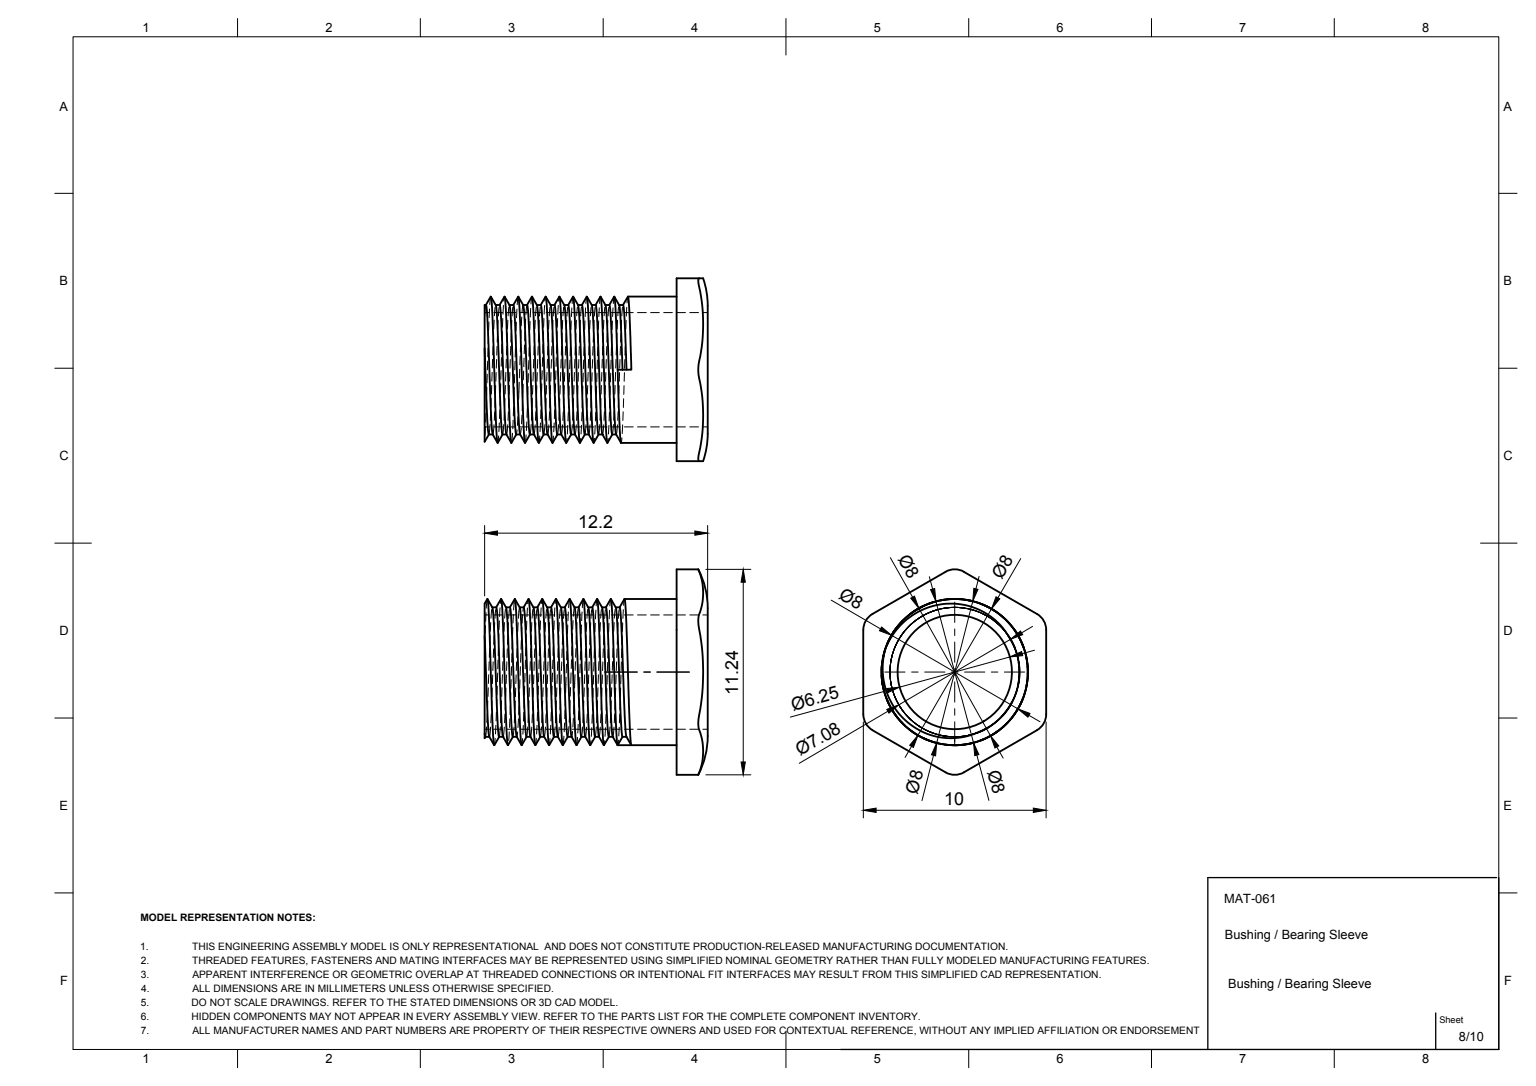
ISO-10303-21;
HEADER;
/* Generated by software containing ST-Developer
 * from STEP Tools, Inc. (www.steptools.com) 
 */

FILE_DESCRIPTION(
/* description */ ('', 'CAx-IF Rec.Pracs.---Representation and Presentation of Product Manufa
cturing Information (PMI)---4.0---2014-10-13'),
/* implementation_level */ '2;1');

FILE_NAME(
/* name */ 'Bushing _ Bearing Sleeve.step',
/* time_stamp */ '2026-10-28T14:45:12+01:00',
/* author */ (''),
/* organization */ (''),
/* preprocessor_version */ 'ST-DEVELOPER v20.2',
/* originating_system */ 'Autodesk Translation Framework v15.17.0.0',
/* authorisation */ '');

FILE_SCHEMA (('AP242_MANAGED_MODEL_BASED_3D_ENGINEERING_MIM_LF { 1 0 10303 442 2 1 4 }'));
ENDSEC;

DATA;
#10=MECHANICAL_DESIGN_GEOMETRIC_PRESENTATION_REPRESENTATION('',(#267),#52164);
#64=(
BOUNDED_CURVE()
B_SPLINE_CURVE(2,(#46348,#46349,#46350),.UNSPECIFIED.,.F.,.F.)
B_SPLINE_CURVE_WITH_KNOTS((3,3),(1.23956041519017,1.57079632679222),
 .UNSPECIFIED.)
CURVE()
GEOMETRIC_REPRESENTATION_ITEM()
RATIONAL_B_SPLINE_CURVE((0.987875274923375,0.980288238878012,1.))
REPRESENTATION_ITEM('')
);
#198=(
BOUNDED_SURFACE()
B_SPLINE_SURFACE(2,2,((#46210,#46211,#46212,#46213,#46214,#46215,#46216,
#46217,#46218),(#46219,#46220,#46221,#46222,#46223,#46224,#46225,#46226,
#46227),(#46228,#46229,#46230,#46231,#46232,#46233,#46234,#46235,#46236)),
 .UNSPECIFIED.,.F.,.T.,.F.)
B_SPLINE_SURFACE_WITH_KNOTS((3,3),(3,2,2,2,3),(-1.57079632679222,-1.09244241804695),
(-3.14159265358979,-1.5707963267949,0.,1.5707963267949,3.14159265358979),
 .UNSPECIFIED.)
GEOMETRIC_REPRESENTATION_ITEM()
RATIONAL_B_SPLINE_SURFACE(((1.,0.707106781186548,1.,0.707106781186548,1.,
0.707106781186548,1.,0.707106781186548,1.),(0.971533285943088,0.686977774638807,
0.971533285943088,0.686977774638807,0.971533285943088,0.686977774638807,
0.971533285943088,0.686977774638807,0.971533285943088),(1.,0.707106781186548,
1.,0.707106781186548,1.,0.707106781186548,1.,0.707106781186548,1.)))
REPRESENTATION_ITEM('')
SURFACE()
);
#241=SHAPE_REPRESENTATION_RELATIONSHIP('SRR','None',#52220,#254);
#254=ADVANCED_BREP_SHAPE_REPRESENTATION('',(#280),#52160);
#267=STYLED_ITEM('',(#52318),#280);
#280=MANIFOLD_SOLID_BREP('Body1',#9127);
#317=FACE_BOUND('',#1584,.T.);
#318=FACE_BOUND('',#1587,.T.);
#319=FACE_BOUND('',#1591,.T.);
#400=B_SPLINE_SURFACE_WITH_KNOTS('',3,3,((#46509,#46510,#46511,#46512,#46513,
#46514,#46515,#46516,#46517,#46518,#46519,#46520,#46521,#46522,#46523,#46524,
#46525,#46526,#46527,#46528,#46529,#46530,#46531,#46532,#46533,#46534,#46535,
#46536,#46537,#46538,#46539,#46540,#46541,#46542,#46543,#46544,#46545,#46546,
#46547,#46548,#46549,#46550,#46551,#46552,#46553,#46554,#46555,#46556,#46557,
#46558,#46559,#46560,#46561,#46562,#46563,#46564,#46565,#46566,#46567,#46568,
#46569,#46570,#46571,#46572,#46573,#46574,#46575),(#46576,#46577,#46578,
#46579,#46580,#46581,#46582,#46583,#46584,#46585,#46586,#46587,#46588,#46589,
#46590,#46591,#46592,#46593,#46594,#46595,#46596,#46597,#46598,#46599,#46600,
#46601,#46602,#46603,#46604,#46605,#46606,#46607,#46608,#46609,#46610,#46611,
#46612,#46613,#46614,#46615,#46616,#46617,#46618,#46619,#46620,#46621,#46622,
#46623,#46624,#46625,#46626,#46627,#46628,#46629,#46630,#46631,#46632,#46633,
#46634,#46635,#46636,#46637,#46638,#46639,#46640,#46641,#46642),(#46643,
#46644,#46645,#46646,#46647,#46648,#46649,#46650,#46651,#46652,#46653,#46654,
#46655,#46656,#46657,#46658,#46659,#46660,#46661,#46662,#46663,#46664,#46665,
#46666,#46667,#46668,#46669,#46670,#46671,#46672,#46673,#46674,#46675,#46676,
#46677,#46678,#46679,#46680,#46681,#46682,#46683,#46684,#46685,#46686,#46687,
#46688,#46689,#46690,#46691,#46692,#46693,#46694,#46695,#46696,#46697,#46698,
#46699,#46700,#46701,#46702,#46703,#46704,#46705,#46706,#46707,#46708,#46709),
(#46710,#46711,#46712,#46713,#46714,#46715,#46716,#46717,#46718,#46719,
#46720,#46721,#46722,#46723,#46724,#46725,#46726,#46727,#46728,#46729,#46730,
#46731,#46732,#46733,#46734,#46735,#46736,#46737,#46738,#46739,#46740,#46741,
#46742,#46743,#46744,#46745,#46746,#46747,#46748,#46749,#46750,#46751,#46752,
#46753,#46754,#46755,#46756,#46757,#46758,#46759,#46760,#46761,#46762,#46763,
#46764,#46765,#46766,#46767,#46768,#46769,#46770,#46771,#46772,#46773,#46774,
#46775,#46776)),.UNSPECIFIED.,.F.,.F.,.F.,(4,4),(4,1,1,1,1,1,1,1,1,1,1,
1,1,1,1,1,1,1,1,1,1,1,1,1,1,1,1,1,1,1,1,1,1,1,1,1,1,1,1,1,1,1,1,1,1,1,1,
1,1,1,1,1,1,1,1,1,1,1,1,1,1,1,1,1,4),(-0.04605142190376,1.046051421904),
(-0.02,-0.00375,0.0125,0.02875,0.045,0.06125,0.0775,0.09375,0.11,0.12625,
0.1425,0.15875,0.175,0.19125,0.2075,0.22375,0.24,0.25625,0.2725,0.28875,
0.305,0.32125,0.3375,0.35375,0.37,0.38625,0.4025,0.41875,0.435,0.45125,
0.4675,0.48375,0.5,0.51625,0.5325,0.54875,0.565,0.58125,0.5975,0.61375,
0.63,0.64625,0.6625,0.67875,0.695,0.71125,0.7275,0.74375,0.76,0.77625,0.7925,
0.80875,0.825,0.84125,0.8575,0.87375,0.89,0.90625,0.9225,0.93875,0.955,
0.97125,0.9875,1.00375,1.02),.UNSPECIFIED.);
#401=B_SPLINE_SURFACE_WITH_KNOTS('',3,3,((#47626,#47627,#47628,#47629,#47630,
#47631,#47632,#47633,#47634,#47635,#47636,#47637,#47638,#47639,#47640,#47641,
#47642,#47643,#47644,#47645,#47646,#47647,#47648,#47649,#47650,#47651,#47652,
#47653,#47654,#47655,#47656,#47657,#47658,#47659,#47660,#47661,#47662,#47663,
#47664,#47665,#47666,#47667,#47668,#47669,#47670,#47671,#47672,#47673,#47674,
#47675,#47676,#47677,#47678,#47679,#47680,#47681,#47682,#47683,#47684,#47685,
#47686,#47687,#47688,#47689,#47690,#47691,#47692),(#47693,#47694,#47695,
#47696,#47697,#47698,#47699,#47700,#47701,#47702,#47703,#47704,#47705,#47706,
#47707,#47708,#47709,#47710,#47711,#47712,#47713,#47714,#47715,#47716,#47717,
#47718,#47719,#47720,#47721,#47722,#47723,#47724,#47725,#47726,#47727,#47728,
#47729,#47730,#47731,#47732,#47733,#47734,#47735,#47736,#47737,#47738,#47739,
#47740,#47741,#47742,#47743,#47744,#47745,#47746,#47747,#47748,#47749,#47750,
#47751,#47752,#47753,#47754,#47755,#47756,#47757,#47758,#47759),(#47760,
#47761,#47762,#47763,#47764,#47765,#47766,#47767,#47768,#47769,#47770,#47771,
#47772,#47773,#47774,#47775,#47776,#47777,#47778,#47779,#47780,#47781,#47782,
#47783,#47784,#47785,#47786,#47787,#47788,#47789,#47790,#47791,#47792,#47793,
#47794,#47795,#47796,#47797,#47798,#47799,#47800,#47801,#47802,#47803,#47804,
#47805,#47806,#47807,#47808,#47809,#47810,#47811,#47812,#47813,#47814,#47815,
#47816,#47817,#47818,#47819,#47820,#47821,#47822,#47823,#47824,#47825,#47826),
(#47827,#47828,#47829,#47830,#47831,#47832,#47833,#47834,#47835,#47836,
#47837,#47838,#47839,#47840,#47841,#47842,#47843,#47844,#47845,#47846,#47847,
#47848,#47849,#47850,#47851,#47852,#47853,#47854,#47855,#47856,#47857,#47858,
#47859,#47860,#47861,#47862,#47863,#47864,#47865,#47866,#47867,#47868,#47869,
#47870,#47871,#47872,#47873,#47874,#47875,#47876,#47877,#47878,#47879,#47880,
#47881,#47882,#47883,#47884,#47885,#47886,#47887,#47888,#47889,#47890,#47891,
#47892,#47893)),.UNSPECIFIED.,.F.,.F.,.F.,(4,4),(4,1,1,1,1,1,1,1,1,1,1,
1,1,1,1,1,1,1,1,1,1,1,1,1,1,1,1,1,1,1,1,1,1,1,1,1,1,1,1,1,1,1,1,1,1,1,1,
1,1,1,1,1,1,1,1,1,1,1,1,1,1,1,1,1,4),(-0.04605142190375,1.046051421904),
(-0.02,-0.00375,0.0125,0.02875,0.045,0.06125,0.0775,0.09375,0.11,0.12625,
0.1425,0.15875,0.175,0.19125,0.2075,0.22375,0.24,0.25625,0.2725,0.28875,
0.305,0.32125,0.3375,0.35375,0.37,0.38625,0.4025,0.41875,0.435,0.45125,
0.4675,0.48375,0.5,0.51625,0.5325,0.54875,0.565,0.58125,0.5975,0.61375,
0.63,0.64625,0.6625,0.67875,0.695,0.71125,0.7275,0.74375,0.76,0.77625,0.7925,
0.80875,0.825,0.84125,0.8575,0.87375,0.89,0.90625,0.9225,0.93875,0.955,
0.97125,0.9875,1.00375,1.02),.UNSPECIFIED.);
#402=B_SPLINE_SURFACE_WITH_KNOTS('',3,3,((#48678,#48679,#48680,#48681,#48682,
#48683,#48684,#48685,#48686,#48687,#48688,#48689,#48690,#48691,#48692,#48693,
#48694,#48695,#48696,#48697,#48698,#48699,#48700,#48701,#48702,#48703,#48704,
#48705,#48706,#48707,#48708,#48709,#48710,#48711,#48712,#48713,#48714,#48715,
#48716,#48717,#48718,#48719,#48720,#48721,#48722,#48723,#48724,#48725,#48726,
#48727,#48728,#48729,#48730,#48731,#48732,#48733,#48734,#48735,#48736,#48737,
#48738,#48739,#48740,#48741,#48742,#48743,#48744),(#48745,#48746,#48747,
#48748,#48749,#48750,#48751,#48752,#48753,#48754,#48755,#48756,#48757,#48758,
#48759,#48760,#48761,#48762,#48763,#48764,#48765,#48766,#48767,#48768,#48769,
#48770,#48771,#48772,#48773,#48774,#48775,#48776,#48777,#48778,#48779,#48780,
#48781,#48782,#48783,#48784,#48785,#48786,#48787,#48788,#48789,#48790,#48791,
#48792,#48793,#48794,#48795,#48796,#48797,#48798,#48799,#48800,#48801,#48802,
#48803,#48804,#48805,#48806,#48807,#48808,#48809,#48810,#48811),(#48812,
#48813,#48814,#48815,#48816,#48817,#48818,#48819,#48820,#48821,#48822,#48823,
#48824,#48825,#48826,#48827,#48828,#48829,#48830,#48831,#48832,#48833,#48834,
#48835,#48836,#48837,#48838,#48839,#48840,#48841,#48842,#48843,#48844,#48845,
#48846,#48847,#48848,#48849,#48850,#48851,#48852,#48853,#48854,#48855,#48856,
#48857,#48858,#48859,#48860,#48861,#48862,#48863,#48864,#48865,#48866,#48867,
#48868,#48869,#48870,#48871,#48872,#48873,#48874,#48875,#48876,#48877,#48878),
(#48879,#48880,#48881,#48882,#48883,#48884,#48885,#48886,#48887,#48888,
#48889,#48890,#48891,#48892,#48893,#48894,#48895,#48896,#48897,#48898,#48899,
#48900,#48901,#48902,#48903,#48904,#48905,#48906,#48907,#48908,#48909,#48910,
#48911,#48912,#48913,#48914,#48915,#48916,#48917,#48918,#48919,#48920,#48921,
#48922,#48923,#48924,#48925,#48926,#48927,#48928,#48929,#48930,#48931,#48932,
#48933,#48934,#48935,#48936,#48937,#48938,#48939,#48940,#48941,#48942,#48943,
#48944,#48945)),.UNSPECIFIED.,.F.,.F.,.F.,(4,4),(4,1,1,1,1,1,1,1,1,1,1,
1,1,1,1,1,1,1,1,1,1,1,1,1,1,1,1,1,1,1,1,1,1,1,1,1,1,1,1,1,1,1,1,1,1,1,1,
1,1,1,1,1,1,1,1,1,1,1,1,1,1,1,1,1,4),(-0.04605142190375,1.046051421904),
(-0.02,-0.00375,0.0125,0.02875,0.045,0.06125,0.0775,0.09375,0.11,0.12625,
0.1425,0.15875,0.175,0.19125,0.2075,0.22375,0.24,0.25625,0.2725,0.28875,
0.305,0.32125,0.3375,0.35375,0.37,0.38625,0.4025,0.41875,0.435,0.45125,
0.4675,0.48375,0.5,0.51625,0.5325,0.54875,0.565,0.58125,0.5975,0.61375,
0.63,0.64625,0.6625,0.67875,0.695,0.71125,0.7275,0.74375,0.76,0.77625,0.7925,
0.80875,0.825,0.84125,0.8575,0.87375,0.89,0.90625,0.9225,0.93875,0.955,
0.97125,0.9875,1.00375,1.02),.UNSPECIFIED.);
#403=B_SPLINE_SURFACE_WITH_KNOTS('',3,3,((#49626,#49627,#49628,#49629,#49630,
#49631,#49632,#49633,#49634,#49635,#49636,#49637,#49638,#49639,#49640,#49641,
#49642,#49643,#49644,#49645,#49646,#49647,#49648,#49649,#49650,#49651,#49652,
#49653,#49654,#49655,#49656,#49657,#49658,#49659,#49660,#49661,#49662,#49663,
#49664,#49665,#49666,#49667,#49668,#49669,#49670,#49671,#49672,#49673,#49674,
#49675,#49676,#49677,#49678,#49679,#49680,#49681,#49682,#49683,#49684,#49685,
#49686,#49687,#49688,#49689,#49690,#49691,#49692),(#49693,#49694,#49695,
#49696,#49697,#49698,#49699,#49700,#49701,#49702,#49703,#49704,#49705,#49706,
#49707,#49708,#49709,#49710,#49711,#49712,#49713,#49714,#49715,#49716,#49717,
#49718,#49719,#49720,#49721,#49722,#49723,#49724,#49725,#49726,#49727,#49728,
#49729,#49730,#49731,#49732,#49733,#49734,#49735,#49736,#49737,#49738,#49739,
#49740,#49741,#49742,#49743,#49744,#49745,#49746,#49747,#49748,#49749,#49750,
#49751,#49752,#49753,#49754,#49755,#49756,#49757,#49758,#49759),(#49760,
#49761,#49762,#49763,#49764,#49765,#49766,#49767,#49768,#49769,#49770,#49771,
#49772,#49773,#49774,#49775,#49776,#49777,#49778,#49779,#49780,#49781,#49782,
#49783,#49784,#49785,#49786,#49787,#49788,#49789,#49790,#49791,#49792,#49793,
#49794,#49795,#49796,#49797,#49798,#49799,#49800,#49801,#49802,#49803,#49804,
#49805,#49806,#49807,#49808,#49809,#49810,#49811,#49812,#49813,#49814,#49815,
#49816,#49817,#49818,#49819,#49820,#49821,#49822,#49823,#49824,#49825,#49826),
(#49827,#49828,#49829,#49830,#49831,#49832,#49833,#49834,#49835,#49836,
#49837,#49838,#49839,#49840,#49841,#49842,#49843,#49844,#49845,#49846,#49847,
#49848,#49849,#49850,#49851,#49852,#49853,#49854,#49855,#49856,#49857,#49858,
#49859,#49860,#49861,#49862,#49863,#49864,#49865,#49866,#49867,#49868,#49869,
#49870,#49871,#49872,#49873,#49874,#49875,#49876,#49877,#49878,#49879,#49880,
#49881,#49882,#49883,#49884,#49885,#49886,#49887,#49888,#49889,#49890,#49891,
#49892,#49893)),.UNSPECIFIED.,.F.,.F.,.F.,(4,4),(4,1,1,1,1,1,1,1,1,1,1,
1,1,1,1,1,1,1,1,1,1,1,1,1,1,1,1,1,1,1,1,1,1,1,1,1,1,1,1,1,1,1,1,1,1,1,1,
1,1,1,1,1,1,1,1,1,1,1,1,1,1,1,1,1,4),(-0.04605142190375,1.046051421904),
(0.151,0.1645257352941,0.1780514705882,0.1915772058824,0.2051029411765,
0.2186286764706,0.2321544117647,0.2456801470588,0.2592058823529,0.2727316176471,
0.2862573529412,0.2997830882353,0.3133088235294,0.3268345588235,0.3403602941176,
0.3538860294118,0.3674117647059,0.3809375,0.3944632352941,0.4079889705882,
0.4215147058824,0.4350404411765,0.4485661764706,0.4620919117647,0.4756176470588,
0.4891433823529,0.5026691176471,0.5161948529412,0.5297205882353,0.5432463235294,
0.5567720588235,0.5702977941176,0.5838235294118,0.5973492647059,0.610875,
0.6244007352941,0.6379264705882,0.6514522058824,0.6649779411765,0.6785036764706,
0.6920294117647,0.7055551470588,0.7190808823529,0.7326066176471,0.7461323529412,
0.7596580882353,0.7731838235294,0.7867095588235,0.8002352941176,0.8137610294118,
0.8272867647059,0.8408125,0.8543382352941,0.8678639705882,0.8813897058824,
0.8949154411765,0.9084411764706,0.9219669117647,0.9354926470588,0.9490183823529,
0.9625441176471,0.9760698529412,0.9895955882353,1.003121323529,1.016647058824),
 .UNSPECIFIED.);
#404=B_SPLINE_SURFACE_WITH_KNOTS('',3,3,((#50188,#50189,#50190,#50191,#50192,
#50193,#50194,#50195,#50196,#50197,#50198,#50199,#50200,#50201,#50202,#50203,
#50204,#50205,#50206,#50207,#50208,#50209,#50210,#50211,#50212,#50213,#50214,
#50215,#50216,#50217,#50218,#50219,#50220,#50221,#50222),(#50223,#50224,
#50225,#50226,#50227,#50228,#50229,#50230,#50231,#50232,#50233,#50234,#50235,
#50236,#50237,#50238,#50239,#50240,#50241,#50242,#50243,#50244,#50245,#50246,
#50247,#50248,#50249,#50250,#50251,#50252,#50253,#50254,#50255,#50256,#50257),
(#50258,#50259,#50260,#50261,#50262,#50263,#50264,#50265,#50266,#50267,
#50268,#50269,#50270,#50271,#50272,#50273,#50274,#50275,#50276,#50277,#50278,
#50279,#50280,#50281,#50282,#50283,#50284,#50285,#50286,#50287,#50288,#50289,
#50290,#50291,#50292),(#50293,#50294,#50295,#50296,#50297,#50298,#50299,
#50300,#50301,#50302,#50303,#50304,#50305,#50306,#50307,#50308,#50309,#50310,
#50311,#50312,#50313,#50314,#50315,#50316,#50317,#50318,#50319,#50320,#50321,
#50322,#50323,#50324,#50325,#50326,#50327)),.UNSPECIFIED.,.F.,.F.,.F.,(4,
4),(4,1,1,1,1,1,1,1,1,1,1,1,1,1,1,1,1,1,1,1,1,1,1,1,1,1,1,1,1,1,1,1,4),
(-0.04605142190375,1.046051421904),(0.3253907954222,0.3468856965485,0.3683805976747,
0.389875498801,0.4113703999272,0.4328653010535,0.4543602021797,0.475855103306,
0.4973500044322,0.5188449055585,0.5403398066847,0.561834707811,0.5833296089372,
0.6048245100635,0.6263194111897,0.647814312316,0.6693092134423,0.6908041145685,
0.7122990156948,0.733793916821,0.7552888179473,0.7767837190735,0.7982786201998,
0.819773521326,0.8412684224523,0.8627633235785,0.8842582247048,0.905753125831,
0.9272480269573,0.9487429280835,0.9702378292098,0.9917327303361,1.013227631462),
 .UNSPECIFIED.);
#405=B_SPLINE_SURFACE_WITH_KNOTS('',3,3,((#50500,#50501,#50502,#50503,#50504,
#50505,#50506,#50507,#50508,#50509,#50510,#50511,#50512,#50513,#50514,#50515,
#50516,#50517,#50518,#50519,#50520,#50521,#50522,#50523,#50524,#50525,#50526,
#50527,#50528,#50529,#50530,#50531,#50532,#50533,#50534),(#50535,#50536,
#50537,#50538,#50539,#50540,#50541,#50542,#50543,#50544,#50545,#50546,#50547,
#50548,#50549,#50550,#50551,#50552,#50553,#50554,#50555,#50556,#50557,#50558,
#50559,#50560,#50561,#50562,#50563,#50564,#50565,#50566,#50567,#50568,#50569),
(#50570,#50571,#50572,#50573,#50574,#50575,#50576,#50577,#50578,#50579,
#50580,#50581,#50582,#50583,#50584,#50585,#50586,#50587,#50588,#50589,#50590,
#50591,#50592,#50593,#50594,#50595,#50596,#50597,#50598,#50599,#50600,#50601,
#50602,#50603,#50604),(#50605,#50606,#50607,#50608,#50609,#50610,#50611,
#50612,#50613,#50614,#50615,#50616,#50617,#50618,#50619,#50620,#50621,#50622,
#50623,#50624,#50625,#50626,#50627,#50628,#50629,#50630,#50631,#50632,#50633,
#50634,#50635,#50636,#50637,#50638,#50639)),.UNSPECIFIED.,.F.,.F.,.F.,(4,
4),(4,1,1,1,1,1,1,1,1,1,1,1,1,1,1,1,1,1,1,1,1,1,1,1,1,1,1,1,1,1,1,1,4),
(-0.1117758545036,1.111775854504),(0.2466092045778,0.2706143034515,0.2946194023253,
0.318624501199,0.3426296000728,0.3666346989465,0.3906397978203,0.414644896694,
0.4386499955678,0.4626550944415,0.4866601933153,0.510665292189,0.5346703910628,
0.5586754899365,0.5826805888103,0.606685687684,0.6306907865577,0.6546958854315,
0.6787009843052,0.702706083179,0.7267111820527,0.7507162809265,0.7747213798002,
0.798726478674,0.8227315775477,0.8467366764215,0.8707417752952,0.894746874169,
0.9187519730427,0.9427570719165,0.9667621707902,0.9907672696639,1.014772368538),
 .UNSPECIFIED.);
#406=B_SPLINE_SURFACE_WITH_KNOTS('',3,3,((#50641,#50642,#50643,#50644,#50645,
#50646,#50647,#50648,#50649,#50650,#50651,#50652,#50653,#50654,#50655,#50656,
#50657,#50658,#50659,#50660,#50661,#50662,#50663,#50664,#50665,#50666,#50667,
#50668,#50669,#50670,#50671,#50672,#50673,#50674,#50675,#50676,#50677,#50678,
#50679,#50680,#50681,#50682,#50683,#50684,#50685,#50686,#50687,#50688,#50689,
#50690,#50691,#50692,#50693,#50694,#50695,#50696,#50697,#50698,#50699,#50700,
#50701,#50702,#50703,#50704,#50705,#50706,#50707),(#50708,#50709,#50710,
#50711,#50712,#50713,#50714,#50715,#50716,#50717,#50718,#50719,#50720,#50721,
#50722,#50723,#50724,#50725,#50726,#50727,#50728,#50729,#50730,#50731,#50732,
#50733,#50734,#50735,#50736,#50737,#50738,#50739,#50740,#50741,#50742,#50743,
#50744,#50745,#50746,#50747,#50748,#50749,#50750,#50751,#50752,#50753,#50754,
#50755,#50756,#50757,#50758,#50759,#50760,#50761,#50762,#50763,#50764,#50765,
#50766,#50767,#50768,#50769,#50770,#50771,#50772,#50773,#50774),(#50775,
#50776,#50777,#50778,#50779,#50780,#50781,#50782,#50783,#50784,#50785,#50786,
#50787,#50788,#50789,#50790,#50791,#50792,#50793,#50794,#50795,#50796,#50797,
#50798,#50799,#50800,#50801,#50802,#50803,#50804,#50805,#50806,#50807,#50808,
#50809,#50810,#50811,#50812,#50813,#50814,#50815,#50816,#50817,#50818,#50819,
#50820,#50821,#50822,#50823,#50824,#50825,#50826,#50827,#50828,#50829,#50830,
#50831,#50832,#50833,#50834,#50835,#50836,#50837,#50838,#50839,#50840,#50841),
(#50842,#50843,#50844,#50845,#50846,#50847,#50848,#50849,#50850,#50851,
#50852,#50853,#50854,#50855,#50856,#50857,#50858,#50859,#50860,#50861,#50862,
#50863,#50864,#50865,#50866,#50867,#50868,#50869,#50870,#50871,#50872,#50873,
#50874,#50875,#50876,#50877,#50878,#50879,#50880,#50881,#50882,#50883,#50884,
#50885,#50886,#50887,#50888,#50889,#50890,#50891,#50892,#50893,#50894,#50895,
#50896,#50897,#50898,#50899,#50900,#50901,#50902,#50903,#50904,#50905,#50906,
#50907,#50908)),.UNSPECIFIED.,.F.,.F.,.F.,(4,4),(4,1,1,1,1,1,1,1,1,1,1,
1,1,1,1,1,1,1,1,1,1,1,1,1,1,1,1,1,1,1,1,1,1,1,1,1,1,1,1,1,1,1,1,1,1,1,1,
1,1,1,1,1,1,1,1,1,1,1,1,1,1,1,1,1,4),(-0.1117758545036,1.111775854504),
(-0.02,-0.00375,0.0125,0.02875,0.045,0.06125,0.0775,0.09375,0.11,0.12625,
0.1425,0.15875,0.175,0.19125,0.2075,0.22375,0.24,0.25625,0.2725,0.28875,
0.305,0.32125,0.3375,0.35375,0.37,0.38625,0.4025,0.41875,0.435,0.45125,
0.4675,0.48375,0.5,0.51625,0.5325,0.54875,0.565,0.58125,0.5975,0.61375,
0.63,0.64625,0.6625,0.67875,0.695,0.71125,0.7275,0.74375,0.76,0.77625,0.7925,
0.80875,0.825,0.84125,0.8575,0.87375,0.89,0.90625,0.9225,0.93875,0.955,
0.97125,0.9875,1.00375,1.02),.UNSPECIFIED.);
#407=B_SPLINE_SURFACE_WITH_KNOTS('',3,3,((#50910,#50911,#50912,#50913,#50914,
#50915,#50916,#50917,#50918,#50919,#50920,#50921,#50922,#50923,#50924,#50925,
#50926,#50927,#50928,#50929,#50930,#50931,#50932,#50933,#50934,#50935,#50936,
#50937,#50938,#50939,#50940,#50941,#50942,#50943,#50944,#50945,#50946,#50947,
#50948,#50949,#50950,#50951,#50952,#50953,#50954,#50955,#50956,#50957,#50958,
#50959,#50960,#50961,#50962,#50963,#50964,#50965,#50966,#50967,#50968,#50969,
#50970,#50971,#50972,#50973,#50974,#50975,#50976),(#50977,#50978,#50979,
#50980,#50981,#50982,#50983,#50984,#50985,#50986,#50987,#50988,#50989,#50990,
#50991,#50992,#50993,#50994,#50995,#50996,#50997,#50998,#50999,#51000,#51001,
#51002,#51003,#51004,#51005,#51006,#51007,#51008,#51009,#51010,#51011,#51012,
#51013,#51014,#51015,#51016,#51017,#51018,#51019,#51020,#51021,#51022,#51023,
#51024,#51025,#51026,#51027,#51028,#51029,#51030,#51031,#51032,#51033,#51034,
#51035,#51036,#51037,#51038,#51039,#51040,#51041,#51042,#51043),(#51044,
#51045,#51046,#51047,#51048,#51049,#51050,#51051,#51052,#51053,#51054,#51055,
#51056,#51057,#51058,#51059,#51060,#51061,#51062,#51063,#51064,#51065,#51066,
#51067,#51068,#51069,#51070,#51071,#51072,#51073,#51074,#51075,#51076,#51077,
#51078,#51079,#51080,#51081,#51082,#51083,#51084,#51085,#51086,#51087,#51088,
#51089,#51090,#51091,#51092,#51093,#51094,#51095,#51096,#51097,#51098,#51099,
#51100,#51101,#51102,#51103,#51104,#51105,#51106,#51107,#51108,#51109,#51110),
(#51111,#51112,#51113,#51114,#51115,#51116,#51117,#51118,#51119,#51120,
#51121,#51122,#51123,#51124,#51125,#51126,#51127,#51128,#51129,#51130,#51131,
#51132,#51133,#51134,#51135,#51136,#51137,#51138,#51139,#51140,#51141,#51142,
#51143,#51144,#51145,#51146,#51147,#51148,#51149,#51150,#51151,#51152,#51153,
#51154,#51155,#51156,#51157,#51158,#51159,#51160,#51161,#51162,#51163,#51164,
#51165,#51166,#51167,#51168,#51169,#51170,#51171,#51172,#51173,#51174,#51175,
#51176,#51177)),.UNSPECIFIED.,.F.,.F.,.F.,(4,4),(4,1,1,1,1,1,1,1,1,1,1,
1,1,1,1,1,1,1,1,1,1,1,1,1,1,1,1,1,1,1,1,1,1,1,1,1,1,1,1,1,1,1,1,1,1,1,1,
1,1,1,1,1,1,1,1,1,1,1,1,1,1,1,1,1,4),(-0.1117758545037,1.111775854504),
(-0.02,-0.00375,0.0125,0.02875,0.045,0.06125,0.0775,0.09375,0.11,0.12625,
0.1425,0.15875,0.175,0.19125,0.2075,0.22375,0.24,0.25625,0.2725,0.28875,
0.305,0.32125,0.3375,0.35375,0.37,0.38625,0.4025,0.41875,0.435,0.45125,
0.4675,0.48375,0.5,0.51625,0.5325,0.54875,0.565,0.58125,0.5975,0.61375,
0.63,0.64625,0.6625,0.67875,0.695,0.71125,0.7275,0.74375,0.76,0.77625,0.7925,
0.80875,0.825,0.84125,0.8575,0.87375,0.89,0.90625,0.9225,0.93875,0.955,
0.97125,0.9875,1.00375,1.02),.UNSPECIFIED.);
#408=B_SPLINE_SURFACE_WITH_KNOTS('',3,3,((#51791,#51792,#51793,#51794,#51795,
#51796,#51797,#51798,#51799,#51800,#51801,#51802,#51803,#51804,#51805,#51806,
#51807,#51808,#51809,#51810,#51811,#51812,#51813,#51814,#51815,#51816,#51817,
#51818,#51819,#51820,#51821,#51822,#51823,#51824,#51825,#51826,#51827,#51828,
#51829,#51830,#51831,#51832,#51833,#51834,#51835,#51836,#51837,#51838,#51839,
#51840,#51841,#51842,#51843,#51844,#51845,#51846,#51847,#51848,#51849,#51850,
#51851,#51852,#51853,#51854,#51855,#51856,#51857),(#51858,#51859,#51860,
#51861,#51862,#51863,#51864,#51865,#51866,#51867,#51868,#51869,#51870,#51871,
#51872,#51873,#51874,#51875,#51876,#51877,#51878,#51879,#51880,#51881,#51882,
#51883,#51884,#51885,#51886,#51887,#51888,#51889,#51890,#51891,#51892,#51893,
#51894,#51895,#51896,#51897,#51898,#51899,#51900,#51901,#51902,#51903,#51904,
#51905,#51906,#51907,#51908,#51909,#51910,#51911,#51912,#51913,#51914,#51915,
#51916,#51917,#51918,#51919,#51920,#51921,#51922,#51923,#51924),(#51925,
#51926,#51927,#51928,#51929,#51930,#51931,#51932,#51933,#51934,#51935,#51936,
#51937,#51938,#51939,#51940,#51941,#51942,#51943,#51944,#51945,#51946,#51947,
#51948,#51949,#51950,#51951,#51952,#51953,#51954,#51955,#51956,#51957,#51958,
#51959,#51960,#51961,#51962,#51963,#51964,#51965,#51966,#51967,#51968,#51969,
#51970,#51971,#51972,#51973,#51974,#51975,#51976,#51977,#51978,#51979,#51980,
#51981,#51982,#51983,#51984,#51985,#51986,#51987,#51988,#51989,#51990,#51991),
(#51992,#51993,#51994,#51995,#51996,#51997,#51998,#51999,#52000,#52001,
#52002,#52003,#52004,#52005,#52006,#52007,#52008,#52009,#52010,#52011,#52012,
#52013,#52014,#52015,#52016,#52017,#52018,#52019,#52020,#52021,#52022,#52023,
#52024,#52025,#52026,#52027,#52028,#52029,#52030,#52031,#52032,#52033,#52034,
#52035,#52036,#52037,#52038,#52039,#52040,#52041,#52042,#52043,#52044,#52045,
#52046,#52047,#52048,#52049,#52050,#52051,#52052,#52053,#52054,#52055,#52056,
#52057,#52058)),.UNSPECIFIED.,.F.,.F.,.F.,(4,4),(4,1,1,1,1,1,1,1,1,1,1,
1,1,1,1,1,1,1,1,1,1,1,1,1,1,1,1,1,1,1,1,1,1,1,1,1,1,1,1,1,1,1,1,1,1,1,1,
1,1,1,1,1,1,1,1,1,1,1,1,1,1,1,1,1,4),(-0.04605142190376,1.046051421904),
(-0.02,-0.00375,0.0125,0.02875,0.045,0.06125,0.0775,0.09375,0.11,0.12625,
0.1425,0.15875,0.175,0.19125,0.2075,0.22375,0.24,0.25625,0.2725,0.28875,
0.305,0.32125,0.3375,0.35375,0.37,0.38625,0.4025,0.41875,0.435,0.45125,
0.4675,0.48375,0.5,0.51625,0.5325,0.54875,0.565,0.58125,0.5975,0.61375,
0.63,0.64625,0.6625,0.67875,0.695,0.71125,0.7275,0.74375,0.76,0.77625,0.7925,
0.80875,0.825,0.84125,0.8575,0.87375,0.89,0.90625,0.9225,0.93875,0.955,
0.97125,0.9875,1.00375,1.02),.UNSPECIFIED.);
#505=PLANE('',#10143);
#506=PLANE('',#10147);
#507=PLANE('',#10151);
#508=PLANE('',#10159);
#509=PLANE('',#10160);
#510=PLANE('',#10162);
#511=PLANE('',#10164);
#512=PLANE('',#10166);
#513=PLANE('',#10168);
#514=PLANE('',#10170);
#1017=FACE_OUTER_BOUND('',#1583,.T.);
#1018=FACE_OUTER_BOUND('',#1585,.T.);
#1019=FACE_OUTER_BOUND('',#1586,.T.);
#1020=FACE_OUTER_BOUND('',#1588,.T.);
#1021=FACE_OUTER_BOUND('',#1589,.T.);
#1022=FACE_OUTER_BOUND('',#1590,.T.);
#1023=FACE_OUTER_BOUND('',#1592,.T.);
#1024=FACE_OUTER_BOUND('',#1593,.T.);
#1025=FACE_OUTER_BOUND('',#1594,.T.);
#1026=FACE_OUTER_BOUND('',#1595,.T.);
#1027=FACE_OUTER_BOUND('',#1596,.T.);
#1028=FACE_OUTER_BOUND('',#1597,.T.);
#1029=FACE_OUTER_BOUND('',#1598,.T.);
#1030=FACE_OUTER_BOUND('',#1599,.T.);
#1031=FACE_OUTER_BOUND('',#1600,.T.);
#1032=FACE_OUTER_BOUND('',#1601,.T.);
#1033=FACE_OUTER_BOUND('',#1602,.T.);
#1034=FACE_OUTER_BOUND('',#1603,.T.);
#1035=FACE_OUTER_BOUND('',#1604,.T.);
#1036=FACE_OUTER_BOUND('',#1605,.T.);
#1037=FACE_OUTER_BOUND('',#1606,.T.);
#1038=FACE_OUTER_BOUND('',#1607,.T.);
#1039=FACE_OUTER_BOUND('',#1608,.T.);
#1040=FACE_OUTER_BOUND('',#1609,.T.);
#1041=FACE_OUTER_BOUND('',#1610,.T.);
#1042=FACE_OUTER_BOUND('',#1611,.T.);
#1043=FACE_OUTER_BOUND('',#1612,.T.);
#1044=FACE_OUTER_BOUND('',#1613,.T.);
#1583=EDGE_LOOP('',(#8170,#8171,#8172,#8173,#8174));
#1584=EDGE_LOOP('',(#8175));
#1585=EDGE_LOOP('',(#8176,#8177,#8178,#8179));
#1586=EDGE_LOOP('',(#8180));
#1587=EDGE_LOOP('',(#8181));
#1588=EDGE_LOOP('',(#8182,#8183,#8184,#8185,#8186,#8187,#8188,#8189,#8190,
#8191,#8192,#8193,#8194,#8195,#8196,#8197));
#1589=EDGE_LOOP('',(#8198,#8199,#8200,#8201));
#1590=EDGE_LOOP('',(#8202,#8203,#8204,#8205,#8206,#8207,#8208,#8209,#8210,
#8211,#8212,#8213));
#1591=EDGE_LOOP('',(#8214));
#1592=EDGE_LOOP('',(#8215,#8216,#8217,#8218,#8219,#8220));
#1593=EDGE_LOOP('',(#8221,#8222,#8223,#8224));
#1594=EDGE_LOOP('',(#8225,#8226,#8227,#8228,#8229));
#1595=EDGE_LOOP('',(#8230,#8231,#8232,#8233,#8234));
#1596=EDGE_LOOP('',(#8235,#8236,#8237,#8238,#8239));
#1597=EDGE_LOOP('',(#8240,#8241,#8242,#8243,#8244,#8245));
#1598=EDGE_LOOP('',(#8246,#8247,#8248,#8249));
#1599=EDGE_LOOP('',(#8250,#8251,#8252,#8253,#8254));
#1600=EDGE_LOOP('',(#8255,#8256,#8257,#8258));
#1601=EDGE_LOOP('',(#8259,#8260,#8261,#8262));
#1602=EDGE_LOOP('',(#8263,#8264,#8265,#8266,#8267,#8268));
#1603=EDGE_LOOP('',(#8269,#8270,#8271,#8272));
#1604=EDGE_LOOP('',(#8273,#8274,#8275,#8276));
#1605=EDGE_LOOP('',(#8277,#8278,#8279,#8280));
#1606=EDGE_LOOP('',(#8281,#8282,#8283,#8284));
#1607=EDGE_LOOP('',(#8285,#8286,#8287,#8288));
#1608=EDGE_LOOP('',(#8289,#8290,#8291,#8292));
#1609=EDGE_LOOP('',(#8293,#8294,#8295,#8296));
#1610=EDGE_LOOP('',(#8297,#8298,#8299,#8300));
#1611=EDGE_LOOP('',(#8301,#8302,#8303,#8304,#8305));
#1612=EDGE_LOOP('',(#8306,#8307,#8308,#8309));
#1613=EDGE_LOOP('',(#8310,#8311,#8312,#8313));
#2071=CIRCLE('',#10144,3.125);
#2072=CIRCLE('',#10146,3.125);
#2073=CIRCLE('',#10148,3.5);
#2074=CIRCLE('',#10150,1.);
#2075=CIRCLE('',#10152,1.);
#2076=CIRCLE('',#10153,1.);
#2077=CIRCLE('',#10154,1.);
#2078=CIRCLE('',#10155,1.);
#2079=CIRCLE('',#10156,1.);
#2080=CIRCLE('',#10157,4.);
#2428=B_SPLINE_CURVE_WITH_KNOTS('',3,(#46066,#46067,#46068,#46069),
 .UNSPECIFIED.,.F.,.F.,(4,4),(-0.000287379327346715,0.),.UNSPECIFIED.);
#2429=B_SPLINE_CURVE_WITH_KNOTS('',3,(#46071,#46072,#46073,#46074,#46075,
#46076,#46077,#46078,#46079,#46080,#46081,#46082,#46083,#46084,#46085,#46086,
#46087,#46088,#46089,#46090,#46091,#46092,#46093,#46094,#46095,#46096,#46097,
#46098,#46099,#46100,#46101,#46102,#46103,#46104,#46105,#46106,#46107,#46108,
#46109,#46110,#46111,#46112,#46113,#46114,#46115,#46116,#46117,#46118,#46119,
#46120,#46121,#46122,#46123,#46124,#46125,#46126,#46127,#46128,#46129,#46130,
#46131,#46132,#46133,#46134,#46135,#46136,#46137,#46138,#46139,#46140,#46141,
#46142,#46143,#46144,#46145,#46146,#46147,#46148,#46149,#46150,#46151,#46152,
#46153,#46154,#46155,#46156,#46157,#46158,#46159,#46160,#46161,#46162,#46163,
#46164),.UNSPECIFIED.,.F.,.F.,(4,3,3,3,3,3,3,3,3,3,3,3,3,3,3,3,3,3,3,3,
3,3,3,3,3,3,3,3,3,3,3,4),(0.,0.0334880516165954,0.0622449481709034,0.0833304545710313,
0.123139222900696,0.158240223188287,0.176189139696093,0.217007009430374,
0.243869787273509,0.26354322405106,0.302458774449498,0.33355876922255,0.374434885871789,
0.405321381393714,0.426172721464637,0.480843228725633,0.507476669962832,
0.544616299200151,0.574867627238567,0.592227140301538,0.637891373171595,
0.668397489031486,0.7156914768719,0.744145082796372,0.770511427895059,0.813365315244751,
0.836703116619631,0.881940300050722,0.91091246542526,0.927753817005376,
0.962791389277124,0.997828961548873),.UNSPECIFIED.);
#2430=B_SPLINE_CURVE_WITH_KNOTS('',3,(#46166,#46167,#46168,#46169),
 .UNSPECIFIED.,.F.,.F.,(4,4),(-0.00107348259049816,0.),.UNSPECIFIED.);
#2431=B_SPLINE_CURVE_WITH_KNOTS('',3,(#46171,#46172,#46173,#46174,#46175,
#46176,#46177,#46178,#46179,#46180,#46181,#46182,#46183,#46184),
 .UNSPECIFIED.,.F.,.F.,(4,2,2,2,2,2,4),(-0.747237513889951,-0.627110670602595,
-0.492162734458781,-0.361378717436516,-0.240449917906045,-0.127292557609884,
-2.3301729044132E-6),.UNSPECIFIED.);
#2432=B_SPLINE_CURVE_WITH_KNOTS('',3,(#46185,#46186,#46187,#46188,#46189,
#46190,#46191,#46192,#46193,#46194,#46195,#46196,#46197,#46198,#46199,#46200),
 .UNSPECIFIED.,.F.,.F.,(4,2,2,2,2,2,2,4),(-0.557266864962719,-0.476580853062999,
-0.396866002960756,-0.315372123091983,-0.242726490281515,-0.148650466132605,
-0.073950688870771,-0.000468069961644113),.UNSPECIFIED.);
#2433=B_SPLINE_CURVE_WITH_KNOTS('',3,(#46239,#46240,#46241,#46242,#46243,
#46244,#46245,#46246,#46247,#46248),.UNSPECIFIED.,.F.,.F.,(4,2,2,2,4),(-0.373790461969616,
-0.353425955511238,-0.32400441351636,-0.295535379633958,-0.267904010196117),
 .UNSPECIFIED.);
#2434=B_SPLINE_CURVE_WITH_KNOTS('',3,(#46250,#46251,#46252,#46253,#46254,
#46255,#46256,#46257,#46258,#46259,#46260),.UNSPECIFIED.,.F.,.F.,(4,2,3,
2,4),(-0.218968937117933,-0.202250368267603,0.,0.202250368267602,0.21896893711841),
 .UNSPECIFIED.);
#2435=B_SPLINE_CURVE_WITH_KNOTS('',3,(#46262,#46263,#46264,#46265,#46266,
#46267,#46268,#46269,#46270,#46271),.UNSPECIFIED.,.F.,.F.,(4,2,2,2,4),(0.267904010196053,
0.295535379633939,0.324004413516362,0.353425955511275,0.37379046196938),
 .UNSPECIFIED.);
#2436=B_SPLINE_CURVE_WITH_KNOTS('',3,(#46273,#46274,#46275,#46276,#46277,
#46278,#46279,#46280,#46281,#46282,#46283),.UNSPECIFIED.,.F.,.F.,(4,2,3,
2,4),(-0.218968937118539,-0.202250368267599,0.,0.202250368267599,0.218968937117935),
 .UNSPECIFIED.);
#2437=B_SPLINE_CURVE_WITH_KNOTS('',3,(#46285,#46286,#46287,#46288,#46289,
#46290,#46291,#46292,#46293,#46294),.UNSPECIFIED.,.F.,.F.,(4,2,2,2,4),(0.26790401019593,
0.295535379633943,0.324004413516341,0.353425955511207,0.373790461969294),
 .UNSPECIFIED.);
#2438=B_SPLINE_CURVE_WITH_KNOTS('',3,(#46296,#46297,#46298,#46299,#46300,
#46301,#46302,#46303,#46304,#46305,#46306),.UNSPECIFIED.,.F.,.F.,(4,2,3,
2,4),(-0.218968937118688,-0.20225036826751,0.,0.202250368267511,0.218968937117607),
 .UNSPECIFIED.);
#2439=B_SPLINE_CURVE_WITH_KNOTS('',3,(#46308,#46309,#46310,#46311,#46312,
#46313,#46314,#46315,#46316,#46317),.UNSPECIFIED.,.F.,.F.,(4,2,2,2,4),(0.267904010195979,
0.295535379633993,0.324004413516352,0.353425955511146,0.373790461969576),
 .UNSPECIFIED.);
#2440=B_SPLINE_CURVE_WITH_KNOTS('',3,(#46319,#46320,#46321,#46322,#46323,
#46324,#46325,#46326,#46327,#46328,#46329),.UNSPECIFIED.,.F.,.F.,(4,2,3,
2,4),(-0.218968937118343,-0.202250368267423,0.,0.202250368267423,0.218968937117866),
 .UNSPECIFIED.);
#2441=B_SPLINE_CURVE_WITH_KNOTS('',3,(#46331,#46332,#46333,#46334,#46335,
#46336,#46337,#46338,#46339,#46340),.UNSPECIFIED.,.F.,.F.,(4,2,2,2,4),(0.267904010196159,
0.295535379634028,0.324004413516362,0.353425955511117,0.373790461969744),
 .UNSPECIFIED.);
#2442=B_SPLINE_CURVE_WITH_KNOTS('',3,(#46342,#46343,#46344,#46345,#46346,
#46347),.UNSPECIFIED.,.F.,.F.,(4,2,4),(0.,0.202250368267416,0.21896893711845),
 .UNSPECIFIED.);
#2443=B_SPLINE_CURVE_WITH_KNOTS('',3,(#46352,#46353,#46354,#46355,#46356,
#46357),.UNSPECIFIED.,.F.,.F.,(4,2,4),(-0.218968937117756,-0.202250368267416,
0.),.UNSPECIFIED.);
#2444=B_SPLINE_CURVE_WITH_KNOTS('',3,(#46359,#46360,#46361,#46362,#46363,
#46364,#46365,#46366,#46367,#46368),.UNSPECIFIED.,.F.,.F.,(4,2,2,2,4),(0.267904010196074,
0.295535379633993,0.324004413516349,0.353425955511146,0.373790461969709),
 .UNSPECIFIED.);
#2445=B_SPLINE_CURVE_WITH_KNOTS('',3,(#46369,#46370,#46371,#46372,#46373,
#46374,#46375,#46376,#46377,#46378,#46379),.UNSPECIFIED.,.F.,.F.,(4,2,3,
2,4),(-0.218968937117586,-0.202250368267507,0.,0.202250368267507,0.218968937118666),
 .UNSPECIFIED.);
#2446=B_SPLINE_CURVE_WITH_KNOTS('',3,(#46414,#46415,#46416,#46417,#46418,
#46419,#46420,#46421,#46422,#46423,#46424,#46425,#46426,#46427,#46428,#46429,
#46430,#46431,#46432,#46433,#46434,#46435,#46436,#46437,#46438,#46439),
 .UNSPECIFIED.,.F.,.F.,(4,2,2,2,2,2,2,2,2,2,2,2,4),(1.6778324559149,1.72014131704469,
1.79018729092096,1.88481538797586,1.95967575697182,2.03596140156688,2.11055839736739,
2.1861310055091,2.25999784739323,2.32219814460217,2.41722647505349,2.46648828140439,
2.51647759383358),.UNSPECIFIED.);
#2447=B_SPLINE_CURVE_WITH_KNOTS('',3,(#46442,#46443,#46444,#46445,#46446,
#46447,#46448,#46449,#46450,#46451,#46452,#46453,#46454,#46455,#46456,#46457,
#46458,#46459,#46460,#46461,#46462,#46463,#46464,#46465,#46466,#46467,#46468,
#46469,#46470,#46471,#46472,#46473,#46474,#46475,#46476,#46477,#46478,#46479,
#46480,#46481,#46482,#46483,#46484,#46485,#46486,#46487),.UNSPECIFIED.,
 .F.,.F.,(4,2,2,2,2,2,2,2,2,2,2,2,2,2,2,2,2,2,2,2,2,2,4),(1.15114226328039E-5,
0.0649848036365928,0.127981322338831,0.255478974596226,0.331652000771546,
0.409872196413906,0.486219934049148,0.564442937902226,0.640587838009818,
0.718804933776125,0.795179715777592,0.873400886535082,0.949509589781659,
1.02772338331364,1.10413447964806,1.18235401068144,1.25841586014867,1.33116362067197,
1.39373306987938,1.45442777298624,1.59477450954928,1.63378500658915,1.6778324559149),
 .UNSPECIFIED.);
#2448=B_SPLINE_CURVE_WITH_KNOTS('',3,(#46490,#46491,#46492,#46493,#46494,
#46495),.UNSPECIFIED.,.F.,.F.,(4,2,4),(-0.0531336167389032,-0.0265660123967773,
-4.38116269941419E-6),.UNSPECIFIED.);
#2449=B_SPLINE_CURVE_WITH_KNOTS('',3,(#46497,#46498,#46499,#46500,#46501,
#46502),.UNSPECIFIED.,.F.,.F.,(4,2,4),(-0.0218956957452984,-0.0109537633218819,
-1.19176186653708E-5),.UNSPECIFIED.);
#2450=B_SPLINE_CURVE_WITH_KNOTS('',3,(#46503,#46504,#46505,#46506,#46507,
#46508),.UNSPECIFIED.,.F.,.F.,(4,2,4),(-0.0531191162051923,-0.026569992816066,
-2.41222135409933E-6),.UNSPECIFIED.);
#2451=B_SPLINE_CURVE_WITH_KNOTS('',3,(#46779,#46780,#46781,#46782,#46783,
#46784,#46785,#46786,#46787,#46788,#46789,#46790,#46791,#46792,#46793,#46794,
#46795,#46796,#46797,#46798,#46799,#46800,#46801,#46802,#46803,#46804,#46805,
#46806,#46807,#46808,#46809,#46810,#46811,#46812,#46813,#46814,#46815,#46816,
#46817,#46818,#46819,#46820,#46821,#46822,#46823,#46824,#46825,#46826,#46827,
#46828,#46829,#46830,#46831,#46832,#46833,#46834,#46835,#46836,#46837,#46838,
#46839,#46840,#46841,#46842),.UNSPECIFIED.,.F.,.F.,(4,2,2,2,2,2,2,2,2,2,
2,2,2,2,2,2,2,2,2,2,2,2,2,2,2,2,2,2,2,2,2,4),(7.36481248802261E-6,0.0579261863271751,
0.114674480656631,0.225347966852895,0.303563316130361,0.375602352513824,
0.453406536051233,0.52859202455298,0.606172616816621,0.682782389736415,
0.749975319947736,0.789346627707107,0.867396567563414,0.945814740155127,
1.02375669910915,1.10207765612309,1.2603944919097,1.41863075344829,1.57694494459286,
1.65531768858497,1.73329243799722,1.81176162349561,1.88982856427288,1.92921183430251,
1.99622866693818,2.07313536180107,2.15061317674896,2.22631027196354,2.3039857757181,
2.41210220258,2.46759986362207,2.52414659527546),.UNSPECIFIED.);
#2452=B_SPLINE_CURVE_WITH_KNOTS('',3,(#46843,#46844,#46845,#46846,#46847,
#46848,#46849,#46850,#46851,#46852,#46853,#46854,#46855,#46856,#46857,#46858,
#46859,#46860,#46861,#46862,#46863,#46864,#46865,#46866,#46867,#46868,#46869,
#46870,#46871,#46872,#46873,#46874,#46875,#46876,#46877,#46878,#46879,#46880,
#46881,#46882,#46883,#46884,#46885,#46886,#46887,#46888,#46889,#46890,#46891,
#46892,#46893,#46894,#46895,#46896,#46897,#46898,#46899,#46900,#46901,#46902,
#46903,#46904,#46905,#46906,#46907,#46908,#46909,#46910,#46911,#46912,#46913,
#46914,#46915,#46916,#46917,#46918,#46919,#46920,#46921,#46922,#46923,#46924,
#46925,#46926,#46927,#46928,#46929,#46930,#46931,#46932,#46933,#46934,#46935,
#46936,#46937,#46938,#46939,#46940,#46941,#46942,#46943,#46944,#46945,#46946,
#46947,#46948,#46949,#46950,#46951,#46952,#46953,#46954,#46955,#46956,#46957,
#46958,#46959,#46960,#46961,#46962,#46963,#46964,#46965,#46966,#46967,#46968,
#46969,#46970,#46971,#46972,#46973,#46974,#46975,#46976,#46977,#46978,#46979,
#46980,#46981,#46982,#46983,#46984,#46985,#46986,#46987,#46988,#46989,#46990,
#46991,#46992,#46993,#46994,#46995,#46996,#46997,#46998,#46999,#47000,#47001,
#47002,#47003,#47004,#47005,#47006,#47007,#47008,#47009,#47010),
 .UNSPECIFIED.,.F.,.F.,(4,2,2,2,2,2,2,2,2,2,2,2,2,2,2,2,2,2,2,2,2,2,2,2,
2,2,2,2,2,2,2,2,2,2,2,2,2,2,2,2,2,2,2,2,2,2,2,2,2,2,2,2,2,2,2,2,2,2,2,2,
2,2,2,2,2,2,2,2,2,2,2,2,2,2,2,2,2,2,2,2,2,2,2,4),(1.24307839451921E-5,0.0500273781858429,
0.099432803829234,0.195716540713382,0.25931817354893,0.337078262407541,
0.41344857617591,0.491361811458937,0.567992316284045,0.685555037500459,
0.763791026299535,0.843756617848861,0.882404673909104,0.998511957697595,
1.03743102042921,1.15497455383376,1.2340055935132,1.31470136763013,1.35366727028043,
1.47047427818367,1.50973762807098,1.58913673742986,1.66712864886114,1.74668253295675,
1.82493349101501,1.90462011905243,1.98308203374839,2.0628836750312,2.14151982609838,
2.26262206703986,2.34260764228006,2.42442363424022,2.50469828881245,2.58645550422729,
2.64529450774882,2.6857733268076,2.76607475517718,2.84663676425656,2.92676812082607,
3.00717695406304,3.16980613391867,3.33233948572403,3.49488234557123,3.57373135676786,
3.65370773327419,3.73415195068027,3.81430460423484,3.8948941969404,3.97521273743168,
4.01569959042438,4.07557765927915,4.15735964286485,4.23756779460293,4.31940929267925,
4.39932515385298,4.52048519992014,4.59929039046647,4.76196968485967,4.9245887247453,
5.08724026339377,5.16760525699317,5.24765305595157,5.3281517942438,5.40837336056063,
5.44882670984173,5.50987808032324,5.59161240552458,5.67174675036586,5.75354015640541,
5.83338037483471,5.9548614177171,6.0337228672632,6.19633644131774,6.35890538617673,
6.5215321367131,6.60193149454333,6.68203660128082,6.76257971195663,6.84285225787908,
6.88331730866563,6.94338925665242,7.02513015990786,7.09949049144025,7.17394332972263),
 .UNSPECIFIED.);
#2453=B_SPLINE_CURVE_WITH_KNOTS('',3,(#47012,#47013,#47014,#47015,#47016,
#47017,#47018,#47019,#47020,#47021,#47022,#47023,#47024,#47025,#47026,#47027,
#47028,#47029,#47030,#47031,#47032,#47033,#47034,#47035,#47036,#47037,#47038,
#47039,#47040,#47041,#47042,#47043,#47044,#47045,#47046,#47047,#47048,#47049,
#47050,#47051,#47052,#47053,#47054,#47055,#47056,#47057,#47058,#47059,#47060,
#47061,#47062,#47063,#47064,#47065,#47066,#47067,#47068,#47069,#47070,#47071,
#47072,#47073,#47074,#47075,#47076,#47077,#47078,#47079,#47080,#47081,#47082,
#47083,#47084,#47085,#47086,#47087,#47088,#47089,#47090,#47091,#47092,#47093,
#47094,#47095,#47096,#47097,#47098,#47099,#47100,#47101,#47102,#47103,#47104,
#47105,#47106,#47107,#47108,#47109,#47110,#47111,#47112,#47113,#47114,#47115,
#47116,#47117,#47118,#47119,#47120,#47121,#47122,#47123,#47124,#47125,#47126,
#47127,#47128,#47129,#47130,#47131,#47132,#47133,#47134,#47135,#47136,#47137,
#47138,#47139,#47140,#47141,#47142,#47143,#47144,#47145,#47146,#47147,#47148,
#47149,#47150,#47151,#47152,#47153,#47154,#47155,#47156,#47157,#47158,#47159,
#47160,#47161,#47162,#47163,#47164,#47165,#47166,#47167,#47168,#47169,#47170,
#47171,#47172,#47173,#47174,#47175,#47176,#47177,#47178,#47179,#47180,#47181,
#47182,#47183,#47184,#47185,#47186,#47187,#47188,#47189,#47190,#47191,#47192,
#47193,#47194,#47195,#47196,#47197,#47198,#47199,#47200,#47201,#47202,#47203,
#47204,#47205,#47206,#47207,#47208,#47209,#47210,#47211,#47212,#47213,#47214,
#47215,#47216,#47217,#47218,#47219,#47220,#47221,#47222,#47223,#47224,#47225,
#47226,#47227,#47228,#47229,#47230,#47231,#47232,#47233,#47234,#47235,#47236,
#47237,#47238,#47239,#47240,#47241,#47242,#47243,#47244,#47245,#47246,#47247,
#47248,#47249,#47250,#47251,#47252,#47253,#47254,#47255,#47256,#47257,#47258,
#47259,#47260,#47261,#47262,#47263,#47264,#47265,#47266,#47267,#47268,#47269,
#47270,#47271,#47272,#47273,#47274,#47275,#47276,#47277,#47278,#47279,#47280,
#47281,#47282,#47283,#47284,#47285,#47286,#47287,#47288,#47289,#47290,#47291,
#47292,#47293,#47294,#47295,#47296,#47297,#47298,#47299,#47300,#47301,#47302,
#47303,#47304,#47305,#47306,#47307,#47308,#47309,#47310,#47311,#47312,#47313,
#47314,#47315,#47316,#47317,#47318,#47319,#47320,#47321,#47322,#47323,#47324,
#47325,#47326,#47327,#47328,#47329,#47330,#47331,#47332,#47333,#47334,#47335,
#47336,#47337,#47338,#47339,#47340,#47341,#47342,#47343,#47344,#47345,#47346,
#47347,#47348,#47349,#47350,#47351,#47352,#47353,#47354,#47355,#47356,#47357,
#47358,#47359,#47360,#47361,#47362,#47363,#47364,#47365,#47366,#47367,#47368,
#47369,#47370,#47371,#47372,#47373,#47374,#47375,#47376,#47377,#47378,#47379,
#47380,#47381,#47382,#47383,#47384,#47385,#47386,#47387,#47388,#47389,#47390,
#47391,#47392,#47393,#47394,#47395,#47396,#47397,#47398,#47399,#47400,#47401,
#47402,#47403,#47404,#47405,#47406,#47407,#47408,#47409,#47410,#47411,#47412,
#47413,#47414,#47415,#47416,#47417,#47418,#47419,#47420,#47421,#47422,#47423,
#47424,#47425,#47426,#47427,#47428,#47429,#47430,#47431,#47432,#47433,#47434,
#47435,#47436,#47437,#47438,#47439,#47440,#47441,#47442,#47443,#47444,#47445,
#47446,#47447,#47448,#47449,#47450,#47451,#47452,#47453,#47454,#47455,#47456,
#47457,#47458,#47459,#47460,#47461,#47462,#47463,#47464,#47465,#47466,#47467,
#47468,#47469,#47470,#47471,#47472,#47473,#47474,#47475,#47476,#47477,#47478,
#47479,#47480,#47481,#47482,#47483,#47484,#47485,#47486,#47487,#47488,#47489,
#47490,#47491,#47492,#47493,#47494,#47495,#47496,#47497,#47498,#47499,#47500,
#47501,#47502,#47503,#47504,#47505,#47506,#47507,#47508,#47509,#47510,#47511,
#47512,#47513,#47514,#47515,#47516,#47517,#47518,#47519,#47520,#47521,#47522,
#47523,#47524,#47525,#47526,#47527,#47528,#47529,#47530,#47531,#47532,#47533,
#47534,#47535,#47536,#47537,#47538,#47539,#47540,#47541,#47542,#47543,#47544,
#47545,#47546,#47547,#47548,#47549,#47550,#47551,#47552,#47553,#47554,#47555,
#47556,#47557,#47558,#47559,#47560,#47561,#47562,#47563,#47564,#47565,#47566,
#47567,#47568,#47569,#47570,#47571,#47572,#47573,#47574,#47575,#47576,#47577,
#47578,#47579,#47580,#47581,#47582,#47583,#47584,#47585,#47586,#47587,#47588,
#47589,#47590,#47591,#47592,#47593,#47594,#47595,#47596,#47597,#47598,#47599,
#47600,#47601,#47602,#47603,#47604,#47605,#47606,#47607,#47608,#47609,#47610,
#47611,#47612,#47613,#47614,#47615,#47616,#47617,#47618,#47619,#47620,#47621,
#47622,#47623,#47624),.UNSPECIFIED.,.F.,.F.,(4,3,3,3,3,3,3,3,3,3,3,3,3,
3,3,3,3,3,3,3,3,3,3,3,3,3,3,3,3,3,3,3,3,3,3,3,3,3,3,3,3,3,3,3,3,3,3,3,3,
3,3,3,3,3,3,3,3,3,3,3,3,3,3,3,3,3,3,3,3,3,3,3,3,3,3,3,3,3,3,3,3,3,3,3,3,
3,3,3,3,3,3,3,3,3,3,3,3,3,3,3,3,3,3,3,3,3,3,3,3,3,3,3,3,3,3,3,3,3,3,3,3,
3,3,3,3,3,3,3,3,3,3,3,3,3,3,3,3,3,3,3,3,3,3,3,3,3,3,3,3,3,3,3,3,3,3,3,3,
3,3,3,3,3,3,3,3,3,3,3,3,3,3,3,3,3,3,3,3,3,3,3,3,3,3,3,3,3,3,3,3,3,3,3,3,
3,3,3,3,3,3,3,3,3,3,3,4),(3.25655971975498E-10,0.006896551724138,0.0124999836137833,
0.01379310344828,0.02068965517241,0.02758620689655,0.0287500147726358,0.03448275862069,
0.04137931034483,0.0449999960540127,0.04827586206897,0.0551724137931,0.061249990576592,
0.06206896551724,0.06896551724138,0.07586206896552,0.0775000201460335,0.08275862068966,
0.08965517241379,0.0937499863389232,0.09655172413793,0.1034482758621,0.109999997295967,
0.1103448275862,0.1172413793103,0.1241379310345,0.126250021167855,0.1310344827586,
0.1379310344828,0.142499980080655,0.1448275862069,0.151724137931,0.1586206896552,
0.15875000071435,0.1655172413793,0.1724137931034,0.17500001705366,0.1793103448276,
0.1862068965517,0.191249978763953,0.1931034482759,0.2,0.2068965517241,0.207500006105615,
0.2137931034483,0.2206896551724,0.223750008641753,0.2275862068966,0.2344827586207,
0.239999982367645,0.2413793103448,0.248275862069,0.2551724137931,0.256250013484736,
0.2620689655172,0.2689655172414,0.272499998025251,0.2758620689655,0.2827586206897,
0.288749989207179,0.2896551724138,0.2965517241379,0.3034482758621,0.305000019440364,
0.3103448275862,0.3172413793103,0.321249987913626,0.3241379310345,0.3310344827586,
0.337499996263586,0.3379310344828,0.3448275862069,0.351724137931,0.353750021363703,
0.3586206896552,0.3655172413793,0.369999980876539,0.3724137931034,0.3793103448276,
0.3862068965517,0.3931034482759,0.4,0.40250001816575,0.4068965517241,0.4137931034483,
0.41874997861438,0.4206896551724,0.4275862068966,0.4344827586207,0.435000004876984,
0.4413793103448,0.448275862069,0.451250010408905,0.4551724137931,0.4620689655172,
0.46749998140113,0.4689655172414,0.4758620689655,0.4827586206897,0.483750012153462,
0.4896551724138,0.4965517241379,0.499999999999995,0.5034482758621,0.5103448275862,
0.516249987846535,0.5172413793103,0.5241379310345,0.5310344827586,0.532500018598869,
0.5379310344828,0.5448275862069,0.548749989591095,0.551724137931,0.5586206896552,
0.564999995123012,0.5655172413793,0.5724137931034,0.5793103448276,0.581250021385624,
0.5862068965517,0.5931034482759,0.597499981834243,0.6,0.6068965517241,0.6137931034483,
0.6206896551724,0.6275862068966,0.630000019123452,0.6344827586207,0.6413793103448,
0.646249978636291,0.648275862069,0.6551724137931,0.6620689655172,0.662500003736419,
0.6689655172414,0.6758620689655,0.678750012086381,0.6827586206897,0.6896551724138,
0.694999980559641,0.6965517241379,0.7034482758621,0.7103448275862,0.711250010792824,
0.7172413793103,0.7241379310345,0.727500001974746,0.7310344827586,0.7379310344828,
0.743749986515264,0.7448275862069,0.751724137931,0.7586206896552,0.760000017632363,
0.7655172413793,0.7724137931034,0.776249991358243,0.7793103448276,0.7862068965517,
0.792499993894376,0.7931034482759,0.8,0.8068965517241,0.808750021236045,
0.8137931034483,0.8206896551724,0.82499998294634,0.8275862068966,0.8344827586207,
0.841249999285646,0.8413793103448,0.848275862069,0.8551724137931,0.85750001991935,
0.8620689655172,0.8689655172414,0.873749978832143,0.8758620689655,0.8827586206897,
0.8896551724138,0.890000002704033,0.8965517241379,0.9034482758621,0.906250013661082,
0.9103448275862,0.9172413793103,0.922499979853959,0.9241379310345,0.9310344827586,
0.9379310344828,0.938750009423415,0.9448275862069,0.951724137931,0.955000003945983,
0.9586206896552,0.9655172413793,0.971249985227355,0.9724137931034,0.9793103448276,
0.9862068965517,0.98750001638623,0.9931034482759,0.999999999088867),
 .UNSPECIFIED.);
#2454=B_SPLINE_CURVE_WITH_KNOTS('',3,(#47895,#47896,#47897,#47898,#47899,
#47900,#47901,#47902,#47903,#47904,#47905,#47906,#47907,#47908,#47909,#47910,
#47911,#47912,#47913,#47914,#47915,#47916,#47917,#47918,#47919,#47920,#47921,
#47922,#47923,#47924,#47925,#47926,#47927,#47928,#47929,#47930,#47931,#47932,
#47933,#47934,#47935,#47936,#47937,#47938,#47939,#47940,#47941,#47942,#47943,
#47944,#47945,#47946,#47947,#47948,#47949,#47950,#47951,#47952,#47953,#47954,
#47955,#47956,#47957,#47958,#47959,#47960,#47961,#47962,#47963,#47964,#47965,
#47966,#47967,#47968,#47969,#47970,#47971,#47972,#47973,#47974,#47975,#47976,
#47977,#47978,#47979,#47980,#47981,#47982,#47983,#47984,#47985,#47986,#47987,
#47988,#47989,#47990,#47991,#47992,#47993,#47994,#47995,#47996,#47997,#47998,
#47999,#48000,#48001,#48002,#48003,#48004,#48005,#48006,#48007,#48008,#48009,
#48010,#48011,#48012,#48013,#48014,#48015,#48016,#48017,#48018,#48019,#48020,
#48021,#48022,#48023,#48024,#48025,#48026,#48027,#48028,#48029,#48030,#48031,
#48032,#48033,#48034,#48035,#48036,#48037,#48038,#48039,#48040,#48041,#48042,
#48043,#48044,#48045,#48046,#48047,#48048,#48049,#48050,#48051,#48052,#48053,
#48054,#48055,#48056,#48057,#48058,#48059,#48060),.UNSPECIFIED.,.F.,.F.,
(4,2,2,2,2,2,2,2,2,2,2,2,2,2,2,2,2,2,2,2,2,2,2,2,2,2,2,2,2,2,2,2,2,2,2,
2,2,2,2,2,2,2,2,2,2,2,2,2,2,2,2,2,2,2,2,2,2,2,2,2,2,2,2,2,2,2,2,2,2,2,2,
2,2,2,2,2,2,2,2,2,2,2,4),(1.24307838879642E-5,0.0646066183114824,0.12856607719689,
0.254865757065513,0.372586486589494,0.449979962307396,0.529184791067371,
0.606862719354848,0.686010979860581,0.744503176051179,0.783677591093499,
0.861352736963718,0.939287795082856,1.09685206179482,1.25431390180843,1.41176835032023,
1.48820524639062,1.60667073493631,1.68398378903913,1.76316312364665,1.80149266896066,
1.87901566013445,1.95514961899729,2.03282673397556,2.10922039203301,2.18702955426342,
2.26363435169808,2.3415577655465,2.41833663806098,2.53655733854788,2.61466702094577,
2.69456135835026,2.77295307250581,2.8527899969026,2.91011937237683,2.94964851629334,
3.02806833447274,3.10674296165139,3.18499796256133,3.26352190353714,3.42232679541464,
3.50005504605113,3.65720764541172,3.81435430173883,3.8922586891329,3.97064841787099,
4.04872265952644,4.1272404412672,4.20548511978754,4.28415133142332,4.36254991085045,
4.40206259190978,4.45974116890874,4.53954264803744,4.61782220009431,4.69768194550285,
4.77567736887365,4.89370244308361,4.97054560362708,5.04848147348265,5.12518346334503,
5.20301839793177,5.27955407125725,5.35727542243828,5.43361193177689,5.5112037764545,
5.587297988917,5.66474041371507,5.70304440969069,5.81603976418334,5.85399652301374,
5.93267626293519,6.00983067657395,6.08856751052276,6.16543987971809,6.28216635188411,
6.35802486747928,6.51454555434391,6.67101557798643,6.82752506424321,6.86956990518419,
6.93242642201505,6.99601164762652),.UNSPECIFIED.);
#2455=B_SPLINE_CURVE_WITH_KNOTS('',3,(#48064,#48065,#48066,#48067,#48068,
#48069,#48070,#48071,#48072,#48073,#48074,#48075,#48076,#48077,#48078,#48079,
#48080,#48081,#48082,#48083,#48084,#48085,#48086,#48087,#48088,#48089,#48090,
#48091,#48092,#48093,#48094,#48095,#48096,#48097,#48098,#48099,#48100,#48101,
#48102,#48103,#48104,#48105,#48106,#48107,#48108,#48109,#48110,#48111,#48112,
#48113,#48114,#48115,#48116,#48117,#48118,#48119,#48120,#48121,#48122,#48123,
#48124,#48125,#48126,#48127,#48128,#48129,#48130,#48131,#48132,#48133,#48134,
#48135,#48136,#48137,#48138,#48139,#48140,#48141,#48142,#48143,#48144,#48145,
#48146,#48147,#48148,#48149,#48150,#48151,#48152,#48153,#48154,#48155,#48156,
#48157,#48158,#48159,#48160,#48161,#48162,#48163,#48164,#48165,#48166,#48167,
#48168,#48169,#48170,#48171,#48172,#48173,#48174,#48175,#48176,#48177,#48178,
#48179,#48180,#48181,#48182,#48183,#48184,#48185,#48186,#48187,#48188,#48189,
#48190,#48191,#48192,#48193,#48194,#48195,#48196,#48197,#48198,#48199,#48200,
#48201,#48202,#48203,#48204,#48205,#48206,#48207,#48208,#48209,#48210,#48211,
#48212,#48213,#48214,#48215,#48216,#48217,#48218,#48219,#48220,#48221,#48222,
#48223,#48224,#48225,#48226,#48227,#48228,#48229,#48230,#48231,#48232,#48233,
#48234,#48235,#48236,#48237,#48238,#48239,#48240,#48241,#48242,#48243,#48244,
#48245,#48246,#48247,#48248,#48249,#48250,#48251,#48252,#48253,#48254,#48255,
#48256,#48257,#48258,#48259,#48260,#48261,#48262,#48263,#48264,#48265,#48266,
#48267,#48268,#48269,#48270,#48271,#48272,#48273,#48274,#48275,#48276,#48277,
#48278,#48279,#48280,#48281,#48282,#48283,#48284,#48285,#48286,#48287,#48288,
#48289,#48290,#48291,#48292,#48293,#48294,#48295,#48296,#48297,#48298,#48299,
#48300,#48301,#48302,#48303,#48304,#48305,#48306,#48307,#48308,#48309,#48310,
#48311,#48312,#48313,#48314,#48315,#48316,#48317,#48318,#48319,#48320,#48321,
#48322,#48323,#48324,#48325,#48326,#48327,#48328,#48329,#48330,#48331,#48332,
#48333,#48334,#48335,#48336,#48337,#48338,#48339,#48340,#48341,#48342,#48343,
#48344,#48345,#48346,#48347,#48348,#48349,#48350,#48351,#48352,#48353,#48354,
#48355,#48356,#48357,#48358,#48359,#48360,#48361,#48362,#48363,#48364,#48365,
#48366,#48367,#48368,#48369,#48370,#48371,#48372,#48373,#48374,#48375,#48376,
#48377,#48378,#48379,#48380,#48381,#48382,#48383,#48384,#48385,#48386,#48387,
#48388,#48389,#48390,#48391,#48392,#48393,#48394,#48395,#48396,#48397,#48398,
#48399,#48400,#48401,#48402,#48403,#48404,#48405,#48406,#48407,#48408,#48409,
#48410,#48411,#48412,#48413,#48414,#48415,#48416,#48417,#48418,#48419,#48420,
#48421,#48422,#48423,#48424,#48425,#48426,#48427,#48428,#48429,#48430,#48431,
#48432,#48433,#48434,#48435,#48436,#48437,#48438,#48439,#48440,#48441,#48442,
#48443,#48444,#48445,#48446,#48447,#48448,#48449,#48450,#48451,#48452,#48453,
#48454,#48455,#48456,#48457,#48458,#48459,#48460,#48461,#48462,#48463,#48464,
#48465,#48466,#48467,#48468,#48469,#48470,#48471,#48472,#48473,#48474,#48475,
#48476,#48477,#48478,#48479,#48480,#48481,#48482,#48483,#48484,#48485,#48486,
#48487,#48488,#48489,#48490,#48491,#48492,#48493,#48494,#48495,#48496,#48497,
#48498,#48499,#48500,#48501,#48502,#48503,#48504,#48505,#48506,#48507,#48508,
#48509,#48510,#48511,#48512,#48513,#48514,#48515,#48516,#48517,#48518,#48519,
#48520,#48521,#48522,#48523,#48524,#48525,#48526,#48527,#48528,#48529,#48530,
#48531,#48532,#48533,#48534,#48535,#48536,#48537,#48538,#48539,#48540,#48541,
#48542,#48543,#48544,#48545,#48546,#48547,#48548,#48549,#48550,#48551,#48552,
#48553,#48554,#48555,#48556,#48557,#48558,#48559,#48560,#48561,#48562,#48563,
#48564,#48565,#48566,#48567,#48568,#48569,#48570,#48571,#48572,#48573,#48574,
#48575,#48576,#48577,#48578,#48579,#48580,#48581,#48582,#48583,#48584,#48585,
#48586,#48587,#48588,#48589,#48590,#48591,#48592,#48593,#48594,#48595,#48596,
#48597,#48598,#48599,#48600,#48601,#48602,#48603,#48604,#48605,#48606,#48607,
#48608,#48609,#48610,#48611,#48612,#48613,#48614,#48615,#48616,#48617,#48618,
#48619,#48620,#48621,#48622,#48623,#48624,#48625,#48626,#48627,#48628,#48629,
#48630,#48631,#48632,#48633,#48634,#48635,#48636,#48637,#48638,#48639,#48640,
#48641,#48642,#48643,#48644,#48645,#48646,#48647,#48648,#48649,#48650,#48651,
#48652,#48653,#48654,#48655,#48656,#48657,#48658,#48659,#48660,#48661,#48662,
#48663,#48664,#48665,#48666,#48667,#48668,#48669,#48670,#48671,#48672,#48673,
#48674,#48675,#48676),.UNSPECIFIED.,.F.,.F.,(4,3,3,3,3,3,3,3,3,3,3,3,3,
3,3,3,3,3,3,3,3,3,3,3,3,3,3,3,3,3,3,3,3,3,3,3,3,3,3,3,3,3,3,3,3,3,3,3,3,
3,3,3,3,3,3,3,3,3,3,3,3,3,3,3,3,3,3,3,3,3,3,3,3,3,3,3,3,3,3,3,3,3,3,3,3,
3,3,3,3,3,3,3,3,3,3,3,3,3,3,3,3,3,3,3,3,3,3,3,3,3,3,3,3,3,3,3,3,3,3,3,3,
3,3,3,3,3,3,3,3,3,3,3,3,3,3,3,3,3,3,3,3,3,3,3,3,3,3,3,3,3,3,3,3,3,3,3,3,
3,3,3,3,3,3,3,3,3,3,3,3,3,3,3,3,3,3,3,3,3,3,3,3,3,3,3,3,3,3,3,3,3,3,3,3,
3,3,3,3,3,3,3,3,3,3,3,4),(0.,0.006896551724138,0.0124999836137735,0.01379310344828,
0.02068965517241,0.02758620689655,0.0287500147726293,0.03448275862069,0.04137931034483,
0.0449999960540111,0.04827586206897,0.0551724137931,0.061249990576592,0.06206896551724,
0.06896551724138,0.07586206896552,0.077500020146031,0.08275862068966,0.08965517241379,
0.0937499863389159,0.09655172413793,0.1034482758621,0.109999997295967,0.1103448275862,
0.1172413793103,0.1241379310345,0.126250021167858,0.1310344827586,0.1379310344828,
0.142499980080653,0.1448275862069,0.151724137931,0.1586206896552,0.15875000071435,
0.1655172413793,0.1724137931034,0.175000017053664,0.1793103448276,0.1862068965517,
0.191249978763952,0.1931034482759,0.2,0.2068965517241,0.207500006105622,
0.2137931034483,0.2206896551724,0.223750008641754,0.2275862068966,0.2344827586207,
0.239999982367649,0.2413793103448,0.248275862069,0.2551724137931,0.256250013484739,
0.2620689655172,0.2689655172414,0.272499998025252,0.2758620689655,0.2827586206897,
0.288749989207176,0.2896551724138,0.2965517241379,0.3034482758621,0.305000019440357,
0.3103448275862,0.3172413793103,0.321249987913624,0.3241379310345,0.3310344827586,
0.337499996263584,0.3379310344828,0.3448275862069,0.351724137931,0.353750021363705,
0.3586206896552,0.3655172413793,0.369999980876542,0.3724137931034,0.3793103448276,
0.3862068965517,0.3931034482759,0.4,0.402500018165757,0.4068965517241,0.4137931034483,
0.418749978614374,0.4206896551724,0.4275862068966,0.4344827586207,0.435000004876983,
0.4413793103448,0.448275862069,0.451250010408905,0.4551724137931,0.4620689655172,
0.467499981401136,0.4689655172414,0.4758620689655,0.4827586206897,0.483750012153467,
0.4896551724138,0.4965517241379,0.5,0.5034482758621,0.5103448275862,0.516249987846536,
0.5172413793103,0.5241379310345,0.5310344827586,0.532500018598866,0.5379310344828,
0.5448275862069,0.548749989591093,0.551724137931,0.5586206896552,0.564999995123015,
0.5655172413793,0.5724137931034,0.5793103448276,0.581250021385624,0.5862068965517,
0.5931034482759,0.597499981834247,0.6,0.6068965517241,0.6137931034483,0.6206896551724,
0.6275862068966,0.63000001912345,0.6344827586207,0.6413793103448,0.646249978636288,
0.648275862069,0.6551724137931,0.6620689655172,0.662500003736417,0.6689655172414,
0.6758620689655,0.678750012086376,0.6827586206897,0.6896551724138,0.694999980559646,
0.6965517241379,0.7034482758621,0.7103448275862,0.711250010792826,0.7172413793103,
0.7241379310345,0.727500001974747,0.7310344827586,0.7379310344828,0.74374998651526,
0.7448275862069,0.751724137931,0.7586206896552,0.760000017632353,0.7655172413793,
0.7724137931034,0.776249991358242,0.7793103448276,0.7862068965517,0.792499993894378,
0.7931034482759,0.8,0.8068965517241,0.808750021236051,0.8137931034483,0.8206896551724,
0.824999982946336,0.8275862068966,0.8344827586207,0.841249999285647,0.8413793103448,
0.848275862069,0.8551724137931,0.857500019919344,0.8620689655172,0.8689655172414,
0.873749978832139,0.8758620689655,0.8827586206897,0.8896551724138,0.890000002704037,
0.8965517241379,0.9034482758621,0.906250013661088,0.9103448275862,0.9172413793103,
0.922499979853961,0.9241379310345,0.9310344827586,0.9379310344828,0.938750009423416,
0.9448275862069,0.951724137931,0.955000003945986,0.9586206896552,0.9655172413793,
0.971249985227364,0.9724137931034,0.9793103448276,0.9862068965517,0.987500016386232,
0.9931034482759,0.999999999674344),.UNSPECIFIED.);
#2456=B_SPLINE_CURVE_WITH_KNOTS('',3,(#48947,#48948,#48949,#48950,#48951,
#48952,#48953,#48954,#48955,#48956,#48957,#48958,#48959,#48960,#48961,#48962,
#48963,#48964,#48965,#48966,#48967,#48968,#48969,#48970,#48971,#48972,#48973,
#48974,#48975,#48976,#48977,#48978,#48979,#48980,#48981,#48982,#48983,#48984,
#48985,#48986,#48987,#48988,#48989,#48990,#48991,#48992,#48993,#48994,#48995,
#48996,#48997,#48998,#48999,#49000,#49001,#49002,#49003,#49004,#49005,#49006,
#49007,#49008,#49009,#49010),.UNSPECIFIED.,.F.,.F.,(4,2,2,2,2,2,2,2,2,2,
2,2,2,2,2,2,2,2,2,2,2,2,2,2,2,2,2,2,2,2,2,4),(-1.66633732000905,-1.59703627011939,
-1.52852012575264,-1.48286496355783,-1.4338739966197,-1.40938609426276,
-1.36138358442955,-1.31255473680488,-1.26336425821289,-1.21403314958031,
-1.1641700898921,-1.06400329438633,-1.0149699430902,-0.965942177532495,
-0.917273319565972,-0.869153345373983,-0.844143351275243,-0.794731617877203,
-0.745484131964617,-0.644804715310458,-0.594705472366083,-0.545267901785368,
-0.496092822607313,-0.44725089796995,-0.398871422897544,-0.374356052946474,
-0.326915236742278,-0.277301516825421,-0.227751301391206,-0.128642088715264,
-0.0642903176182427,-1.08468575917311E-5),.UNSPECIFIED.);
#2457=B_SPLINE_CURVE_WITH_KNOTS('',3,(#49012,#49013,#49014,#49015,#49016,
#49017,#49018,#49019,#49020,#49021,#49022,#49023,#49024,#49025,#49026,#49027,
#49028,#49029,#49030,#49031,#49032,#49033,#49034,#49035,#49036,#49037,#49038,
#49039,#49040,#49041,#49042,#49043,#49044,#49045,#49046,#49047,#49048,#49049,
#49050,#49051,#49052,#49053,#49054,#49055,#49056,#49057,#49058,#49059,#49060,
#49061,#49062,#49063,#49064,#49065,#49066,#49067,#49068,#49069,#49070,#49071,
#49072,#49073,#49074,#49075,#49076,#49077,#49078,#49079,#49080,#49081,#49082,
#49083,#49084,#49085,#49086,#49087,#49088,#49089,#49090,#49091,#49092,#49093,
#49094,#49095,#49096,#49097,#49098,#49099,#49100,#49101,#49102,#49103,#49104,
#49105,#49106,#49107,#49108,#49109,#49110,#49111,#49112,#49113,#49114,#49115,
#49116,#49117,#49118,#49119,#49120,#49121,#49122,#49123,#49124,#49125,#49126,
#49127,#49128,#49129,#49130,#49131,#49132,#49133,#49134,#49135,#49136,#49137,
#49138,#49139,#49140,#49141,#49142,#49143,#49144,#49145,#49146,#49147,#49148,
#49149,#49150,#49151,#49152,#49153,#49154,#49155,#49156,#49157,#49158,#49159,
#49160,#49161,#49162,#49163,#49164,#49165,#49166,#49167,#49168,#49169,#49170,
#49171,#49172,#49173,#49174,#49175,#49176,#49177,#49178,#49179,#49180,#49181,
#49182,#49183,#49184,#49185,#49186,#49187,#49188,#49189,#49190,#49191,#49192,
#49193,#49194,#49195,#49196,#49197,#49198,#49199,#49200,#49201,#49202,#49203,
#49204,#49205,#49206,#49207,#49208,#49209,#49210,#49211,#49212,#49213,#49214,
#49215,#49216,#49217,#49218,#49219,#49220,#49221,#49222,#49223,#49224,#49225,
#49226,#49227,#49228,#49229,#49230,#49231,#49232,#49233,#49234,#49235,#49236,
#49237,#49238,#49239,#49240,#49241,#49242,#49243,#49244,#49245,#49246,#49247,
#49248,#49249,#49250,#49251,#49252,#49253,#49254,#49255,#49256,#49257,#49258,
#49259,#49260,#49261,#49262,#49263,#49264,#49265,#49266,#49267,#49268,#49269,
#49270,#49271,#49272,#49273,#49274,#49275,#49276,#49277,#49278,#49279,#49280,
#49281,#49282,#49283,#49284,#49285,#49286,#49287,#49288,#49289,#49290,#49291,
#49292,#49293,#49294,#49295,#49296,#49297,#49298,#49299,#49300,#49301,#49302,
#49303,#49304,#49305,#49306,#49307,#49308,#49309,#49310,#49311,#49312,#49313,
#49314,#49315,#49316,#49317,#49318,#49319,#49320,#49321,#49322,#49323,#49324,
#49325,#49326,#49327,#49328,#49329,#49330,#49331,#49332,#49333,#49334,#49335,
#49336,#49337,#49338,#49339,#49340,#49341,#49342,#49343,#49344,#49345,#49346,
#49347,#49348,#49349,#49350,#49351,#49352,#49353,#49354,#49355,#49356,#49357,
#49358,#49359,#49360,#49361,#49362,#49363,#49364,#49365,#49366,#49367,#49368,
#49369,#49370,#49371,#49372,#49373,#49374,#49375,#49376,#49377,#49378,#49379,
#49380,#49381,#49382,#49383,#49384,#49385,#49386,#49387,#49388,#49389,#49390,
#49391,#49392,#49393,#49394,#49395,#49396,#49397,#49398,#49399,#49400,#49401,
#49402,#49403,#49404,#49405,#49406,#49407,#49408,#49409,#49410,#49411,#49412,
#49413,#49414,#49415,#49416,#49417,#49418,#49419,#49420,#49421,#49422,#49423,
#49424,#49425,#49426,#49427,#49428,#49429,#49430,#49431,#49432,#49433,#49434,
#49435,#49436,#49437,#49438,#49439,#49440,#49441,#49442,#49443,#49444,#49445,
#49446,#49447,#49448,#49449,#49450,#49451,#49452,#49453,#49454,#49455,#49456,
#49457,#49458,#49459,#49460,#49461,#49462,#49463,#49464,#49465,#49466,#49467,
#49468,#49469,#49470,#49471,#49472,#49473,#49474,#49475,#49476,#49477,#49478,
#49479,#49480,#49481,#49482,#49483,#49484,#49485,#49486,#49487,#49488,#49489,
#49490,#49491,#49492,#49493,#49494,#49495,#49496,#49497,#49498,#49499,#49500,
#49501,#49502,#49503,#49504,#49505,#49506,#49507,#49508,#49509,#49510,#49511,
#49512,#49513,#49514,#49515,#49516,#49517,#49518,#49519,#49520,#49521,#49522,
#49523,#49524,#49525,#49526,#49527,#49528,#49529,#49530,#49531,#49532,#49533,
#49534,#49535,#49536,#49537,#49538,#49539,#49540,#49541,#49542,#49543,#49544,
#49545,#49546,#49547,#49548,#49549,#49550,#49551,#49552,#49553,#49554,#49555,
#49556,#49557,#49558,#49559,#49560,#49561,#49562,#49563,#49564,#49565,#49566,
#49567,#49568,#49569,#49570,#49571,#49572,#49573,#49574,#49575,#49576,#49577,
#49578,#49579,#49580,#49581,#49582,#49583,#49584,#49585,#49586,#49587,#49588,
#49589,#49590,#49591,#49592,#49593,#49594,#49595,#49596,#49597,#49598,#49599,
#49600,#49601,#49602,#49603,#49604,#49605,#49606,#49607,#49608,#49609,#49610,
#49611,#49612,#49613,#49614,#49615,#49616,#49617,#49618,#49619,#49620,#49621,
#49622,#49623,#49624),.UNSPECIFIED.,.F.,.F.,(4,3,3,3,3,3,3,3,3,3,3,3,3,
3,3,3,3,3,3,3,3,3,3,3,3,3,3,3,3,3,3,3,3,3,3,3,3,3,3,3,3,3,3,3,3,3,3,3,3,
3,3,3,3,3,3,3,3,3,3,3,3,3,3,3,3,3,3,3,3,3,3,3,3,3,3,3,3,3,3,3,3,3,3,3,3,
3,3,3,3,3,3,3,3,3,3,3,3,3,3,3,3,3,3,3,3,3,3,3,3,3,3,3,3,3,3,3,3,3,3,3,3,
3,3,3,3,3,3,3,3,3,3,3,3,3,3,3,3,3,3,3,3,3,3,3,3,3,3,3,3,3,3,3,3,3,3,3,3,
3,3,3,3,3,3,3,3,3,3,3,3,3,3,3,3,3,3,3,3,3,3,3,3,3,3,3,3,3,3,3,3,3,3,3,3,
3,3,3,3,3,3,3,3,3,3,3,4),(0.,0.006896551724138,0.0124999836137735,0.01379310344828,
0.02068965517241,0.02758620689655,0.0287500147726293,0.03448275862069,0.04137931034483,
0.0449999960540111,0.04827586206897,0.0551724137931,0.061249990576592,0.06206896551724,
0.06896551724138,0.07586206896552,0.077500020146031,0.08275862068966,0.08965517241379,
0.0937499863389159,0.09655172413793,0.1034482758621,0.109999997295967,0.1103448275862,
0.1172413793103,0.1241379310345,0.126250021167858,0.1310344827586,0.1379310344828,
0.142499980080653,0.1448275862069,0.151724137931,0.1586206896552,0.15875000071435,
0.1655172413793,0.1724137931034,0.175000017053664,0.1793103448276,0.1862068965517,
0.191249978763952,0.1931034482759,0.2,0.2068965517241,0.207500006105622,
0.2137931034483,0.2206896551724,0.223750008641754,0.2275862068966,0.2344827586207,
0.239999982367649,0.2413793103448,0.248275862069,0.2551724137931,0.256250013484739,
0.2620689655172,0.2689655172414,0.272499998025252,0.2758620689655,0.2827586206897,
0.288749989207176,0.2896551724138,0.2965517241379,0.3034482758621,0.305000019440357,
0.3103448275862,0.3172413793103,0.321249987913624,0.3241379310345,0.3310344827586,
0.337499996263584,0.3379310344828,0.3448275862069,0.351724137931,0.353750021363705,
0.3586206896552,0.3655172413793,0.369999980876542,0.3724137931034,0.3793103448276,
0.3862068965517,0.3931034482759,0.4,0.40250001816575,0.4068965517241,0.4137931034483,
0.418749978614372,0.4206896551724,0.4275862068966,0.4344827586207,0.435000004876983,
0.4413793103448,0.448275862069,0.451250010408905,0.4551724137931,0.4620689655172,
0.467499981401136,0.4689655172414,0.4758620689655,0.4827586206897,0.483750012153467,
0.4896551724138,0.4965517241379,0.5,0.5034482758621,0.5103448275862,0.516249987846536,
0.5172413793103,0.5241379310345,0.5310344827586,0.532500018598866,0.5379310344828,
0.5448275862069,0.548749989591093,0.551724137931,0.5586206896552,0.564999995123015,
0.5655172413793,0.5724137931034,0.5793103448276,0.581250021385624,0.5862068965517,
0.5931034482759,0.597499981834247,0.6,0.6068965517241,0.6137931034483,0.6206896551724,
0.6275862068966,0.63000001912345,0.6344827586207,0.6413793103448,0.646249978636288,
0.648275862069,0.6551724137931,0.6620689655172,0.662500003736417,0.6689655172414,
0.6758620689655,0.678750012086376,0.6827586206897,0.6896551724138,0.694999980559646,
0.6965517241379,0.7034482758621,0.7103448275862,0.711250010792826,0.7172413793103,
0.7241379310345,0.727500001974747,0.7310344827586,0.7379310344828,0.74374998651526,
0.7448275862069,0.751724137931,0.7586206896552,0.760000017632353,0.7655172413793,
0.7724137931034,0.776249991358242,0.7793103448276,0.7862068965517,0.792499993894378,
0.7931034482759,0.8,0.8068965517241,0.808750021236051,0.8137931034483,0.8206896551724,
0.824999982946336,0.8275862068966,0.8344827586207,0.841249999285647,0.8413793103448,
0.848275862069,0.8551724137931,0.857500019919344,0.8620689655172,0.8689655172414,
0.873749978832139,0.8758620689655,0.8827586206897,0.8896551724138,0.890000002704037,
0.8965517241379,0.9034482758621,0.906250013661088,0.9103448275862,0.9172413793103,
0.922499979853961,0.9241379310345,0.9310344827586,0.9379310344828,0.938750009423416,
0.9448275862069,0.951724137931,0.955000003945986,0.9586206896552,0.9655172413793,
0.971249985227364,0.9724137931034,0.9793103448276,0.9862068965517,0.987500016386232,
0.9931034482759,0.999999999699303),.UNSPECIFIED.);
#2458=B_SPLINE_CURVE_WITH_KNOTS('',3,(#49894,#49895,#49896,#49897,#49898,
#49899,#49900,#49901,#49902,#49903,#49904,#49905,#49906,#49907,#49908,#49909,
#49910,#49911,#49912,#49913,#49914,#49915,#49916,#49917,#49918,#49919,#49920,
#49921,#49922,#49923,#49924,#49925,#49926,#49927,#49928,#49929,#49930,#49931,
#49932,#49933,#49934,#49935,#49936,#49937,#49938,#49939,#49940,#49941,#49942,
#49943,#49944,#49945,#49946,#49947,#49948,#49949,#49950,#49951,#49952,#49953,
#49954,#49955,#49956,#49957,#49958,#49959,#49960,#49961,#49962,#49963,#49964,
#49965,#49966,#49967,#49968,#49969,#49970,#49971,#49972,#49973,#49974,#49975,
#49976,#49977,#49978,#49979,#49980,#49981,#49982,#49983,#49984,#49985,#49986,
#49987,#49988,#49989,#49990,#49991,#49992,#49993,#49994,#49995,#49996,#49997,
#49998,#49999,#50000,#50001,#50002,#50003,#50004,#50005,#50006,#50007,#50008,
#50009,#50010,#50011,#50012,#50013,#50014,#50015,#50016,#50017,#50018,#50019,
#50020,#50021,#50022,#50023,#50024,#50025,#50026,#50027,#50028,#50029,#50030,
#50031,#50032,#50033,#50034,#50035,#50036,#50037,#50038,#50039,#50040,#50041,
#50042,#50043,#50044,#50045,#50046,#50047,#50048,#50049,#50050,#50051,#50052,
#50053,#50054,#50055,#50056,#50057,#50058,#50059,#50060,#50061,#50062,#50063,
#50064,#50065,#50066,#50067,#50068,#50069,#50070,#50071,#50072,#50073,#50074,
#50075,#50076,#50077,#50078,#50079,#50080,#50081,#50082,#50083),
 .UNSPECIFIED.,.F.,.F.,(4,2,2,2,2,2,2,2,2,2,2,2,2,2,2,2,2,2,2,2,2,2,2,2,
2,2,2,2,2,2,2,2,2,2,2,2,2,2,2,2,2,2,2,2,2,2,2,2,2,2,2,2,2,2,2,2,2,2,2,2,
2,2,2,2,2,2,2,2,2,2,2,2,2,2,2,2,2,2,2,2,2,2,2,2,2,2,2,2,2,2,2,2,2,2,4),
(-12.5010893468563,-12.3955019246696,-12.29254455623,-12.1459237162089,
-12.0534009089294,-11.9236776502422,-11.7491077006647,-11.6772399648329,
-11.5712782716806,-11.3238756382021,-11.2051337123826,-11.1056993724438,
-11.0021239973504,-10.7378793159625,-10.5155966870519,-10.3512039322814,
-10.1466748655266,-9.87142699075404,-9.73709147703406,-9.53389602132558,
-9.31814598815267,-9.17117893543063,-9.01109017484306,-8.80905691073069,
-8.41805541817743,-8.12716271658195,-8.00669735542938,-7.8039680852172,
-7.53375845441259,-7.40232630908509,-7.27541859109228,-7.1062648398012,
-6.96164817241986,-6.79904573142915,-6.69501805425453,-6.51076918321285,
-6.23766454972543,-6.05716403248301,-5.87761455247391,-5.653672802988,-5.51404475617032,
-5.26873717693825,-5.05382167631166,-4.90073408060745,-4.81137902932328,
-4.51359899975272,-4.42504630749999,-4.34128325511,-4.25738441999853,-4.11551925816328,
-3.92192946120956,-3.72812417494571,-3.61710817639108,-3.40662038260933,
-3.16125849456072,-2.99827957516932,-2.84630234994494,-2.63994642266069,
-2.51541401577412,-2.4373640545864,-2.27085778902812,-2.18206961488083,
-2.10754515662402,-1.99262515056807,-1.85155851909128,-1.77732091277462,
-1.71535701253962,-1.6526902916784,-1.562493505486,-1.50083657181577,-1.46545499373709,
-1.40994218479656,-1.359563114224,-1.29488296358145,-1.26302820187884,-1.21758580791865,
-1.15676382139674,-1.07603643283981,-1.03198768531833,-0.973241214322041,
-0.90395132170858,-0.837813892070961,-0.769710721948455,-0.724142155412939,
-0.67612082666296,-0.625966063761364,-0.560562807638131,-0.497620494482934,
-0.4468543143013,-0.355950889046661,-0.292569617992569,-0.241516995465503,
-0.166846284360261,-0.0399205669991334,-5.63539519875474E-5),
 .UNSPECIFIED.);
#2459=B_SPLINE_CURVE_WITH_KNOTS('',3,(#50084,#50085,#50086,#50087,#50088,
#50089,#50090,#50091,#50092,#50093,#50094,#50095,#50096,#50097,#50098,#50099,
#50100,#50101,#50102,#50103,#50104,#50105,#50106,#50107,#50108,#50109,#50110,
#50111,#50112,#50113,#50114,#50115,#50116,#50117,#50118,#50119,#50120,#50121,
#50122,#50123,#50124,#50125,#50126,#50127,#50128,#50129,#50130,#50131,#50132,
#50133,#50134,#50135,#50136,#50137,#50138,#50139,#50140,#50141,#50142,#50143,
#50144,#50145,#50146,#50147,#50148,#50149,#50150,#50151,#50152,#50153,#50154,
#50155,#50156,#50157,#50158,#50159,#50160,#50161,#50162,#50163,#50164,#50165,
#50166,#50167,#50168,#50169,#50170,#50171,#50172,#50173,#50174,#50175,#50176,
#50177,#50178,#50179,#50180,#50181,#50182,#50183,#50184,#50185,#50186,#50187),
 .UNSPECIFIED.,.F.,.F.,(4,2,2,2,2,2,2,2,2,2,2,2,2,2,2,2,2,2,2,2,2,2,2,2,
2,2,2,2,2,2,2,2,2,2,2,2,2,2,2,2,2,2,2,2,2,2,2,2,2,2,2,4),(-5.72457039602614,
-5.67740959373671,-5.63122585579928,-5.55949891583999,-5.51613971115158,
-5.47294026658525,-5.38759086497003,-5.34869162708517,-5.30945877254513,
-5.22227376857796,-5.16149754031448,-5.11547880467284,-5.06672492745363,
-4.9564919053269,-4.89278834378409,-4.82903674184974,-4.69584725936334,
-4.63115794223737,-4.56625122927357,-4.42357125813279,-4.34725616502263,
-4.26987365048767,-4.1158488390985,-4.03705650559149,-3.9049361991664,-3.8267107788816,
-3.74890540080541,-3.56871767260129,-3.48072229414968,-3.257626156076,-3.12571880576179,
-2.99213032376785,-2.75262686455332,-2.64193775641107,-2.53021199520972,
-2.31081713723528,-2.19937460680053,-1.98583275220802,-1.76266385660368,
-1.65123683467011,-1.43290388293514,-1.32316089943354,-1.21496827736271,
-0.993191000517704,-0.883789162915291,-0.774073723773991,-0.561001501856556,
-0.453917196237877,-0.353256981724687,-0.17227205692989,-0.0868655698498306,
-3.32283829430584E-6),.UNSPECIFIED.);
#2460=B_SPLINE_CURVE_WITH_KNOTS('',3,(#50328,#50329,#50330,#50331,#50332,
#50333,#50334,#50335,#50336,#50337,#50338,#50339,#50340,#50341,#50342,#50343,
#50344,#50345,#50346,#50347,#50348,#50349,#50350,#50351,#50352,#50353,#50354,
#50355,#50356,#50357,#50358,#50359,#50360,#50361,#50362,#50363,#50364,#50365,
#50366,#50367,#50368,#50369,#50370,#50371,#50372,#50373,#50374,#50375,#50376,
#50377,#50378,#50379,#50380,#50381,#50382,#50383,#50384,#50385,#50386,#50387,
#50388,#50389,#50390,#50391,#50392,#50393,#50394,#50395,#50396,#50397,#50398,
#50399,#50400,#50401,#50402,#50403,#50404,#50405,#50406,#50407,#50408,#50409,
#50410,#50411,#50412,#50413,#50414,#50415,#50416,#50417,#50418,#50419,#50420,
#50421,#50422,#50423,#50424,#50425,#50426,#50427,#50428,#50429,#50430,#50431,
#50432,#50433,#50434,#50435,#50436,#50437,#50438,#50439,#50440,#50441,#50442,
#50443,#50444,#50445,#50446,#50447,#50448,#50449,#50450,#50451,#50452,#50453,
#50454,#50455,#50456,#50457,#50458,#50459,#50460,#50461,#50462,#50463,#50464,
#50465,#50466,#50467,#50468,#50469,#50470,#50471,#50472,#50473,#50474,#50475,
#50476,#50477,#50478,#50479,#50480,#50481,#50482,#50483,#50484,#50485,#50486,
#50487,#50488,#50489,#50490,#50491,#50492,#50493,#50494,#50495,#50496,#50497,
#50498,#50499),.UNSPECIFIED.,.F.,.F.,(4,2,2,2,2,2,2,2,2,2,2,2,2,2,2,2,2,
2,2,2,2,2,2,2,2,2,2,2,2,2,2,2,2,2,2,2,2,2,2,2,2,2,2,2,2,2,2,2,2,2,2,2,2,
2,2,2,2,2,2,2,2,2,2,2,2,2,2,2,2,2,2,2,2,2,2,2,2,2,2,2,2,2,2,2,2,4),(0.000470698768311942,
0.148321453566357,0.317425857543853,0.436101923702642,0.557844942473512,
0.744678636579374,0.855687791842655,0.9076686119342,0.983660372768557,1.0725845720498,
1.12117238638503,1.2178861382758,1.27910492119424,1.31465770016191,1.34870198596797,
1.41444082490198,1.45852650913111,1.53071781722442,1.56634174180461,1.6216854737005,
1.66350990999233,1.72858009368055,1.77623273819062,1.83294115633519,1.87503221650589,
1.95031796433434,2.02516118191607,2.09873098639522,2.17430958552449,2.23710534751301,
2.29662438387701,2.44410295517342,2.6462228959603,2.89691576438539,3.0543071171469,
3.20520804542532,3.34590083749761,3.53109280663704,3.66876538880978,3.74839244187486,
3.89972766502862,4.03103446017813,4.10749792180876,4.23142124648352,4.31252932960002,
4.46142079174021,4.54933535333564,4.6710448490143,4.74136792982459,4.89446451461515,
5.00598172369279,5.12745759051139,5.20868840672564,5.33920348711798,5.58984772231306,
5.71210658233482,5.88394566206482,6.19877568160708,6.45985913569223,6.67667688005281,
6.77822327741072,6.87703056315368,6.98871985461782,7.0873938977894,7.16085653401938,
7.32786847784497,7.41628138031729,7.47331330577707,7.54654259779913,7.62125918027395,
7.68880174806676,7.764248864466,7.82221895060197,7.91842932475137,7.98331302303493,
8.07813386136645,8.12849570087089,8.18024002119065,8.26551377880065,8.41891269762442,
8.49837485663615,8.58182636321036,8.69126476283946,8.80338860033424,8.95484442293788,
9.18218359913891),.UNSPECIFIED.);
#2461=B_SPLINE_CURVE_WITH_KNOTS('',3,(#51178,#51179,#51180,#51181,#51182,
#51183,#51184,#51185,#51186,#51187,#51188,#51189,#51190,#51191,#51192,#51193,
#51194,#51195,#51196,#51197,#51198,#51199,#51200,#51201,#51202,#51203,#51204,
#51205,#51206,#51207,#51208,#51209,#51210,#51211,#51212,#51213,#51214,#51215,
#51216,#51217,#51218,#51219,#51220,#51221,#51222,#51223,#51224,#51225,#51226,
#51227,#51228,#51229,#51230,#51231,#51232,#51233,#51234,#51235,#51236,#51237,
#51238,#51239,#51240,#51241,#51242,#51243,#51244,#51245,#51246,#51247,#51248,
#51249,#51250,#51251,#51252,#51253,#51254,#51255,#51256,#51257,#51258,#51259,
#51260,#51261,#51262,#51263,#51264,#51265,#51266,#51267,#51268,#51269,#51270,
#51271,#51272,#51273,#51274,#51275,#51276,#51277,#51278,#51279,#51280,#51281,
#51282,#51283,#51284,#51285,#51286,#51287,#51288,#51289,#51290,#51291,#51292,
#51293,#51294,#51295,#51296,#51297,#51298,#51299,#51300,#51301,#51302,#51303,
#51304,#51305,#51306,#51307,#51308,#51309,#51310,#51311,#51312,#51313,#51314,
#51315,#51316,#51317,#51318,#51319,#51320,#51321,#51322,#51323,#51324,#51325,
#51326,#51327,#51328,#51329,#51330,#51331,#51332,#51333,#51334,#51335,#51336,
#51337,#51338,#51339,#51340,#51341,#51342,#51343,#51344,#51345,#51346,#51347,
#51348,#51349,#51350,#51351,#51352,#51353,#51354,#51355,#51356,#51357,#51358,
#51359,#51360,#51361,#51362,#51363,#51364,#51365,#51366,#51367,#51368,#51369,
#51370,#51371,#51372,#51373,#51374,#51375,#51376,#51377,#51378,#51379,#51380,
#51381,#51382,#51383,#51384,#51385,#51386,#51387,#51388,#51389,#51390,#51391,
#51392,#51393,#51394,#51395,#51396,#51397,#51398,#51399,#51400,#51401,#51402,
#51403,#51404,#51405,#51406,#51407,#51408,#51409,#51410,#51411,#51412,#51413,
#51414,#51415,#51416,#51417,#51418,#51419,#51420,#51421,#51422,#51423,#51424,
#51425,#51426,#51427,#51428,#51429,#51430,#51431,#51432,#51433,#51434,#51435,
#51436,#51437,#51438,#51439,#51440,#51441,#51442,#51443,#51444,#51445,#51446,
#51447,#51448,#51449,#51450,#51451,#51452,#51453,#51454,#51455,#51456,#51457,
#51458,#51459,#51460,#51461,#51462,#51463,#51464,#51465,#51466,#51467,#51468,
#51469,#51470,#51471,#51472,#51473,#51474,#51475,#51476,#51477,#51478,#51479,
#51480,#51481,#51482,#51483,#51484,#51485,#51486,#51487,#51488,#51489,#51490,
#51491,#51492,#51493,#51494,#51495,#51496,#51497,#51498,#51499,#51500,#51501,
#51502,#51503,#51504,#51505,#51506,#51507,#51508,#51509,#51510,#51511,#51512,
#51513,#51514,#51515,#51516,#51517,#51518,#51519,#51520,#51521,#51522,#51523,
#51524,#51525,#51526,#51527,#51528,#51529,#51530,#51531,#51532,#51533,#51534,
#51535,#51536,#51537,#51538,#51539,#51540,#51541,#51542,#51543,#51544,#51545,
#51546,#51547,#51548,#51549,#51550,#51551,#51552,#51553,#51554,#51555,#51556,
#51557,#51558,#51559,#51560,#51561,#51562,#51563,#51564,#51565,#51566,#51567,
#51568,#51569,#51570,#51571,#51572,#51573,#51574,#51575,#51576,#51577,#51578,
#51579,#51580,#51581,#51582,#51583,#51584,#51585,#51586,#51587,#51588,#51589,
#51590,#51591,#51592,#51593,#51594,#51595,#51596,#51597,#51598,#51599,#51600,
#51601,#51602,#51603,#51604,#51605,#51606,#51607,#51608,#51609,#51610,#51611,
#51612,#51613,#51614,#51615,#51616,#51617,#51618,#51619,#51620,#51621,#51622,
#51623,#51624,#51625,#51626,#51627,#51628,#51629,#51630,#51631,#51632,#51633,
#51634,#51635,#51636,#51637,#51638,#51639,#51640,#51641,#51642,#51643,#51644,
#51645,#51646,#51647,#51648,#51649,#51650,#51651,#51652,#51653,#51654,#51655,
#51656,#51657,#51658,#51659,#51660,#51661,#51662,#51663,#51664,#51665,#51666,
#51667,#51668,#51669,#51670,#51671,#51672,#51673,#51674,#51675,#51676,#51677,
#51678,#51679,#51680,#51681,#51682,#51683,#51684,#51685,#51686,#51687,#51688,
#51689,#51690,#51691,#51692,#51693,#51694,#51695,#51696,#51697,#51698,#51699,
#51700,#51701,#51702,#51703,#51704,#51705,#51706,#51707,#51708,#51709,#51710,
#51711,#51712,#51713,#51714,#51715,#51716,#51717,#51718,#51719,#51720,#51721,
#51722,#51723,#51724,#51725,#51726,#51727,#51728,#51729,#51730,#51731,#51732,
#51733,#51734,#51735,#51736,#51737,#51738,#51739,#51740,#51741,#51742,#51743,
#51744,#51745,#51746,#51747,#51748,#51749,#51750,#51751,#51752,#51753,#51754,
#51755,#51756,#51757,#51758,#51759,#51760,#51761,#51762,#51763,#51764,#51765,
#51766,#51767,#51768,#51769,#51770,#51771,#51772,#51773,#51774,#51775,#51776,
#51777,#51778,#51779,#51780,#51781,#51782,#51783,#51784,#51785,#51786,#51787,
#51788,#51789,#51790),.UNSPECIFIED.,.F.,.F.,(4,3,3,3,3,3,3,3,3,3,3,3,3,
3,3,3,3,3,3,3,3,3,3,3,3,3,3,3,3,3,3,3,3,3,3,3,3,3,3,3,3,3,3,3,3,3,3,3,3,
3,3,3,3,3,3,3,3,3,3,3,3,3,3,3,3,3,3,3,3,3,3,3,3,3,3,3,3,3,3,3,3,3,3,3,3,
3,3,3,3,3,3,3,3,3,3,3,3,3,3,3,3,3,3,3,3,3,3,3,3,3,3,3,3,3,3,3,3,3,3,3,3,
3,3,3,3,3,3,3,3,3,3,3,3,3,3,3,3,3,3,3,3,3,3,3,3,3,3,3,3,3,3,3,3,3,3,3,3,
3,3,3,3,3,3,3,3,3,3,3,3,3,3,3,3,3,3,3,3,3,3,3,3,3,3,3,3,3,3,3,3,3,3,3,3,
3,3,3,3,3,3,3,3,3,3,3,4),(3.00696909155215E-10,0.006896551724138,0.0124999836137833,
0.01379310344828,0.02068965517241,0.02758620689655,0.0287500147726358,0.03448275862069,
0.04137931034483,0.0449999960540127,0.04827586206897,0.0551724137931,0.061249990576592,
0.06206896551724,0.06896551724138,0.07586206896552,0.0775000201460335,0.08275862068966,
0.08965517241379,0.0937499863389232,0.09655172413793,0.1034482758621,0.109999997295967,
0.1103448275862,0.1172413793103,0.1241379310345,0.126250021167855,0.1310344827586,
0.1379310344828,0.142499980080655,0.1448275862069,0.151724137931,0.1586206896552,
0.15875000071435,0.1655172413793,0.1724137931034,0.17500001705366,0.1793103448276,
0.1862068965517,0.191249978763953,0.1931034482759,0.2,0.2068965517241,0.207500006105615,
0.2137931034483,0.2206896551724,0.223750008641753,0.2275862068966,0.2344827586207,
0.239999982367645,0.2413793103448,0.248275862069,0.2551724137931,0.256250013484737,
0.2620689655172,0.2689655172414,0.272499998025251,0.2758620689655,0.2827586206897,
0.288749989207179,0.2896551724138,0.2965517241379,0.3034482758621,0.305000019440364,
0.3103448275862,0.3172413793103,0.321249987913626,0.3241379310345,0.3310344827586,
0.337499996263586,0.3379310344828,0.3448275862069,0.351724137931,0.353750021363703,
0.3586206896552,0.3655172413793,0.369999980876539,0.3724137931034,0.3793103448276,
0.3862068965517,0.3931034482759,0.4,0.40250001816575,0.4068965517241,0.4137931034483,
0.41874997861438,0.4206896551724,0.4275862068966,0.4344827586207,0.435000004876984,
0.4413793103448,0.448275862069,0.451250010408905,0.4551724137931,0.4620689655172,
0.46749998140113,0.4689655172414,0.4758620689655,0.4827586206897,0.483750012153462,
0.4896551724138,0.4965517241379,0.499999999999995,0.5034482758621,0.5103448275862,
0.516249987846535,0.5172413793103,0.5241379310345,0.5310344827586,0.532500018598869,
0.5379310344828,0.5448275862069,0.548749989591095,0.551724137931,0.5586206896552,
0.564999995123012,0.5655172413793,0.5724137931034,0.5793103448276,0.581250021385624,
0.5862068965517,0.5931034482759,0.597499981834243,0.6,0.6068965517241,0.6137931034483,
0.6206896551724,0.6275862068966,0.630000019123452,0.6344827586207,0.6413793103448,
0.646249978636291,0.648275862069,0.6551724137931,0.6620689655172,0.662500003736419,
0.6689655172414,0.6758620689655,0.678750012086381,0.6827586206897,0.6896551724138,
0.694999980559641,0.6965517241379,0.7034482758621,0.7103448275862,0.711250010792824,
0.7172413793103,0.7241379310345,0.727500001974746,0.7310344827586,0.7379310344828,
0.743749986515264,0.7448275862069,0.751724137931,0.7586206896552,0.760000017632363,
0.7655172413793,0.7724137931034,0.776249991358243,0.7793103448276,0.7862068965517,
0.792499993894376,0.7931034482759,0.8,0.8068965517241,0.808750021236045,
0.8137931034483,0.8206896551724,0.82499998294634,0.8275862068966,0.8344827586207,
0.841249999285646,0.8413793103448,0.848275862069,0.8551724137931,0.85750001991935,
0.8620689655172,0.8689655172414,0.873749978832143,0.8758620689655,0.8827586206897,
0.8896551724138,0.890000002704033,0.8965517241379,0.9034482758621,0.906250013661082,
0.9103448275862,0.9172413793103,0.922499979853959,0.9241379310345,0.9310344827586,
0.9379310344828,0.938750009423415,0.9448275862069,0.951724137931,0.955000003945983,
0.9586206896552,0.9655172413793,0.971249985227355,0.9724137931034,0.9793103448276,
0.9862068965517,0.98750001638623,0.9931034482759,0.999999999124025),
 .UNSPECIFIED.);
#2896=LINE('',#46206,#3361);
#2897=LINE('',#46384,#3362);
#2898=LINE('',#46385,#3363);
#2899=LINE('',#46388,#3364);
#2900=LINE('',#46392,#3365);
#2901=LINE('',#46396,#3366);
#2902=LINE('',#46400,#3367);
#2903=LINE('',#46404,#3368);
#2904=LINE('',#46407,#3369);
#2905=LINE('',#46412,#3370);
#2906=LINE('',#46441,#3371);
#2907=LINE('',#47625,#3372);
#2908=LINE('',#48062,#3373);
#2909=LINE('',#48677,#3374);
#2910=LINE('',#49625,#3375);
#2911=LINE('',#50640,#3376);
#2912=LINE('',#50909,#3377);
#2913=LINE('',#52060,#3378);
#2914=LINE('',#52062,#3379);
#2915=LINE('',#52064,#3380);
#2916=LINE('',#52066,#3381);
#2917=LINE('',#52068,#3382);
#2918=LINE('',#52070,#3383);
#2919=LINE('',#52072,#3384);
#2920=LINE('',#52074,#3385);
#2921=LINE('',#52076,#3386);
#2922=LINE('',#52078,#3387);
#3361=VECTOR('',#12388,3.125);
#3362=VECTOR('',#12397,1.239616396338);
#3363=VECTOR('',#12398,1.239616396338);
#3364=VECTOR('',#12401,4.61880215351685);
#3365=VECTOR('',#12404,4.618802153517);
#3366=VECTOR('',#12407,4.61880215351685);
#3367=VECTOR('',#12410,4.61880215351685);
#3368=VECTOR('',#12413,4.618802153517);
#3369=VECTOR('',#12416,4.61880215351685);
#3370=VECTOR('',#12421,4.);
#3371=VECTOR('',#12422,0.75);
#3372=VECTOR('',#12425,0.531162247654508);
#3373=VECTOR('',#12426,0.531162247654478);
#3374=VECTOR('',#12427,0.531162247654508);
#3375=VECTOR('',#12428,0.531162247654478);
#3376=VECTOR('',#12429,0.2188377523455);
#3377=VECTOR('',#12430,0.2188377523455);
#3378=VECTOR('',#12433,1.239616396338);
#3379=VECTOR('',#12436,1.239616396338);
#3380=VECTOR('',#12439,1.239616396338);
#3381=VECTOR('',#12442,1.239616396338);
#3382=VECTOR('',#12445,1.239616396338);
#3383=VECTOR('',#12448,1.239616396338);
#3384=VECTOR('',#12451,1.239616396338);
#3385=VECTOR('',#12454,1.239616396338);
#3386=VECTOR('',#12457,1.239616396338);
#3387=VECTOR('',#12460,1.239616396338);
#4197=VERTEX_POINT('',#46064);
#4198=VERTEX_POINT('',#46065);
#4199=VERTEX_POINT('',#46070);
#4200=VERTEX_POINT('',#46165);
#4201=VERTEX_POINT('',#46170);
#4202=VERTEX_POINT('',#46201);
#4203=VERTEX_POINT('',#46204);
#4204=VERTEX_POINT('',#46208);
#4205=VERTEX_POINT('',#46237);
#4206=VERTEX_POINT('',#46238);
#4207=VERTEX_POINT('',#46249);
#4208=VERTEX_POINT('',#46261);
#4209=VERTEX_POINT('',#46272);
#4210=VERTEX_POINT('',#46284);
#4211=VERTEX_POINT('',#46295);
#4212=VERTEX_POINT('',#46307);
#4213=VERTEX_POINT('',#46318);
#4214=VERTEX_POINT('',#46330);
#4215=VERTEX_POINT('',#46341);
#4216=VERTEX_POINT('',#46351);
#4217=VERTEX_POINT('',#46358);
#4218=VERTEX_POINT('',#46381);
#4219=VERTEX_POINT('',#46382);
#4220=VERTEX_POINT('',#46387);
#4221=VERTEX_POINT('',#46389);
#4222=VERTEX_POINT('',#46391);
#4223=VERTEX_POINT('',#46393);
#4224=VERTEX_POINT('',#46395);
#4225=VERTEX_POINT('',#46397);
#4226=VERTEX_POINT('',#46399);
#4227=VERTEX_POINT('',#46401);
#4228=VERTEX_POINT('',#46403);
#4229=VERTEX_POINT('',#46405);
#4230=VERTEX_POINT('',#46408);
#4231=VERTEX_POINT('',#46411);
#4232=VERTEX_POINT('',#46413);
#4233=VERTEX_POINT('',#46440);
#4234=VERTEX_POINT('',#46489);
#4235=VERTEX_POINT('',#46496);
#4236=VERTEX_POINT('',#46777);
#4237=VERTEX_POINT('',#46778);
#4238=VERTEX_POINT('',#47011);
#4239=VERTEX_POINT('',#47894);
#4240=VERTEX_POINT('',#48061);
#4241=VERTEX_POINT('',#48063);
#4242=VERTEX_POINT('',#48946);
#4243=VERTEX_POINT('',#49011);
#5531=EDGE_CURVE('',#4197,#4198,#2428,.T.);
#5532=EDGE_CURVE('',#4197,#4199,#2429,.T.);
#5533=EDGE_CURVE('',#4200,#4199,#2430,.T.);
#5534=EDGE_CURVE('',#4200,#4201,#2431,.T.);
#5535=EDGE_CURVE('',#4201,#4198,#2432,.T.);
#5536=EDGE_CURVE('',#4202,#4202,#2071,.T.);
#5537=EDGE_CURVE('',#4203,#4203,#2072,.T.);
#5538=EDGE_CURVE('',#4203,#4202,#2896,.T.);
#5539=EDGE_CURVE('',#4204,#4204,#2073,.T.);
#5540=EDGE_CURVE('',#4205,#4206,#2433,.F.);
#5541=EDGE_CURVE('',#4207,#4206,#2434,.T.);
#5542=EDGE_CURVE('',#4207,#4208,#2435,.T.);
#5543=EDGE_CURVE('',#4209,#4208,#2436,.T.);
#5544=EDGE_CURVE('',#4209,#4210,#2437,.T.);
#5545=EDGE_CURVE('',#4211,#4210,#2438,.T.);
#5546=EDGE_CURVE('',#4211,#4212,#2439,.T.);
#5547=EDGE_CURVE('',#4213,#4212,#2440,.T.);
#5548=EDGE_CURVE('',#4213,#4214,#2441,.T.);
#5549=EDGE_CURVE('',#4215,#4214,#2442,.T.);
#5550=EDGE_CURVE('',#4215,#4204,#64,.T.);
#5551=EDGE_CURVE('',#4216,#4215,#2443,.T.);
#5552=EDGE_CURVE('',#4216,#4217,#2444,.T.);
#5553=EDGE_CURVE('',#4205,#4217,#2445,.T.);
#5554=EDGE_CURVE('',#4218,#4219,#2074,.T.);
#5555=EDGE_CURVE('',#4206,#4218,#2897,.T.);
#5556=EDGE_CURVE('',#4205,#4219,#2898,.T.);
#5557=EDGE_CURVE('',#4220,#4219,#2899,.T.);
#5558=EDGE_CURVE('',#4220,#4221,#2075,.T.);
#5559=EDGE_CURVE('',#4222,#4221,#2900,.T.);
#5560=EDGE_CURVE('',#4222,#4223,#2076,.T.);
#5561=EDGE_CURVE('',#4224,#4223,#2901,.T.);
#5562=EDGE_CURVE('',#4224,#4225,#2077,.T.);
#5563=EDGE_CURVE('',#4226,#4225,#2902,.T.);
#5564=EDGE_CURVE('',#4226,#4227,#2078,.T.);
#5565=EDGE_CURVE('',#4228,#4227,#2903,.T.);
#5566=EDGE_CURVE('',#4228,#4229,#2079,.T.);
#5567=EDGE_CURVE('',#4218,#4229,#2904,.T.);
#5568=EDGE_CURVE('',#4230,#4230,#2080,.T.);
#5569=EDGE_CURVE('',#4230,#4231,#2905,.T.);
#5570=EDGE_CURVE('',#4231,#4232,#2446,.T.);
#5571=EDGE_CURVE('',#4232,#4233,#2906,.T.);
#5572=EDGE_CURVE('',#4233,#4231,#2447,.T.);
#5573=EDGE_CURVE('',#4234,#4232,#2448,.T.);
#5574=EDGE_CURVE('',#4235,#4234,#2449,.T.);
#5575=EDGE_CURVE('',#4233,#4235,#2450,.T.);
#5576=EDGE_CURVE('',#4236,#4237,#2451,.T.);
#5577=EDGE_CURVE('',#4237,#4233,#2452,.T.);
#5578=EDGE_CURVE('',#4238,#4235,#2453,.T.);
#5579=EDGE_CURVE('',#4236,#4238,#2907,.T.);
#5580=EDGE_CURVE('',#4239,#4236,#2454,.F.);
#5581=EDGE_CURVE('',#4240,#4239,#2908,.T.);
#5582=EDGE_CURVE('',#4240,#4241,#2455,.T.);
#5583=EDGE_CURVE('',#4241,#4237,#2909,.T.);
#5584=EDGE_CURVE('',#4242,#4239,#2456,.T.);
#5585=EDGE_CURVE('',#4243,#4238,#2457,.T.);
#5586=EDGE_CURVE('',#4242,#4243,#2910,.T.);
#5587=EDGE_CURVE('',#4199,#4240,#2458,.T.);
#5588=EDGE_CURVE('',#4201,#4242,#2459,.F.);
#5589=EDGE_CURVE('',#4198,#4243,#2460,.T.);
#5590=EDGE_CURVE('',#4243,#4240,#2911,.T.);
#5591=EDGE_CURVE('',#4238,#4241,#2912,.T.);
#5592=EDGE_CURVE('',#4241,#4234,#2461,.T.);
#5593=EDGE_CURVE('',#4207,#4229,#2913,.T.);
#5594=EDGE_CURVE('',#4208,#4228,#2914,.T.);
#5595=EDGE_CURVE('',#4209,#4227,#2915,.T.);
#5596=EDGE_CURVE('',#4210,#4226,#2916,.T.);
#5597=EDGE_CURVE('',#4211,#4225,#2917,.T.);
#5598=EDGE_CURVE('',#4212,#4224,#2918,.T.);
#5599=EDGE_CURVE('',#4217,#4220,#2919,.T.);
#5600=EDGE_CURVE('',#4216,#4221,#2920,.T.);
#5601=EDGE_CURVE('',#4214,#4222,#2921,.T.);
#5602=EDGE_CURVE('',#4213,#4223,#2922,.T.);
#8170=ORIENTED_EDGE('',*,*,#5531,.F.);
#8171=ORIENTED_EDGE('',*,*,#5532,.T.);
#8172=ORIENTED_EDGE('',*,*,#5533,.F.);
#8173=ORIENTED_EDGE('',*,*,#5534,.T.);
#8174=ORIENTED_EDGE('',*,*,#5535,.T.);
#8175=ORIENTED_EDGE('',*,*,#5536,.F.);
#8176=ORIENTED_EDGE('',*,*,#5537,.F.);
#8177=ORIENTED_EDGE('',*,*,#5538,.T.);
#8178=ORIENTED_EDGE('',*,*,#5536,.T.);
#8179=ORIENTED_EDGE('',*,*,#5538,.F.);
#8180=ORIENTED_EDGE('',*,*,#5539,.T.);
#8181=ORIENTED_EDGE('',*,*,#5537,.T.);
#8182=ORIENTED_EDGE('',*,*,#5540,.T.);
#8183=ORIENTED_EDGE('',*,*,#5541,.F.);
#8184=ORIENTED_EDGE('',*,*,#5542,.T.);
#8185=ORIENTED_EDGE('',*,*,#5543,.F.);
#8186=ORIENTED_EDGE('',*,*,#5544,.T.);
#8187=ORIENTED_EDGE('',*,*,#5545,.F.);
#8188=ORIENTED_EDGE('',*,*,#5546,.T.);
#8189=ORIENTED_EDGE('',*,*,#5547,.F.);
#8190=ORIENTED_EDGE('',*,*,#5548,.T.);
#8191=ORIENTED_EDGE('',*,*,#5549,.F.);
#8192=ORIENTED_EDGE('',*,*,#5550,.T.);
#8193=ORIENTED_EDGE('',*,*,#5539,.F.);
#8194=ORIENTED_EDGE('',*,*,#5550,.F.);
#8195=ORIENTED_EDGE('',*,*,#5551,.F.);
#8196=ORIENTED_EDGE('',*,*,#5552,.T.);
#8197=ORIENTED_EDGE('',*,*,#5553,.F.);
#8198=ORIENTED_EDGE('',*,*,#5554,.F.);
#8199=ORIENTED_EDGE('',*,*,#5555,.F.);
#8200=ORIENTED_EDGE('',*,*,#5540,.F.);
#8201=ORIENTED_EDGE('',*,*,#5556,.T.);
#8202=ORIENTED_EDGE('',*,*,#5554,.T.);
#8203=ORIENTED_EDGE('',*,*,#5557,.F.);
#8204=ORIENTED_EDGE('',*,*,#5558,.T.);
#8205=ORIENTED_EDGE('',*,*,#5559,.F.);
#8206=ORIENTED_EDGE('',*,*,#5560,.T.);
#8207=ORIENTED_EDGE('',*,*,#5561,.F.);
#8208=ORIENTED_EDGE('',*,*,#5562,.T.);
#8209=ORIENTED_EDGE('',*,*,#5563,.F.);
#8210=ORIENTED_EDGE('',*,*,#5564,.T.);
#8211=ORIENTED_EDGE('',*,*,#5565,.F.);
#8212=ORIENTED_EDGE('',*,*,#5566,.T.);
#8213=ORIENTED_EDGE('',*,*,#5567,.F.);
#8214=ORIENTED_EDGE('',*,*,#5568,.T.);
#8215=ORIENTED_EDGE('',*,*,#5568,.F.);
#8216=ORIENTED_EDGE('',*,*,#5569,.T.);
#8217=ORIENTED_EDGE('',*,*,#5570,.T.);
#8218=ORIENTED_EDGE('',*,*,#5571,.T.);
#8219=ORIENTED_EDGE('',*,*,#5572,.T.);
#8220=ORIENTED_EDGE('',*,*,#5569,.F.);
#8221=ORIENTED_EDGE('',*,*,#5571,.F.);
#8222=ORIENTED_EDGE('',*,*,#5573,.F.);
#8223=ORIENTED_EDGE('',*,*,#5574,.F.);
#8224=ORIENTED_EDGE('',*,*,#5575,.F.);
#8225=ORIENTED_EDGE('',*,*,#5576,.T.);
#8226=ORIENTED_EDGE('',*,*,#5577,.T.);
#8227=ORIENTED_EDGE('',*,*,#5575,.T.);
#8228=ORIENTED_EDGE('',*,*,#5578,.F.);
#8229=ORIENTED_EDGE('',*,*,#5579,.F.);
#8230=ORIENTED_EDGE('',*,*,#5580,.F.);
#8231=ORIENTED_EDGE('',*,*,#5581,.F.);
#8232=ORIENTED_EDGE('',*,*,#5582,.T.);
#8233=ORIENTED_EDGE('',*,*,#5583,.T.);
#8234=ORIENTED_EDGE('',*,*,#5576,.F.);
#8235=ORIENTED_EDGE('',*,*,#5584,.T.);
#8236=ORIENTED_EDGE('',*,*,#5580,.T.);
#8237=ORIENTED_EDGE('',*,*,#5579,.T.);
#8238=ORIENTED_EDGE('',*,*,#5585,.F.);
#8239=ORIENTED_EDGE('',*,*,#5586,.F.);
#8240=ORIENTED_EDGE('',*,*,#5534,.F.);
#8241=ORIENTED_EDGE('',*,*,#5533,.T.);
#8242=ORIENTED_EDGE('',*,*,#5587,.T.);
#8243=ORIENTED_EDGE('',*,*,#5581,.T.);
#8244=ORIENTED_EDGE('',*,*,#5584,.F.);
#8245=ORIENTED_EDGE('',*,*,#5588,.F.);
#8246=ORIENTED_EDGE('',*,*,#5589,.F.);
#8247=ORIENTED_EDGE('',*,*,#5535,.F.);
#8248=ORIENTED_EDGE('',*,*,#5588,.T.);
#8249=ORIENTED_EDGE('',*,*,#5586,.T.);
#8250=ORIENTED_EDGE('',*,*,#5587,.F.);
#8251=ORIENTED_EDGE('',*,*,#5532,.F.);
#8252=ORIENTED_EDGE('',*,*,#5531,.T.);
#8253=ORIENTED_EDGE('',*,*,#5589,.T.);
#8254=ORIENTED_EDGE('',*,*,#5590,.T.);
#8255=ORIENTED_EDGE('',*,*,#5590,.F.);
#8256=ORIENTED_EDGE('',*,*,#5585,.T.);
#8257=ORIENTED_EDGE('',*,*,#5591,.T.);
#8258=ORIENTED_EDGE('',*,*,#5582,.F.);
#8259=ORIENTED_EDGE('',*,*,#5591,.F.);
#8260=ORIENTED_EDGE('',*,*,#5578,.T.);
#8261=ORIENTED_EDGE('',*,*,#5574,.T.);
#8262=ORIENTED_EDGE('',*,*,#5592,.F.);
#8263=ORIENTED_EDGE('',*,*,#5577,.F.);
#8264=ORIENTED_EDGE('',*,*,#5583,.F.);
#8265=ORIENTED_EDGE('',*,*,#5592,.T.);
#8266=ORIENTED_EDGE('',*,*,#5573,.T.);
#8267=ORIENTED_EDGE('',*,*,#5570,.F.);
#8268=ORIENTED_EDGE('',*,*,#5572,.F.);
#8269=ORIENTED_EDGE('',*,*,#5555,.T.);
#8270=ORIENTED_EDGE('',*,*,#5567,.T.);
#8271=ORIENTED_EDGE('',*,*,#5593,.F.);
#8272=ORIENTED_EDGE('',*,*,#5541,.T.);
#8273=ORIENTED_EDGE('',*,*,#5566,.F.);
#8274=ORIENTED_EDGE('',*,*,#5594,.F.);
#8275=ORIENTED_EDGE('',*,*,#5542,.F.);
#8276=ORIENTED_EDGE('',*,*,#5593,.T.);
#8277=ORIENTED_EDGE('',*,*,#5594,.T.);
#8278=ORIENTED_EDGE('',*,*,#5565,.T.);
#8279=ORIENTED_EDGE('',*,*,#5595,.F.);
#8280=ORIENTED_EDGE('',*,*,#5543,.T.);
#8281=ORIENTED_EDGE('',*,*,#5564,.F.);
#8282=ORIENTED_EDGE('',*,*,#5596,.F.);
#8283=ORIENTED_EDGE('',*,*,#5544,.F.);
#8284=ORIENTED_EDGE('',*,*,#5595,.T.);
#8285=ORIENTED_EDGE('',*,*,#5596,.T.);
#8286=ORIENTED_EDGE('',*,*,#5563,.T.);
#8287=ORIENTED_EDGE('',*,*,#5597,.F.);
#8288=ORIENTED_EDGE('',*,*,#5545,.T.);
#8289=ORIENTED_EDGE('',*,*,#5562,.F.);
#8290=ORIENTED_EDGE('',*,*,#5598,.F.);
#8291=ORIENTED_EDGE('',*,*,#5546,.F.);
#8292=ORIENTED_EDGE('',*,*,#5597,.T.);
#8293=ORIENTED_EDGE('',*,*,#5556,.F.);
#8294=ORIENTED_EDGE('',*,*,#5553,.T.);
#8295=ORIENTED_EDGE('',*,*,#5599,.T.);
#8296=ORIENTED_EDGE('',*,*,#5557,.T.);
#8297=ORIENTED_EDGE('',*,*,#5558,.F.);
#8298=ORIENTED_EDGE('',*,*,#5599,.F.);
#8299=ORIENTED_EDGE('',*,*,#5552,.F.);
#8300=ORIENTED_EDGE('',*,*,#5600,.T.);
#8301=ORIENTED_EDGE('',*,*,#5601,.T.);
#8302=ORIENTED_EDGE('',*,*,#5559,.T.);
#8303=ORIENTED_EDGE('',*,*,#5600,.F.);
#8304=ORIENTED_EDGE('',*,*,#5551,.T.);
#8305=ORIENTED_EDGE('',*,*,#5549,.T.);
#8306=ORIENTED_EDGE('',*,*,#5560,.F.);
#8307=ORIENTED_EDGE('',*,*,#5601,.F.);
#8308=ORIENTED_EDGE('',*,*,#5548,.F.);
#8309=ORIENTED_EDGE('',*,*,#5602,.T.);
#8310=ORIENTED_EDGE('',*,*,#5598,.T.);
#8311=ORIENTED_EDGE('',*,*,#5561,.T.);
#8312=ORIENTED_EDGE('',*,*,#5602,.F.);
#8313=ORIENTED_EDGE('',*,*,#5547,.T.);
#8569=CYLINDRICAL_SURFACE('',#10145,3.125);
#8570=CYLINDRICAL_SURFACE('',#10149,1.);
#8571=CYLINDRICAL_SURFACE('',#10158,4.);
#8572=CYLINDRICAL_SURFACE('',#10161,1.);
#8573=CYLINDRICAL_SURFACE('',#10163,1.);
#8574=CYLINDRICAL_SURFACE('',#10165,1.);
#8575=CYLINDRICAL_SURFACE('',#10167,1.);
#8576=CYLINDRICAL_SURFACE('',#10169,1.);
#9080=ADVANCED_FACE('',(#1017,#317),#505,.F.);
#9081=ADVANCED_FACE('',(#1018),#8569,.F.);
#9082=ADVANCED_FACE('',(#1019,#318),#506,.T.);
#9083=ADVANCED_FACE('',(#1020),#198,.F.);
#9084=ADVANCED_FACE('',(#1021),#8570,.T.);
#9085=ADVANCED_FACE('',(#1022,#319),#507,.F.);
#9086=ADVANCED_FACE('',(#1023),#8571,.T.);
#9087=ADVANCED_FACE('',(#1024),#508,.F.);
#9088=ADVANCED_FACE('',(#1025),#400,.F.);
#9089=ADVANCED_FACE('',(#1026),#401,.F.);
#9090=ADVANCED_FACE('',(#1027),#402,.F.);
#9091=ADVANCED_FACE('',(#1028),#403,.F.);
#9092=ADVANCED_FACE('',(#1029),#404,.F.);
#9093=ADVANCED_FACE('',(#1030),#405,.F.);
#9094=ADVANCED_FACE('',(#1031),#406,.F.);
#9095=ADVANCED_FACE('',(#1032),#407,.F.);
#9096=ADVANCED_FACE('',(#1033),#408,.F.);
#9097=ADVANCED_FACE('',(#1034),#509,.T.);
#9098=ADVANCED_FACE('',(#1035),#8572,.T.);
#9099=ADVANCED_FACE('',(#1036),#510,.T.);
#9100=ADVANCED_FACE('',(#1037),#8573,.T.);
#9101=ADVANCED_FACE('',(#1038),#511,.T.);
#9102=ADVANCED_FACE('',(#1039),#8574,.T.);
#9103=ADVANCED_FACE('',(#1040),#512,.T.);
#9104=ADVANCED_FACE('',(#1041),#8575,.T.);
#9105=ADVANCED_FACE('',(#1042),#513,.T.);
#9106=ADVANCED_FACE('',(#1043),#8576,.T.);
#9107=ADVANCED_FACE('',(#1044),#514,.T.);
#9127=CLOSED_SHELL('',(#9080,#9081,#9082,#9083,#9084,#9085,#9086,#9087,
#9088,#9089,#9090,#9091,#9092,#9093,#9094,#9095,#9096,#9097,#9098,#9099,
#9100,#9101,#9102,#9103,#9104,#9105,#9106,#9107));
#10142=AXIS2_PLACEMENT_3D('',#46062,#12378,#12379);
#10143=AXIS2_PLACEMENT_3D('',#46063,#12380,#12381);
#10144=AXIS2_PLACEMENT_3D('',#46202,#12382,#12383);
#10145=AXIS2_PLACEMENT_3D('',#46203,#12384,#12385);
#10146=AXIS2_PLACEMENT_3D('',#46205,#12386,#12387);
#10147=AXIS2_PLACEMENT_3D('',#46207,#12389,#12390);
#10148=AXIS2_PLACEMENT_3D('',#46209,#12391,#12392);
#10149=AXIS2_PLACEMENT_3D('',#46380,#12393,#12394);
#10150=AXIS2_PLACEMENT_3D('',#46383,#12395,#12396);
#10151=AXIS2_PLACEMENT_3D('',#46386,#12399,#12400);
#10152=AXIS2_PLACEMENT_3D('',#46390,#12402,#12403);
#10153=AXIS2_PLACEMENT_3D('',#46394,#12405,#12406);
#10154=AXIS2_PLACEMENT_3D('',#46398,#12408,#12409);
#10155=AXIS2_PLACEMENT_3D('',#46402,#12411,#12412);
#10156=AXIS2_PLACEMENT_3D('',#46406,#12414,#12415);
#10157=AXIS2_PLACEMENT_3D('',#46409,#12417,#12418);
#10158=AXIS2_PLACEMENT_3D('',#46410,#12419,#12420);
#10159=AXIS2_PLACEMENT_3D('',#46488,#12423,#12424);
#10160=AXIS2_PLACEMENT_3D('',#52059,#12431,#12432);
#10161=AXIS2_PLACEMENT_3D('',#52061,#12434,#12435);
#10162=AXIS2_PLACEMENT_3D('',#52063,#12437,#12438);
#10163=AXIS2_PLACEMENT_3D('',#52065,#12440,#12441);
#10164=AXIS2_PLACEMENT_3D('',#52067,#12443,#12444);
#10165=AXIS2_PLACEMENT_3D('',#52069,#12446,#12447);
#10166=AXIS2_PLACEMENT_3D('',#52071,#12449,#12450);
#10167=AXIS2_PLACEMENT_3D('',#52073,#12452,#12453);
#10168=AXIS2_PLACEMENT_3D('',#52075,#12455,#12456);
#10169=AXIS2_PLACEMENT_3D('',#52077,#12458,#12459);
#10170=AXIS2_PLACEMENT_3D('',#52079,#12461,#12462);
#12378=DIRECTION('axis',(0.,0.,1.));
#12379=DIRECTION('refdir',(1.,0.,0.));
#12380=DIRECTION('center_axis',(0.,0.,-1.));
#12381=DIRECTION('ref_axis',(0.,-1.,0.));
#12382=DIRECTION('center_axis',(0.,0.,1.));
#12383=DIRECTION('ref_axis',(0.,-1.,0.));
#12384=DIRECTION('center_axis',(0.,0.,1.));
#12385=DIRECTION('ref_axis',(0.,-1.,0.));
#12386=DIRECTION('center_axis',(0.,0.,1.));
#12387=DIRECTION('ref_axis',(0.,-1.,0.));
#12388=DIRECTION('',(0.,0.,1.));
#12389=DIRECTION('center_axis',(0.,0.,-1.));
#12390=DIRECTION('ref_axis',(0.,-1.,0.));
#12391=DIRECTION('center_axis',(0.,0.,-1.));
#12392=DIRECTION('ref_axis',(0.,1.,0.));
#12393=DIRECTION('center_axis',(0.,0.,1.));
#12394=DIRECTION('ref_axis',(0.500000000000017,0.866025403784429,0.));
#12395=DIRECTION('center_axis',(0.,0.,1.));
#12396=DIRECTION('ref_axis',(0.500000000000017,0.866025403784429,0.));
#12397=DIRECTION('',(0.,0.,1.));
#12398=DIRECTION('',(0.,0.,1.));
#12399=DIRECTION('center_axis',(0.,0.,-1.));
#12400=DIRECTION('ref_axis',(0.,-1.,0.));
#12401=DIRECTION('',(0.866025403784429,0.500000000000017,0.));
#12402=DIRECTION('center_axis',(0.,0.,1.));
#12403=DIRECTION('ref_axis',(-0.500000000000017,0.866025403784429,0.));
#12404=DIRECTION('',(0.,1.,0.));
#12405=DIRECTION('center_axis',(0.,0.,1.));
#12406=DIRECTION('ref_axis',(-1.,0.,0.));
#12407=DIRECTION('',(-0.866025403784429,0.500000000000017,0.));
#12408=DIRECTION('center_axis',(0.,0.,1.));
#12409=DIRECTION('ref_axis',(-0.500000000000017,-0.866025403784429,0.));
#12410=DIRECTION('',(-0.866025403784429,-0.500000000000017,0.));
#12411=DIRECTION('center_axis',(0.,0.,1.));
#12412=DIRECTION('ref_axis',(0.500000000000017,-0.866025403784429,0.));
#12413=DIRECTION('',(0.,-1.,0.));
#12414=DIRECTION('center_axis',(0.,0.,1.));
#12415=DIRECTION('ref_axis',(1.,0.,0.));
#12416=DIRECTION('',(0.866025403784429,-0.500000000000017,0.));
#12417=DIRECTION('center_axis',(0.,0.,-1.));
#12418=DIRECTION('ref_axis',(0.,-1.,0.));
#12419=DIRECTION('center_axis',(0.,0.,-1.));
#12420=DIRECTION('ref_axis',(0.,-1.,0.));
#12421=DIRECTION('',(0.,0.,1.));
#12422=DIRECTION('',(0.,0.,1.));
#12423=DIRECTION('center_axis',(-0.500000000000017,-0.866025403784429,0.));
#12424=DIRECTION('ref_axis',(-0.866025403784429,0.500000000000017,0.));
#12425=DIRECTION('',(0.296198132725996,0.813797681349388,-0.499999999999993));
#12426=DIRECTION('',(-0.852868531952436,0.150383733180406,-0.500000000000021));
#12427=DIRECTION('',(-0.296198132725996,-0.813797681349388,-0.499999999999993));
#12428=DIRECTION('',(0.852868531952436,-0.150383733180406,-0.500000000000021));
#12429=DIRECTION('',(0.,0.,-1.));
#12430=DIRECTION('',(0.,0.,-1.));
#12431=DIRECTION('center_axis',(0.500000000000017,0.866025403784429,0.));
#12432=DIRECTION('ref_axis',(0.866025403784429,-0.500000000000017,0.));
#12433=DIRECTION('',(0.,0.,1.));
#12434=DIRECTION('center_axis',(0.,0.,1.));
#12435=DIRECTION('ref_axis',(1.,0.,0.));
#12436=DIRECTION('',(0.,0.,1.));
#12437=DIRECTION('center_axis',(1.,0.,0.));
#12438=DIRECTION('ref_axis',(0.,-1.,0.));
#12439=DIRECTION('',(0.,0.,1.));
#12440=DIRECTION('center_axis',(0.,0.,1.));
#12441=DIRECTION('ref_axis',(0.500000000000017,-0.866025403784429,0.));
#12442=DIRECTION('',(0.,0.,1.));
#12443=DIRECTION('center_axis',(0.500000000000017,-0.866025403784429,0.));
#12444=DIRECTION('ref_axis',(-0.866025403784429,-0.500000000000017,0.));
#12445=DIRECTION('',(0.,0.,1.));
#12446=DIRECTION('center_axis',(0.,0.,1.));
#12447=DIRECTION('ref_axis',(-0.500000000000017,-0.866025403784429,0.));
#12448=DIRECTION('',(0.,0.,1.));
#12449=DIRECTION('center_axis',(-0.500000000000017,0.866025403784429,0.));
#12450=DIRECTION('ref_axis',(0.866025403784429,0.500000000000017,0.));
#12451=DIRECTION('',(0.,0.,1.));
#12452=DIRECTION('center_axis',(0.,0.,1.));
#12453=DIRECTION('ref_axis',(-0.500000000000017,0.866025403784429,0.));
#12454=DIRECTION('',(0.,0.,1.));
#12455=DIRECTION('center_axis',(-1.,0.,0.));
#12456=DIRECTION('ref_axis',(0.,1.,0.));
#12457=DIRECTION('',(0.,2.221133174104E-14,1.));
#12458=DIRECTION('center_axis',(0.,0.,1.));
#12459=DIRECTION('ref_axis',(-1.,0.,0.));
#12460=DIRECTION('',(0.,0.,1.));
#12461=DIRECTION('center_axis',(-0.500000000000017,-0.866025403784429,0.));
#12462=DIRECTION('ref_axis',(-0.866025403784429,0.500000000000017,0.));
#46062=CARTESIAN_POINT('',(0.,0.,0.));
#46063=CARTESIAN_POINT('Origin',(0.,0.,0.));
#46064=CARTESIAN_POINT('',(3.48003877702181,-0.646332386289707,7.2890636783777E-5));
#46065=CARTESIAN_POINT('',(3.47936545704605,-0.650670105535317,-4.76018332824096E-10));
#46066=CARTESIAN_POINT('Ctrl Pts',(3.4800387770396,-0.646332386169619,7.2890641512717E-5));
#46067=CARTESIAN_POINT('Ctrl Pts',(3.47981522939477,-0.647778405716227,
4.85936023357466E-5));
#46068=CARTESIAN_POINT('Ctrl Pts',(3.47959078938191,-0.649224312550689,
2.42965631587873E-5));
#46069=CARTESIAN_POINT('Ctrl Pts',(3.47936545704605,-0.650670105535317,
-4.76018183204197E-10));
#46070=CARTESIAN_POINT('',(-0.264621262814254,3.52921885147511,9.97465998686664E-17));
#46071=CARTESIAN_POINT('Ctrl Pts',(3.48016653829928,-0.646334509992552,
-5.89805981832114E-17));
#46072=CARTESIAN_POINT('Ctrl Pts',(3.49317607817561,-0.575677005108545,
-4.47285692339558E-17));
#46073=CARTESIAN_POINT('Ctrl Pts',(3.50395521937367,-0.50501662146249,-2.70647475776074E-16));
#46074=CARTESIAN_POINT('Ctrl Pts',(3.51259146904678,-0.434285235184753,
-9.71445146547012E-17));
#46075=CARTESIAN_POINT('Ctrl Pts',(3.52000759887453,-0.373546701285584,
5.18461391449629E-17));
#46076=CARTESIAN_POINT('Ctrl Pts',(3.5258427031227,-0.312755312469289,3.08838204074247E-17));
#46077=CARTESIAN_POINT('Ctrl Pts',(3.53012221027278,-0.251861352637095,
6.93889390390723E-18));
#46078=CARTESIAN_POINT('Ctrl Pts',(3.53326008626827,-0.207211889947475,
-1.06183171145701E-17));
#46079=CARTESIAN_POINT('Ctrl Pts',(3.53556105447104,-0.162507144984163,
-9.16607259699049E-18));
#46080=CARTESIAN_POINT('Ctrl Pts',(3.53702575001128,-0.11772666792086,-4.85722573273506E-17));
#46081=CARTESIAN_POINT('Ctrl Pts',(3.53979104880602,-0.0331825453716335,
-1.22969886149647E-16));
#46082=CARTESIAN_POINT('Ctrl Pts',(3.53956910994069,0.0516350306695476,
-6.18610164700975E-17));
#46083=CARTESIAN_POINT('Ctrl Pts',(3.53634427120997,0.136328894393368,-1.31838984174237E-16));
#46084=CARTESIAN_POINT('Ctrl Pts',(3.53350080053847,0.211006897749522,-1.93541387126446E-16));
#46085=CARTESIAN_POINT('Ctrl Pts',(3.52832339789583,0.285588347755748,-7.27345771358064E-17));
#46086=CARTESIAN_POINT('Ctrl Pts',(3.52083348352867,0.359802147884021,-1.31838984174237E-16));
#46087=CARTESIAN_POINT('Ctrl Pts',(3.51700351154709,0.397751416888196,-1.620620564082E-16));
#46088=CARTESIAN_POINT('Ctrl Pts',(3.5125699817729,0.435600311646885,2.2803504033583E-16));
#46089=CARTESIAN_POINT('Ctrl Pts',(3.5075361770783,0.473331412925596,1.87350135405495E-16));
#46090=CARTESIAN_POINT('Ctrl Pts',(3.49608873487737,0.559136212132028,9.48280520320672E-17));
#46091=CARTESIAN_POINT('Ctrl Pts',(3.48153875813074,0.644349892122457,9.44312770845489E-18));
#46092=CARTESIAN_POINT('Ctrl Pts',(3.46387334496763,0.72891602679703,-5.55111512312578E-17));
#46093=CARTESIAN_POINT('Ctrl Pts',(3.45224750382509,0.784570114176018,-9.82584179670611E-17));
#46094=CARTESIAN_POINT('Ctrl Pts',(3.43927126982642,0.839943685437852,2.39787204036035E-17));
#46095=CARTESIAN_POINT('Ctrl Pts',(3.42492877103772,0.895018163495264,-4.16333634234434E-17));
#46096=CARTESIAN_POINT('Ctrl Pts',(3.41442478500919,0.935352944523725,-8.96855488881198E-17));
#46097=CARTESIAN_POINT('Ctrl Pts',(3.40318658623661,0.975530746433315,1.11794948779964E-16));
#46098=CARTESIAN_POINT('Ctrl Pts',(3.39121177775683,1.0155208901864,1.2490009027033E-16));
#46099=CARTESIAN_POINT('Ctrl Pts',(3.36752469815931,1.09462442823421,1.80738876930359E-16));
#46100=CARTESIAN_POINT('Ctrl Pts',(3.34095533515231,1.17299052953756,-1.19499472761792E-16));
#46101=CARTESIAN_POINT('Ctrl Pts',(3.3116102147096,1.2503974394701,-1.2490009027033E-16));
#46102=CARTESIAN_POINT('Ctrl Pts',(3.28815858462756,1.31225842999066,-1.29216081553176E-16));
#46103=CARTESIAN_POINT('Ctrl Pts',(3.2629344689088,1.37350678139125,3.39993763381456E-16));
#46104=CARTESIAN_POINT('Ctrl Pts',(3.23599822549168,1.43403048862511,2.77555756156289E-16));
#46105=CARTESIAN_POINT('Ctrl Pts',(3.20059471381763,1.51357950897026,1.95490685557198E-16));
#46106=CARTESIAN_POINT('Ctrl Pts',(3.16223650327715,1.59188240530522,1.34206159441388E-16));
#46107=CARTESIAN_POINT('Ctrl Pts',(3.12094944371241,1.66888339837784,9.71445146547012E-17));
#46108=CARTESIAN_POINT('Ctrl Pts',(3.08975243467893,1.72706629398237,6.91402808973229E-17));
#46109=CARTESIAN_POINT('Ctrl Pts',(3.0568822049507,1.78450547174452,-3.62912008896638E-17));
#46110=CARTESIAN_POINT('Ctrl Pts',(3.02233378145072,1.84116537654111,0.));
#46111=CARTESIAN_POINT('Ctrl Pts',(2.99901028957703,1.87941623418409,2.45000333817547E-17));
#46112=CARTESIAN_POINT('Ctrl Pts',(2.974919809587,1.91731447029493,2.10095953603969E-16));
#46113=CARTESIAN_POINT('Ctrl Pts',(2.95006469153859,1.95483542786409,2.08166817117217E-16));
#46114=CARTESIAN_POINT('Ctrl Pts',(2.88489660607661,2.05321230801891,2.03108779123126E-16));
#46115=CARTESIAN_POINT('Ctrl Pts',(2.8144819340267,2.14897369239657,-2.965152410952E-17));
#46116=CARTESIAN_POINT('Ctrl Pts',(2.73904724714154,2.24141498451818,-8.32667268468867E-17));
#46117=CARTESIAN_POINT('Ctrl Pts',(2.70229826855952,2.28644894972098,-1.0938606290333E-16));
#46118=CARTESIAN_POINT('Ctrl Pts',(2.66435761337232,2.33069592454894,-3.5640658198706E-17));
#46119=CARTESIAN_POINT('Ctrl Pts',(2.62525892065778,2.37406997285321,-2.77555756156289E-17));
#46120=CARTESIAN_POINT('Ctrl Pts',(2.5707368279943,2.4345539357852,-1.67600365475454E-17));
#46121=CARTESIAN_POINT('Ctrl Pts',(2.51397031226346,2.49332645267094,5.10850161412582E-17));
#46122=CARTESIAN_POINT('Ctrl Pts',(2.45517505526017,2.55006466651292,-8.32667268468867E-17));
#46123=CARTESIAN_POINT('Ctrl Pts',(2.40728457699653,2.5962796221949,-1.92700200824151E-16));
#46124=CARTESIAN_POINT('Ctrl Pts',(2.3580489717218,2.64114531836818,-2.20460030602934E-16));
#46125=CARTESIAN_POINT('Ctrl Pts',(2.30760323636819,2.68450503882998,-2.77555756156289E-16));
#46126=CARTESIAN_POINT('Ctrl Pts',(2.27865530387642,2.7093867112249,-3.38235922399021E-16));
#46127=CARTESIAN_POINT('Ctrl Pts',(2.24931159991021,2.73377088022847,1.71863076464404E-16));
#46128=CARTESIAN_POINT('Ctrl Pts',(2.21959827171105,2.75764646490264,1.38777878078145E-16));
#46129=CARTESIAN_POINT('Ctrl Pts',(2.14143730410158,2.82045123681735,5.17471993844663E-17));
#46130=CARTESIAN_POINT('Ctrl Pts',(2.06070142653763,2.87975713463521,-1.56650036923279E-16));
#46131=CARTESIAN_POINT('Ctrl Pts',(1.97762156218559,2.93552733768934,-1.11022302462516E-16));
#46132=CARTESIAN_POINT('Ctrl Pts',(1.92211983121906,2.97278477461466,-8.05405694649354E-17));
#46133=CARTESIAN_POINT('Ctrl Pts',(1.86557114727434,3.00846349169955,-2.42724910906657E-17));
#46134=CARTESIAN_POINT('Ctrl Pts',(1.80803658801739,3.0425422416155,0.));
#46135=CARTESIAN_POINT('Ctrl Pts',(1.7188400885876,3.09537492577444,3.76299265291851E-17));
#46136=CARTESIAN_POINT('Ctrl Pts',(1.62727618984203,3.14435347841968,-5.86239920736008E-20));
#46137=CARTESIAN_POINT('Ctrl Pts',(1.53385010392579,3.18924471308555,5.55111512312578E-17));
#46138=CARTESIAN_POINT('Ctrl Pts',(1.47764192286276,3.21625274431682,8.89437408206909E-17));
#46139=CARTESIAN_POINT('Ctrl Pts',(1.42076021590392,3.24178219173936,8.07486977161786E-17));
#46140=CARTESIAN_POINT('Ctrl Pts',(1.36331845320285,3.26579067475782,1.11022302462516E-16));
#46141=CARTESIAN_POINT('Ctrl Pts',(1.31009042500589,3.28803797621554,1.39075137391133E-16));
#46142=CARTESIAN_POINT('Ctrl Pts',(1.25638952610923,3.3089769997134,-7.7221606089057E-17));
#46143=CARTESIAN_POINT('Ctrl Pts',(1.20225233191348,3.32859739842768,-5.55111512312578E-17));
#46144=CARTESIAN_POINT('Ctrl Pts',(1.1142617813533,3.36048692855069,-2.0224600012103E-17));
#46145=CARTESIAN_POINT('Ctrl Pts',(1.02511436445074,3.38889779844708,-1.78457313905869E-17));
#46146=CARTESIAN_POINT('Ctrl Pts',(0.934925304373438,3.41375797748399,-5.55111512312578E-17));
#46147=CARTESIAN_POINT('Ctrl Pts',(0.885809238120318,3.42729658404664,-7.60233647387536E-17));
#46148=CARTESIAN_POINT('Ctrl Pts',(0.836383195275312,3.43978145529386,-2.05712469523657E-16));
#46149=CARTESIAN_POINT('Ctrl Pts',(0.786666628307869,3.4511940464116,-1.38777878078145E-16));
#46150=CARTESIAN_POINT('Ctrl Pts',(0.690297762049071,3.47331581656142,-9.03419132430871E-18));
#46151=CARTESIAN_POINT('Ctrl Pts',(0.59285483884902,3.49139795611778,8.42365090681754E-17));
#46152=CARTESIAN_POINT('Ctrl Pts',(0.494841798296601,3.50524344299471,1.11022302462516E-16));
#46153=CARTESIAN_POINT('Ctrl Pts',(0.432069322108475,3.51411078850706,1.28713363252148E-16));
#46154=CARTESIAN_POINT('Ctrl Pts',(0.369063375024884,3.52124159998704,1.271306364805E-16));
#46155=CARTESIAN_POINT('Ctrl Pts',(0.305964768744507,3.52664906588399,1.66533453693773E-16));
#46156=CARTESIAN_POINT('Ctrl Pts',(0.269285915132926,3.52979239442539,1.89438082649088E-16));
#46157=CARTESIAN_POINT('Ctrl Pts',(0.232581119446525,3.53235340649015,2.30811615431158E-17));
#46158=CARTESIAN_POINT('Ctrl Pts',(0.19585282992679,3.5343374073664,2.77555756156289E-17));
#46159=CARTESIAN_POINT('Ctrl Pts',(0.119441498428624,3.53846501991332,3.74804554813947E-17));
#46160=CARTESIAN_POINT('Ctrl Pts',(0.0429151096247929,3.54010034667225,
6.94070683690155E-17));
#46161=CARTESIAN_POINT('Ctrl Pts',(-0.0338049752335097,3.53925398805205,
1.38777878078145E-16));
#46162=CARTESIAN_POINT('Ctrl Pts',(-0.110525060091812,3.53840762943185,
2.08148687787274E-16));
#46163=CARTESIAN_POINT('Ctrl Pts',(-0.187439519225311,3.5350795447432,-4.39206313887317E-17));
#46164=CARTESIAN_POINT('Ctrl Pts',(-0.264621262814249,3.52921885147511,
-1.11022302462516E-16));
#46165=CARTESIAN_POINT('',(-0.278675535189408,3.52854398769841,0.000242178628510733));
#46166=CARTESIAN_POINT('Ctrl Pts',(-0.278642183567104,3.52812649287716,
0.000242178628510788));
#46167=CARTESIAN_POINT('Ctrl Pts',(-0.273969233930499,3.52849979200248,
0.000161453268946271));
#46168=CARTESIAN_POINT('Ctrl Pts',(-0.26929558191709,3.52886391325551,8.07279093816785E-5));
#46169=CARTESIAN_POINT('Ctrl Pts',(-0.264621264353401,3.52921885135824,
2.54981716296676E-9));
#46170=CARTESIAN_POINT('',(-2.97253954097099,-2.67651699463381,-6.72783956812026E-18));
#46171=CARTESIAN_POINT('Ctrl Pts',(-0.278697848415911,3.52896236434037,
2.38524477946811E-17));
#46172=CARTESIAN_POINT('Ctrl Pts',(-0.754955028066917,3.51933407567894,
2.38524477946811E-17));
#46173=CARTESIAN_POINT('Ctrl Pts',(-1.18674072769151,3.41430558451068,-1.24655644773836E-14));
#46174=CARTESIAN_POINT('Ctrl Pts',(-1.96733714971687,3.09598181816572,-1.24622173902629E-14));
#46175=CARTESIAN_POINT('Ctrl Pts',(-2.34699951566166,2.85180221342043,-2.1094237467878E-14));
#46176=CARTESIAN_POINT('Ctrl Pts',(-2.99020885234353,2.24735338315926,-2.1094237467878E-14));
#46177=CARTESIAN_POINT('Ctrl Pts',(-3.29244004341223,1.85806081342808,-4.6609974510937E-14));
#46178=CARTESIAN_POINT('Ctrl Pts',(-3.71972888834082,0.9162945088732,-4.66139109655266E-14));
#46179=CARTESIAN_POINT('Ctrl Pts',(-3.83362815108384,0.428864103968153,
-7.34116402883767E-14));
#46180=CARTESIAN_POINT('Ctrl Pts',(-3.86808345271407,-0.535129438249572,
-7.34152353651497E-14));
#46181=CARTESIAN_POINT('Ctrl Pts',(-3.79982816305649,-0.999034854858048,
-5.31172328344098E-14));
#46182=CARTESIAN_POINT('Ctrl Pts',(-3.48665287488867,-1.93562500296496,
-5.31172328344098E-14));
#46183=CARTESIAN_POINT('Ctrl Pts',(-3.23969235129666,-2.34687602292039,
-1.9992468236924E-17));
#46184=CARTESIAN_POINT('Ctrl Pts',(-2.97252122137584,-2.6765004993568,-1.9992468236924E-17));
#46185=CARTESIAN_POINT('Ctrl Pts',(-2.97255786056614,-2.67653348991082,
6.53678910068347E-18));
#46186=CARTESIAN_POINT('Ctrl Pts',(-2.66529278319453,-2.98406739191157,
6.53678910068347E-18));
#46187=CARTESIAN_POINT('Ctrl Pts',(-2.30678228389453,-3.24050676320864,
3.24897772374216E-14));
#46188=CARTESIAN_POINT('Ctrl Pts',(-1.53166232714772,-3.62228294569805,
3.24929449932003E-14));
#46189=CARTESIAN_POINT('Ctrl Pts',(-1.12143089614916,-3.74638918522431,
3.97756064862856E-14));
#46190=CARTESIAN_POINT('Ctrl Pts',(-0.259412793720378,-3.85602623074799,
3.97788478927697E-14));
#46191=CARTESIAN_POINT('Ctrl Pts',(0.239543577753453,-3.84465005200125,
4.68007943103259E-14));
#46192=CARTESIAN_POINT('Ctrl Pts',(1.22159631150557,-3.5865596742176,4.68046624085105E-14));
#46193=CARTESIAN_POINT('Ctrl Pts',(1.66110604070138,-3.37568430365941,3.39640246886428E-14));
#46194=CARTESIAN_POINT('Ctrl Pts',(2.54221189401124,-2.72072246706673,3.3968295615247E-14));
#46195=CARTESIAN_POINT('Ctrl Pts',(2.83181469633017,-2.31316909850315,2.74445762896468E-14));
#46196=CARTESIAN_POINT('Ctrl Pts',(3.1232636873208,-1.82954859920293,2.74423321302002E-14));
#46197=CARTESIAN_POINT('Ctrl Pts',(3.23034582646799,-1.60226308336958,2.94209101525666E-14));
#46198=CARTESIAN_POINT('Ctrl Pts',(3.39277224036371,-1.13390966780497,2.94209101525666E-14));
#46199=CARTESIAN_POINT('Ctrl Pts',(3.44860799855318,-0.893678441777806,
-3.9176209116266E-18));
#46200=CARTESIAN_POINT('Ctrl Pts',(3.47936545786246,-0.65067010563865,-3.9176209116266E-18));
#46201=CARTESIAN_POINT('',(-3.82702124733548E-16,3.125,0.));
#46202=CARTESIAN_POINT('Origin',(0.,0.,0.));
#46203=CARTESIAN_POINT('Origin',(0.,0.,0.));
#46204=CARTESIAN_POINT('',(-3.82702124733548E-16,3.125,-12.2));
#46205=CARTESIAN_POINT('Origin',(0.,0.,-12.2));
#46206=CARTESIAN_POINT('',(-3.82702124733548E-16,3.125,0.));
#46207=CARTESIAN_POINT('Origin',(0.,0.,-12.2));
#46208=CARTESIAN_POINT('',(-3.5,3.32700602805782E-12,-12.2));
#46209=CARTESIAN_POINT('Origin',(0.,0.,-12.2));
#46210=CARTESIAN_POINT('Ctrl Pts',(-3.49999999998833,3.32743465443771E-12,
-12.2000000000021));
#46211=CARTESIAN_POINT('Ctrl Pts',(-3.49999999998833,-3.49999999998997,
-12.2000000000024));
#46212=CARTESIAN_POINT('Ctrl Pts',(4.96254670649323E-12,-3.49999999998997,
-12.2000000000027));
#46213=CARTESIAN_POINT('Ctrl Pts',(3.49999999999826,-3.49999999998997,-12.200000000003));
#46214=CARTESIAN_POINT('Ctrl Pts',(3.49999999999826,3.32743465443771E-12,
-12.2000000000027));
#46215=CARTESIAN_POINT('Ctrl Pts',(3.49999999999826,3.49999999999662,-12.2000000000024));
#46216=CARTESIAN_POINT('Ctrl Pts',(4.96254670649327E-12,3.49999999999662,
-12.2000000000021));
#46217=CARTESIAN_POINT('Ctrl Pts',(-3.49999999998833,3.49999999999662,-12.2000000000018));
#46218=CARTESIAN_POINT('Ctrl Pts',(-3.49999999998833,3.32743465443771E-12,
-12.2000000000021));
#46219=CARTESIAN_POINT('Ctrl Pts',(-4.62347603751425,3.32743465443744E-12,
-12.199999999999));
#46220=CARTESIAN_POINT('Ctrl Pts',(-4.62347603751425,-4.62347603751589,
-12.1999999999994));
#46221=CARTESIAN_POINT('Ctrl Pts',(4.96254670649346E-12,-4.62347603751589,
-12.1999999999998));
#46222=CARTESIAN_POINT('Ctrl Pts',(4.62347603752418,-4.62347603751589,-12.2000000000002));
#46223=CARTESIAN_POINT('Ctrl Pts',(4.62347603752418,3.32743465443745E-12,
-12.1999999999998));
#46224=CARTESIAN_POINT('Ctrl Pts',(4.62347603752418,4.62347603752254,-12.1999999999994));
#46225=CARTESIAN_POINT('Ctrl Pts',(4.96254670649352E-12,4.62347603752254,
-12.199999999999));
#46226=CARTESIAN_POINT('Ctrl Pts',(-4.62347603751425,4.62347603752254,-12.1999999999986));
#46227=CARTESIAN_POINT('Ctrl Pts',(-4.62347603751425,3.32743465443744E-12,
-12.199999999999));
#46228=CARTESIAN_POINT('Ctrl Pts',(-5.62084621677168,3.28230425252773E-12,
-11.6828432225872));
#46229=CARTESIAN_POINT('Ctrl Pts',(-5.62084621677167,-5.6208462167734,-11.6828432225877));
#46230=CARTESIAN_POINT('Ctrl Pts',(5.00412375663656E-12,-5.6208462167734,
-11.6828432225882));
#46231=CARTESIAN_POINT('Ctrl Pts',(5.62084621678168,-5.6208462167734,-11.6828432225886));
#46232=CARTESIAN_POINT('Ctrl Pts',(5.62084621678168,3.28230425252773E-12,
-11.6828432225881));
#46233=CARTESIAN_POINT('Ctrl Pts',(5.62084621678168,5.62084621677996,-11.6828432225876));
#46234=CARTESIAN_POINT('Ctrl Pts',(5.00412375663663E-12,5.62084621677996,
-11.6828432225872));
#46235=CARTESIAN_POINT('Ctrl Pts',(-5.62084621677167,5.62084621677996,-11.6828432225867));
#46236=CARTESIAN_POINT('Ctrl Pts',(-5.62084621677168,3.28230425252773E-12,
-11.6828432225872));
#46237=CARTESIAN_POINT('',(-0.5,5.484827557301,-11.73961639634));
#46238=CARTESIAN_POINT('',(0.5,5.484827557301,-11.73961639634));
#46239=CARTESIAN_POINT('Ctrl Pts',(0.500000000000787,5.48482755730098,-11.7396163963385));
#46240=CARTESIAN_POINT('Ctrl Pts',(0.442684070576578,5.51791892458297,-11.7261817950198));
#46241=CARTESIAN_POINT('Ctrl Pts',(0.381778410179616,5.54550032053989,-11.7147465052769));
#46242=CARTESIAN_POINT('Ctrl Pts',(0.225874984854292,5.59779342699823,-11.6928840241783));
#46243=CARTESIAN_POINT('Ctrl Pts',(0.129395940067804,5.6152273204819,-11.685424085685));
#46244=CARTESIAN_POINT('Ctrl Pts',(-0.0633603875161564,5.62128903423765,
-11.6828439564321));
#46245=CARTESIAN_POINT('Ctrl Pts',(-0.15776624407999,5.6107743725528,-11.6873559211886));
#46246=CARTESIAN_POINT('Ctrl Pts',(-0.337799258730956,5.56446316521236,
-11.706856455775));
#46247=CARTESIAN_POINT('Ctrl Pts',(-0.422085563497117,5.5298114781902,-11.7213535957186));
#46248=CARTESIAN_POINT('Ctrl Pts',(-0.500000000000555,5.48482755730112,
-11.7396163963379));
#46249=CARTESIAN_POINT('',(4.5,3.175426480543,-11.73961639634));
#46250=CARTESIAN_POINT('Ctrl Pts',(4.49999999999983,3.17542648054266,-11.7396163963401));
#46251=CARTESIAN_POINT('Ctrl Pts',(4.44888679227145,3.20493670478379,-11.7515971070228));
#46252=CARTESIAN_POINT('Ctrl Pts',(4.39760419976511,3.23454472337207,-11.7629653582921));
#46253=CARTESIAN_POINT('Ctrl Pts',(3.72427898920667,3.62328921494017,-11.9041229940746));
#46254=CARTESIAN_POINT('Ctrl Pts',(3.08384652281725,3.99304307180789,-11.9489869609561));
#46255=CARTESIAN_POINT('Ctrl Pts',(2.50000000000225,4.33012701892057,-11.9489869609561));
#46256=CARTESIAN_POINT('Ctrl Pts',(1.91615347718725,4.66721096603325,-11.948986960956));
#46257=CARTESIAN_POINT('Ctrl Pts',(1.27572101079784,5.03696482290097,-11.9041229940743));
#46258=CARTESIAN_POINT('Ctrl Pts',(0.602395800237954,5.4257093144699,-11.7629653582913));
#46259=CARTESIAN_POINT('Ctrl Pts',(0.551113207730164,5.45531733305902,-11.7515971070216));
#46260=CARTESIAN_POINT('Ctrl Pts',(0.500000000000331,5.48482755730098,-11.7396163963385));
#46261=CARTESIAN_POINT('',(5.,2.309401076759,-11.73961639634));
#46262=CARTESIAN_POINT('Ctrl Pts',(4.50000000000015,3.17542648054335,-11.7396163963398));
#46263=CARTESIAN_POINT('Ctrl Pts',(4.57791443650374,3.13044255965423,-11.7213535957204));
#46264=CARTESIAN_POINT('Ctrl Pts',(4.65006683013206,3.07477432204653,-11.7068564557768));
#46265=CARTESIAN_POINT('Ctrl Pts',(4.78019001949428,2.94201676150879,-11.6873559211905));
#46266=CARTESIAN_POINT('Ctrl Pts',(4.83649891190742,2.86551622230077,-11.682843956434));
#46267=CARTESIAN_POINT('Ctrl Pts',(4.92762747759628,2.6955534889947,-11.6854240856869));
#46268=CARTESIAN_POINT('Ctrl Pts',(4.96076880534568,2.60328323853475,-11.6928840241803));
#46269=CARTESIAN_POINT('Ctrl Pts',(4.99343335937216,2.44212035843757,-11.7147465052788));
#46270=CARTESIAN_POINT('Ctrl Pts',(5.,2.37558381132197,-11.7261817950215));
#46271=CARTESIAN_POINT('Ctrl Pts',(5.,2.30940107675898,-11.7396163963399));
#46272=CARTESIAN_POINT('',(5.,-2.309401076759,-11.73961639634));
#46273=CARTESIAN_POINT('Ctrl Pts',(5.,-2.30940107675881,-11.739616396339));
#46274=CARTESIAN_POINT('Ctrl Pts',(5.,-2.25038062827441,-11.7515971070222));
#46275=CARTESIAN_POINT('Ctrl Pts',(5.,-2.19116459109572,-11.762965358292));
#46276=CARTESIAN_POINT('Ctrl Pts',(5.,-1.41367560795741,-11.9041229940749));
#46277=CARTESIAN_POINT('Ctrl Pts',(5.,-0.674167894222026,-11.9489869609566));
#46278=CARTESIAN_POINT('Ctrl Pts',(5.,3.30552965419114E-12,-11.9489869609566));
#46279=CARTESIAN_POINT('Ctrl Pts',(5.,0.674167894228636,-11.9489869609565));
#46280=CARTESIAN_POINT('Ctrl Pts',(5.,1.41367560796401,-11.9041229940747));
#46281=CARTESIAN_POINT('Ctrl Pts',(5.,2.19116459110015,-11.762965358292));
#46282=CARTESIAN_POINT('Ctrl Pts',(5.,2.25038062827671,-11.7515971070227));
#46283=CARTESIAN_POINT('Ctrl Pts',(5.,2.30940107675899,-11.7396163963399));
#46284=CARTESIAN_POINT('',(4.5,-3.175426480543,-11.73961639634));
#46285=CARTESIAN_POINT('Ctrl Pts',(5.,-2.3094010767588,-11.739616396339));
#46286=CARTESIAN_POINT('Ctrl Pts',(5.00000000000002,-2.39936891853743,-11.7213535957195));
#46287=CARTESIAN_POINT('Ctrl Pts',(4.98786608886193,-2.48968884316767,-11.7068564557758));
#46288=CARTESIAN_POINT('Ctrl Pts',(4.93795626357266,-2.66875761104596,-11.6873559211893));
#46289=CARTESIAN_POINT('Ctrl Pts',(4.89985929942184,-2.75577281193861,-11.6828439564328));
#46290=CARTESIAN_POINT('Ctrl Pts',(4.79823153752659,-2.91967383148839,-11.6854240856856));
#46291=CARTESIAN_POINT('Ctrl Pts',(4.73489382048948,-2.99451018846436,-11.692884024179));
#46292=CARTESIAN_POINT('Ctrl Pts',(4.61165494919162,-3.10337996210302,-11.7147465052774));
#46293=CARTESIAN_POINT('Ctrl Pts',(4.55731592942336,-3.14233511326201,-11.7261817950201));
#46294=CARTESIAN_POINT('Ctrl Pts',(4.49999999999993,-3.17542648054348,-11.7396163963385));
#46295=CARTESIAN_POINT('',(0.5,-5.484827557301,-11.73961639634));
#46296=CARTESIAN_POINT('Ctrl Pts',(0.500000000000835,-5.48482755730095,
-11.7396163963363));
#46297=CARTESIAN_POINT('Ctrl Pts',(0.551113207731787,-5.45531733305834,
-11.7515971070197));
#46298=CARTESIAN_POINT('Ctrl Pts',(0.602395800240705,-5.42570931446857,
-11.7629653582897));
#46299=CARTESIAN_POINT('Ctrl Pts',(1.27572101080142,-5.03696482289917,-11.904122994073));
#46300=CARTESIAN_POINT('Ctrl Pts',(1.91615347719049,-4.66721096603164,-11.948986960955));
#46301=CARTESIAN_POINT('Ctrl Pts',(2.50000000000522,-4.33012701891911,-11.948986960955));
#46302=CARTESIAN_POINT('Ctrl Pts',(3.08384652281996,-3.99304307180658,-11.948986960955));
#46303=CARTESIAN_POINT('Ctrl Pts',(3.72427898920903,-3.62328921493906,-11.9041229940731));
#46304=CARTESIAN_POINT('Ctrl Pts',(4.39760419976643,-3.23454472337157,-11.7629653582905));
#46305=CARTESIAN_POINT('Ctrl Pts',(4.44888679227204,-3.20493670478371,-11.7515971070213));
#46306=CARTESIAN_POINT('Ctrl Pts',(4.49999999999971,-3.17542648054299,-11.7396163963387));
#46307=CARTESIAN_POINT('',(-0.5,-5.484827557301,-11.73961639634));
#46308=CARTESIAN_POINT('Ctrl Pts',(0.50000000000084,-5.48482755730095,-11.7396163963363));
#46309=CARTESIAN_POINT('Ctrl Pts',(0.422085563496947,-5.52981147819033,
-11.7213535957167));
#46310=CARTESIAN_POINT('Ctrl Pts',(0.337799258730246,-5.56446316521267,
-11.7068564557729));
#46311=CARTESIAN_POINT('Ctrl Pts',(0.157766244078805,-5.61077437255297,
-11.6873559211863));
#46312=CARTESIAN_POINT('Ctrl Pts',(0.0633603875151218,-5.6212890342377,
-11.6828439564298));
#46313=CARTESIAN_POINT('Ctrl Pts',(-0.129395940068389,-5.6152273204818,
-11.6854240856825));
#46314=CARTESIAN_POINT('Ctrl Pts',(-0.225874984854586,-5.59779342699814,
-11.6928840241757));
#46315=CARTESIAN_POINT('Ctrl Pts',(-0.381778410179812,-5.54550032053983,
-11.7147465052743));
#46316=CARTESIAN_POINT('Ctrl Pts',(-0.442684070576918,-5.51791892458282,
-11.7261817950172));
#46317=CARTESIAN_POINT('Ctrl Pts',(-0.500000000001249,-5.48482755730072,
-11.7396163963359));
#46318=CARTESIAN_POINT('',(-4.5,-3.175426480543,-11.73961639634));
#46319=CARTESIAN_POINT('Ctrl Pts',(-4.49999999999882,-3.17542648054325,
-11.7396163963343));
#46320=CARTESIAN_POINT('Ctrl Pts',(-4.44888679226865,-3.20493670478541,
-11.7515971070176));
#46321=CARTESIAN_POINT('Ctrl Pts',(-4.39760419976052,-3.23454472337472,
-11.7629653582874));
#46322=CARTESIAN_POINT('Ctrl Pts',(-3.72427898920092,-3.62328921494349,
-11.9041229940708));
#46323=CARTESIAN_POINT('Ctrl Pts',(-3.08384652281212,-3.99304307181085,
-11.9489869609528));
#46324=CARTESIAN_POINT('Ctrl Pts',(-2.49999999999764,-4.33012701892324,
-11.9489869609528));
#46325=CARTESIAN_POINT('Ctrl Pts',(-1.91615347718316,-4.66721096603562,
-11.9489869609529));
#46326=CARTESIAN_POINT('Ctrl Pts',(-1.27572101079435,-5.03696482290299,
-11.9041229940711));
#46327=CARTESIAN_POINT('Ctrl Pts',(-0.602395800236188,-5.42570931447092,
-11.7629653582882));
#46328=CARTESIAN_POINT('Ctrl Pts',(-0.551113207729517,-5.45531733305939,
-11.7515971070188));
#46329=CARTESIAN_POINT('Ctrl Pts',(-0.500000000000796,-5.48482755730071,
-11.7396163963359));
#46330=CARTESIAN_POINT('',(-5.,-2.309401076759,-11.73961639634));
#46331=CARTESIAN_POINT('Ctrl Pts',(-4.49999999999914,-3.17542648054393,
-11.739616396334));
#46332=CARTESIAN_POINT('Ctrl Pts',(-4.5779144365027,-3.13044255965495,-11.7213535957145));
#46333=CARTESIAN_POINT('Ctrl Pts',(-4.65006683013103,-3.0747743220474,-11.7068564557708));
#46334=CARTESIAN_POINT('Ctrl Pts',(-4.78019001949316,-2.94201676151012,
-11.6873559211842));
#46335=CARTESIAN_POINT('Ctrl Pts',(-4.83649891190626,-2.86551622230246,
-11.6828439564276));
#46336=CARTESIAN_POINT('Ctrl Pts',(-4.92762747759513,-2.69555348899732,
-11.6854240856803));
#46337=CARTESIAN_POINT('Ctrl Pts',(-4.96076880534464,-2.60328323853797,
-11.6928840241735));
#46338=CARTESIAN_POINT('Ctrl Pts',(-4.99343335937199,-2.44212035843974,
-11.7147465052721));
#46339=CARTESIAN_POINT('Ctrl Pts',(-5.00000000000008,-2.37558381132245,
-11.7261817950152));
#46340=CARTESIAN_POINT('Ctrl Pts',(-5.,-2.30940107675779,-11.739616396334));
#46341=CARTESIAN_POINT('',(-5.,3.30530319330631E-12,-11.9489869609522));
#46342=CARTESIAN_POINT('Ctrl Pts',(-5.,3.30541150006525E-12,-11.9489869609522));
#46343=CARTESIAN_POINT('Ctrl Pts',(-5.,-0.674167894221416,-11.9489869609523));
#46344=CARTESIAN_POINT('Ctrl Pts',(-5.,-1.41367560795614,-11.9041229940705));
#46345=CARTESIAN_POINT('Ctrl Pts',(-5.,-2.19116459109405,-11.7629653582872));
#46346=CARTESIAN_POINT('Ctrl Pts',(-5.,-2.25038062827307,-11.7515971070173));
#46347=CARTESIAN_POINT('Ctrl Pts',(-5.,-2.30940107675779,-11.739616396334));
#46348=CARTESIAN_POINT('Ctrl Pts',(-5.,3.3055296541908E-12,-11.9489869609522));
#46349=CARTESIAN_POINT('Ctrl Pts',(-4.27100251525133,3.32743465443753E-12,
-12.2));
#46350=CARTESIAN_POINT('Ctrl Pts',(-3.49999999998833,3.32743465443771E-12,
-12.2000000000021));
#46351=CARTESIAN_POINT('',(-5.,2.309401076758,-11.73961639634));
#46352=CARTESIAN_POINT('Ctrl Pts',(-5.,2.30940107675701,-11.7396163963351));
#46353=CARTESIAN_POINT('Ctrl Pts',(-5.,2.25038062827473,-11.7515971070179));
#46354=CARTESIAN_POINT('Ctrl Pts',(-5.,2.19116459109816,-11.7629653582873));
#46355=CARTESIAN_POINT('Ctrl Pts',(-5.,1.41367560796274,-11.9041229940702));
#46356=CARTESIAN_POINT('Ctrl Pts',(-5.,0.674167894228026,-11.9489869609522));
#46357=CARTESIAN_POINT('Ctrl Pts',(-5.,3.3056890558214E-12,-11.9489869609522));
#46358=CARTESIAN_POINT('',(-4.5,3.175426480543,-11.73961639634));
#46359=CARTESIAN_POINT('Ctrl Pts',(-5.,2.30940107675701,-11.7396163963351));
#46360=CARTESIAN_POINT('Ctrl Pts',(-5.00000000000018,2.39936891853531,-11.7213535957156));
#46361=CARTESIAN_POINT('Ctrl Pts',(-4.98786608886234,2.48968884316526,-11.7068564557719));
#46362=CARTESIAN_POINT('Ctrl Pts',(-4.93795626357369,2.66875761104321,-11.6873559211853));
#46363=CARTESIAN_POINT('Ctrl Pts',(-4.8998592994232,2.75577281193584,-11.6828439564288));
#46364=CARTESIAN_POINT('Ctrl Pts',(-4.79823153752867,2.91967383148563,-11.6854240856815));
#46365=CARTESIAN_POINT('Ctrl Pts',(-4.73489382049198,2.99451018846164,-11.6928840241748));
#46366=CARTESIAN_POINT('Ctrl Pts',(-4.61165494919357,3.10337996210165,-11.7147465052734));
#46367=CARTESIAN_POINT('Ctrl Pts',(-4.55731592942412,3.14233511326163,-11.7261817950164));
#46368=CARTESIAN_POINT('Ctrl Pts',(-4.49999999999936,3.17542648054381,-11.7396163963353));
#46369=CARTESIAN_POINT('Ctrl Pts',(-0.500000000000548,5.48482755730111,
-11.7396163963379));
#46370=CARTESIAN_POINT('Ctrl Pts',(-0.551113207728163,5.45531733306043,
-11.7515971070205));
#46371=CARTESIAN_POINT('Ctrl Pts',(-0.60239580023372,5.4257093144726,-11.7629653582897));
#46372=CARTESIAN_POINT('Ctrl Pts',(-1.27572101079105,5.03696482290515,-11.9041229940722));
#46373=CARTESIAN_POINT('Ctrl Pts',(-1.91615347718016,4.6672109660376,-11.9489869609538));
#46374=CARTESIAN_POINT('Ctrl Pts',(-2.49999999999489,4.33012701892508,-11.9489869609538));
#46375=CARTESIAN_POINT('Ctrl Pts',(-3.08384652280961,3.99304307181256,-11.9489869609537));
#46376=CARTESIAN_POINT('Ctrl Pts',(-3.72427898919873,3.62328921494501,-11.9041229940721));
#46377=CARTESIAN_POINT('Ctrl Pts',(-4.39760419975937,3.23454472337564,-11.7629653582888));
#46378=CARTESIAN_POINT('Ctrl Pts',(-4.44888679226823,3.20493670478591,-11.7515971070189));
#46379=CARTESIAN_POINT('Ctrl Pts',(-4.49999999999913,3.17542648054333,-11.7396163963355));
#46380=CARTESIAN_POINT('Origin',(0.,4.618802153517,-28.10392));
#46381=CARTESIAN_POINT('',(0.5,5.484827557301,-10.5));
#46382=CARTESIAN_POINT('',(-0.5,5.484827557301,-10.5));
#46383=CARTESIAN_POINT('Origin',(0.,4.618802153517,-10.5));
#46384=CARTESIAN_POINT('',(0.5,5.484827557301,-11.73961639634));
#46385=CARTESIAN_POINT('',(-0.5,5.484827557301,-11.73961639634));
#46386=CARTESIAN_POINT('Origin',(0.,0.,-10.5));
#46387=CARTESIAN_POINT('',(-4.5,3.175426480543,-10.5));
#46388=CARTESIAN_POINT('',(-4.5,3.175426480543,-10.5));
#46389=CARTESIAN_POINT('',(-5.,2.309401076759,-10.5));
#46390=CARTESIAN_POINT('Origin',(-4.,2.309401076759,-10.5));
#46391=CARTESIAN_POINT('',(-5.,-2.309401076759,-10.5));
#46392=CARTESIAN_POINT('',(-5.,-2.309401076759,-10.5));
#46393=CARTESIAN_POINT('',(-4.5,-3.175426480543,-10.5));
#46394=CARTESIAN_POINT('Origin',(-4.,-2.309401076759,-10.5));
#46395=CARTESIAN_POINT('',(-0.5,-5.484827557301,-10.5));
#46396=CARTESIAN_POINT('',(-0.5,-5.484827557301,-10.5));
#46397=CARTESIAN_POINT('',(0.5,-5.484827557301,-10.5));
#46398=CARTESIAN_POINT('Origin',(0.,-4.618802153517,-10.5));
#46399=CARTESIAN_POINT('',(4.5,-3.175426480543,-10.5));
#46400=CARTESIAN_POINT('',(4.5,-3.175426480543,-10.5));
#46401=CARTESIAN_POINT('',(5.,-2.309401076759,-10.5));
#46402=CARTESIAN_POINT('Origin',(4.,-2.309401076759,-10.5));
#46403=CARTESIAN_POINT('',(5.,2.309401076759,-10.5));
#46404=CARTESIAN_POINT('',(5.,2.309401076759,-10.5));
#46405=CARTESIAN_POINT('',(4.5,3.175426480543,-10.5));
#46406=CARTESIAN_POINT('Origin',(4.,2.309401076759,-10.5));
#46407=CARTESIAN_POINT('',(0.5,5.484827557301,-10.5));
#46408=CARTESIAN_POINT('',(0.,4.,-10.5));
#46409=CARTESIAN_POINT('Origin',(0.,0.,-10.5));
#46410=CARTESIAN_POINT('Origin',(0.,0.,0.525));
#46411=CARTESIAN_POINT('',(5.89886872482066E-17,4.,-7.77511165445773));
#46412=CARTESIAN_POINT('',(4.89858719658941E-16,4.,0.525));
#46413=CARTESIAN_POINT('',(3.46410161481665,-1.99999999976831,-8.02507037766139));
#46414=CARTESIAN_POINT('Ctrl Pts',(3.2612801348364E-15,4.,-7.77511165445773));
#46415=CARTESIAN_POINT('Ctrl Pts',(0.140778732285844,4.,-7.77934161327365));
#46416=CARTESIAN_POINT('Ctrl Pts',(0.281562623126605,3.99256795970819,-7.78354814467748));
#46417=CARTESIAN_POINT('Ctrl Pts',(0.653870198275523,3.95309174821613,-7.79466178870193));
#46418=CARTESIAN_POINT('Ctrl Pts',(0.883378592649572,3.90821221631589,-7.80149898784317));
#46419=CARTESIAN_POINT('Ctrl Pts',(1.41065467753745,3.75625914261328,-7.81796018704639));
#46420=CARTESIAN_POINT('Ctrl Pts',(1.70226943948582,3.63341618820113,-7.82745442148589));
#46421=CARTESIAN_POINT('Ctrl Pts',(2.19330078093717,3.35434968240981,-7.8441809508052));
#46422=CARTESIAN_POINT('Ctrl Pts',(2.39817450095537,3.21107275634099,-7.85153722441686));
#46423=CARTESIAN_POINT('Ctrl Pts',(2.78217511180761,2.88515562249177,-7.86670078290223));
#46424=CARTESIAN_POINT('Ctrl Pts',(2.95986659741527,2.70255684997506,-7.87432379850575));
#46425=CARTESIAN_POINT('Ctrl Pts',(3.2746594474262,2.31049777386795,-7.88922429124318));
#46426=CARTESIAN_POINT('Ctrl Pts',(3.41188551680376,2.10257724441769,-7.89653713856435));
#46427=CARTESIAN_POINT('Ctrl Pts',(3.64749116775576,1.66109269263352,-7.91159591530977));
#46428=CARTESIAN_POINT('Ctrl Pts',(3.74481430291147,1.42821183215052,-7.91916263122237));
#46429=CARTESIAN_POINT('Ctrl Pts',(3.89268525469654,0.952677249501694,-7.93393539966148));
#46430=CARTESIAN_POINT('Ctrl Pts',(3.9439231690797,0.711380494141654,-7.9411566697106));
#46431=CARTESIAN_POINT('Ctrl Pts',(3.99685095219547,0.261048337853231,-7.95478618466598));
#46432=CARTESIAN_POINT('Ctrl Pts',(4.00500813357676,0.0536167255429015,
-7.96103764007249));
#46433=CARTESIAN_POINT('Ctrl Pts',(3.98489990856592,-0.469954806053514,
-7.97666285858365));
#46434=CARTESIAN_POINT('Ctrl Pts',(3.93521088393896,-0.78383650500982,-7.98590074114378));
#46435=CARTESIAN_POINT('Ctrl Pts',(3.80435504362991,-1.24652798426401,-8.00036597408868));
#46436=CARTESIAN_POINT('Ctrl Pts',(3.74999731300928,-1.40159549116537,-8.00531733948733));
#46437=CARTESIAN_POINT('Ctrl Pts',(3.62159245785615,-1.70640549464178,-8.0152126777857));
#46438=CARTESIAN_POINT('Ctrl Pts',(3.54739645091892,-1.85572911241389,-8.02014529730486));
#46439=CARTESIAN_POINT('Ctrl Pts',(3.46410161516789,-1.9999999999478,-8.02507037834385));
#46440=CARTESIAN_POINT('',(3.4640667802615,-1.999976852445,-7.27511360468106));
#46441=CARTESIAN_POINT('',(3.464101615138,-2.,-8.025));
#46442=CARTESIAN_POINT('Ctrl Pts',(3.46410332849671,-1.99999703237231,-7.27513768185083));
#46443=CARTESIAN_POINT('Ctrl Pts',(3.35586300106758,-2.18747514981733,-7.28160344842495));
#46444=CARTESIAN_POINT('Ctrl Pts',(3.23258197797168,-2.36585667498483,-7.28797035088014));
#46445=CARTESIAN_POINT('Ctrl Pts',(2.96253849585541,-2.69581554812532,-7.30060798938785));
#46446=CARTESIAN_POINT('Ctrl Pts',(2.81702488992057,-2.84752954740615,-7.30693910263489));
#46447=CARTESIAN_POINT('Ctrl Pts',(2.34305642289716,-3.26963843275094,-7.32602735225743));
#46448=CARTESIAN_POINT('Ctrl Pts',(1.98284299927815,-3.49982606803557,-7.33834991377517));
#46449=CARTESIAN_POINT('Ctrl Pts',(1.3604085738985,-3.77010588037409,-7.35876508310621));
#46450=CARTESIAN_POINT('Ctrl Pts',(1.11852150423245,-3.84880786584587,-7.3663943452422));
#46451=CARTESIAN_POINT('Ctrl Pts',(0.616447115067628,-3.96079714425207,
-7.38165683539358));
#46452=CARTESIAN_POINT('Ctrl Pts',(0.357146543798483,-3.992538907047,-7.38930579330697));
#46453=CARTESIAN_POINT('Ctrl Pts',(-0.157696072795193,-4.00497685917401,
-7.40479909079884));
#46454=CARTESIAN_POINT('Ctrl Pts',(-0.412009437255292,-3.98684818401563,
-7.412446025683));
#46455=CARTESIAN_POINT('Ctrl Pts',(-0.919900651375685,-3.90150110816807,
-7.4277259558367));
#46456=CARTESIAN_POINT('Ctrl Pts',(-1.17208922886167,-3.83329289933414,
-7.4353757396454));
#46457=CARTESIAN_POINT('Ctrl Pts',(-1.65312578169036,-3.65123835423638,
-7.45084951467785));
#46458=CARTESIAN_POINT('Ctrl Pts',(-1.88132825994924,-3.53906383830923,
-7.45847619461585));
#46459=CARTESIAN_POINT('Ctrl Pts',(-2.31928013956748,-3.26938214774931,
-7.47373613423981));
#46460=CARTESIAN_POINT('Ctrl Pts',(-2.52730851911268,-3.11137126658911,
-7.48138496898291));
#46461=CARTESIAN_POINT('Ctrl Pts',(-2.90515881640126,-2.76130583412243,
-7.49688111703797));
#46462=CARTESIAN_POINT('Ctrl Pts',(-3.07490559617139,-2.57093674770182,
-7.50453101279154));
#46463=CARTESIAN_POINT('Ctrl Pts',(-3.37956067272974,-2.15557391372885,
-7.51981386213054));
#46464=CARTESIAN_POINT('Ctrl Pts',(-3.51279729686478,-1.93085056262191,
-7.52746378143529));
#46465=CARTESIAN_POINT('Ctrl Pts',(-3.7306700897575,-1.46506312330292,-7.54293428241289));
#46466=CARTESIAN_POINT('Ctrl Pts',(-3.81602919117647,-1.22565614517854,
-7.55055756936701));
#46467=CARTESIAN_POINT('Ctrl Pts',(-3.94198275788177,-0.727111070355683,
-7.56581415670827));
#46468=CARTESIAN_POINT('Ctrl Pts',(-3.98097214940275,-0.468805753691623,
-7.57346282862271));
#46469=CARTESIAN_POINT('Ctrl Pts',(-4.00783408750042,0.0457088510394772,
-7.58896272305745));
#46470=CARTESIAN_POINT('Ctrl Pts',(-3.99680256889971,0.300657827573293,
-7.59661651140217));
#46471=CARTESIAN_POINT('Ctrl Pts',(-3.9255927125405,0.810957805583728,-7.61190319735917));
#46472=CARTESIAN_POINT('Ctrl Pts',(-3.86442850093518,1.06495191091268,-7.61955329356721));
#46473=CARTESIAN_POINT('Ctrl Pts',(-3.69591527108494,1.55062713376603,-7.63501948572712));
#46474=CARTESIAN_POINT('Ctrl Pts',(-3.59026664206739,1.7816346800881,-7.64263830916872));
#46475=CARTESIAN_POINT('Ctrl Pts',(-3.34220362495083,2.21098074661499,-7.65735043678452));
#46476=CARTESIAN_POINT('Ctrl Pts',(-3.20210686624951,2.40941328215933,-7.66445800738338));
#46477=CARTESIAN_POINT('Ctrl Pts',(-2.90970717095085,2.75264826764198,-7.67800500544158));
#46478=CARTESIAN_POINT('Ctrl Pts',(-2.76230107077787,2.9005451583952,-7.6842970732713));
#46479=CARTESIAN_POINT('Ctrl Pts',(-2.4505214701389,3.16794066444546,-7.69655196788191));
#46480=CARTESIAN_POINT('Ctrl Pts',(-2.28723825110935,3.28777200012571,-7.7025029263712));
#46481=CARTESIAN_POINT('Ctrl Pts',(-1.71869730004351,3.64208556189983,-7.72235370186981));
#46482=CARTESIAN_POINT('Ctrl Pts',(-1.28148120429361,3.81791991428226,-7.73646510285903));
#46483=CARTESIAN_POINT('Ctrl Pts',(-0.696644060123244,3.94101312641292,
-7.75413628251737));
#46484=CARTESIAN_POINT('Ctrl Pts',(-0.568212890367792,3.96156931347538,
-7.7579824927024));
#46485=CARTESIAN_POINT('Ctrl Pts',(-0.293121491848629,3.99194467622145,
-7.76627846400883));
#46486=CARTESIAN_POINT('Ctrl Pts',(-0.146563545278887,4.,-7.77070788017748));
#46487=CARTESIAN_POINT('Ctrl Pts',(1.38777878078145E-15,4.,-7.77511165445773));
#46488=CARTESIAN_POINT('Origin',(3.464101615138,-2.,-8.5));
#46489=CARTESIAN_POINT('',(3.06563522285152,-1.76994531315727,-7.75941845703217));
#46490=CARTESIAN_POINT('Ctrl Pts',(3.0656354288223,-1.76994544006766,-7.75941803818134));
#46491=CARTESIAN_POINT('Ctrl Pts',(3.13205392611679,-1.80829217735981,-7.8036984058573));
#46492=CARTESIAN_POINT('Ctrl Pts',(3.19847242341131,-1.84663891465196,-7.84797877353323));
#46493=CARTESIAN_POINT('Ctrl Pts',(3.33129448534567,-1.92332376786409,-7.9365295534741));
#46494=CARTESIAN_POINT('Ctrl Pts',(3.39769804998552,-1.96166188378406,-7.98079996573903));
#46495=CARTESIAN_POINT('Ctrl Pts',(3.46410161462537,-1.99999999970403,-8.02507037800398));
#46496=CARTESIAN_POINT('',(3.06563502767401,-1.76994519830837,-7.54058067576584));
#46497=CARTESIAN_POINT('Ctrl Pts',(3.06563511413263,-1.76994525838149,-7.54058067576584));
#46498=CARTESIAN_POINT('Ctrl Pts',(3.06563511413263,-1.76994525838149,-7.57705378384389));
#46499=CARTESIAN_POINT('Ctrl Pts',(3.06563511413263,-1.76994525838149,-7.61352689192195));
#46500=CARTESIAN_POINT('Ctrl Pts',(3.06563511413263,-1.76994525838149,-7.68647281901072));
#46501=CARTESIAN_POINT('Ctrl Pts',(3.06563511413263,-1.76994525838149,-7.72294563802144));
#46502=CARTESIAN_POINT('Ctrl Pts',(3.06563511413263,-1.76994525838149,-7.75941845703217));
#46503=CARTESIAN_POINT('Ctrl Pts',(3.46400702067617,-1.999945385862,-7.27499059099672));
#46504=CARTESIAN_POINT('Ctrl Pts',(3.39763472540694,-1.96162532332158,-7.3192401563699));
#46505=CARTESIAN_POINT('Ctrl Pts',(3.33126243013771,-1.92330526078116,-7.36348972174309));
#46506=CARTESIAN_POINT('Ctrl Pts',(3.19847169694209,-1.84663849522478,-7.45201961521233));
#46507=CARTESIAN_POINT('Ctrl Pts',(3.13205325901568,-1.8082917922088,-7.49629994330838));
#46508=CARTESIAN_POINT('Ctrl Pts',(3.06563482108927,-1.76994508919283,-7.54058027140441));
#46509=CARTESIAN_POINT('Ctrl Pts',(0.5039879501212,-3.989475419894,-4.372769611617));
#46510=CARTESIAN_POINT('Ctrl Pts',(-0.0089492302955,-4.054274455078,-4.388116833839));
#46511=CARTESIAN_POINT('Ctrl Pts',(-1.059906716638,-3.983530501776,-4.418811278284));
#46512=CARTESIAN_POINT('Ctrl Pts',(-2.480771754885,-3.292085724309,-4.46485294495));
#46513=CARTESIAN_POINT('Ctrl Pts',(-3.537058667077,-2.116886952389,-4.510894611617));
#46514=CARTESIAN_POINT('Ctrl Pts',(-4.073613014997,-0.6306285969564,-4.556936278284));
#46515=CARTESIAN_POINT('Ctrl Pts',(-4.011576156733,0.9482964751911,-4.60297794495));
#46516=CARTESIAN_POINT('Ctrl Pts',(-3.360068212288,2.387876153023,-4.649019611617));
#46517=CARTESIAN_POINT('Ctrl Pts',(-2.214822403112,3.476574800745,-4.695061278284));
#46518=CARTESIAN_POINT('Ctrl Pts',(-0.7441245898171,4.054416019338,-4.74110294495));
#46519=CARTESIAN_POINT('Ctrl Pts',(0.8359169456045,4.036490248204,-4.787144611617));
#46520=CARTESIAN_POINT('Ctrl Pts',(2.29312655145,3.425431546469,-4.833186278284));
#46521=CARTESIAN_POINT('Ctrl Pts',(3.413377863899,2.311030553742,-4.87922794495));
#46522=CARTESIAN_POINT('Ctrl Pts',(4.03205808599,0.8570404032131,-4.925269611617));
#46523=CARTESIAN_POINT('Ctrl Pts',(4.058256652206,-0.7228856109492,-4.971311278284));
#46524=CARTESIAN_POINT('Ctrl Pts',(3.488123873377,-2.196588833996,-5.01735294495));
#46525=CARTESIAN_POINT('Ctrl Pts',(2.405436621222,-3.347519278951,-5.063394611617));
#46526=CARTESIAN_POINT('Ctrl Pts',(0.9692879252418,-4.006556074691,-5.109436278284));
#46527=CARTESIAN_POINT('Ctrl Pts',(-0.6092905926321,-4.076858549839,-5.15547794495));
#46528=CARTESIAN_POINT('Ctrl Pts',(-2.098338282431,-3.548096266189,-5.201519611617));
#46529=CARTESIAN_POINT('Ctrl Pts',(-3.279050399221,-2.497967001589,-5.247561278284));
#46530=CARTESIAN_POINT('Ctrl Pts',(-3.97792987147,-1.080779625702,-5.29360294495));
#46531=CARTESIAN_POINT('Ctrl Pts',(-4.092281435813,0.4952204678384,-5.339644611617));
#46532=CARTESIAN_POINT('Ctrl Pts',(-3.605301960262,1.998451509793,-5.385686278284));
#46533=CARTESIAN_POINT('Ctrl Pts',(-2.588549542429,3.208024614627,-5.43172794495));
#46534=CARTESIAN_POINT('Ctrl Pts',(-1.19142856672,3.946201798194,-5.477769611617));
#46535=CARTESIAN_POINT('Ctrl Pts',(0.3807641850203,4.104513283822,-5.523811278284));
#46536=CARTESIAN_POINT('Ctrl Pts',(1.897006404783,3.659696348315,-5.56985294495));
#46537=CARTESIAN_POINT('Ctrl Pts',(3.134497308938,2.677113610201,-5.615894611617));
#46538=CARTESIAN_POINT('Ctrl Pts',(3.91139659546,1.30114846758,-5.661936278284));
#46539=CARTESIAN_POINT('Ctrl Pts',(4.113544555839,-0.2660109937444,-5.70797794495));
#46540=CARTESIAN_POINT('Ctrl Pts',(3.711237015243,-1.794082071242,-5.754019611617));
#46541=CARTESIAN_POINT('Ctrl Pts',(2.763590145309,-3.058525816535,-5.800061278284));
#46542=CARTESIAN_POINT('Ctrl Pts',(1.409853772006,-3.873541403319,-5.84610294495));
#46543=CARTESIAN_POINT('Ctrl Pts',(-0.1510503750974,-4.119368209549,-5.892144611617));
#46544=CARTESIAN_POINT('Ctrl Pts',(-1.689758766469,-3.759883771183,-5.938186278284));
#46545=CARTESIAN_POINT('Ctrl Pts',(-2.980169377703,-2.847911715953,-5.98422794495));
#46546=CARTESIAN_POINT('Ctrl Pts',(-3.83266574011,-1.517459714869,-6.030269611617));
#46547=CARTESIAN_POINT('Ctrl Pts',(-4.121979703844,0.03597197191163,-6.076311278284));
#46548=CARTESIAN_POINT('Ctrl Pts',(-3.805598682858,1.584117838639,-6.12235294495));
#46549=CARTESIAN_POINT('Ctrl Pts',(-2.930012570708,2.899489092436,-6.168394611617));
#46550=CARTESIAN_POINT('Ctrl Pts',(-1.623882388293,3.788801479446,-6.214436278284));
#46551=CARTESIAN_POINT('Ctrl Pts',(-0.07913448113579,4.121377002357,-6.26047794495));
#46552=CARTESIAN_POINT('Ctrl Pts',(1.47724166337,3.848346103155,-6.306519611617));
#46553=CARTESIAN_POINT('Ctrl Pts',(2.816547872794,3.009828689797,-6.352561278284));
#46554=CARTESIAN_POINT('Ctrl Pts',(3.741982825359,1.729038807078,-6.39860294495));
#46555=CARTESIAN_POINT('Ctrl Pts',(4.117560575058,0.1941792274952,-6.444644611617));
#46556=CARTESIAN_POINT('Ctrl Pts',(3.888092698922,-1.369213579488,-6.490686278284));
#46557=CARTESIAN_POINT('Ctrl Pts',(3.087297835011,-2.731410393844,-6.53672794495));
#46558=CARTESIAN_POINT('Ctrl Pts',(1.832846973412,-3.692246285626,-6.582769611617));
#46559=CARTESIAN_POINT('Ctrl Pts',(0.3090725587339,-4.110533397882,-6.628811278284));
#46560=CARTESIAN_POINT('Ctrl Pts',(-1.260117824043,-3.924807476958,-6.67485294495));
#46561=CARTESIAN_POINT('Ctrl Pts',(-2.644143043235,-3.162359598245,-6.720894611617));
#46562=CARTESIAN_POINT('Ctrl Pts',(-3.639630643292,-1.935225940801,-6.766936278284));
#46563=CARTESIAN_POINT('Ctrl Pts',(-4.100300950458,-0.4237248845199,-6.81297794495));
#46564=CARTESIAN_POINT('Ctrl Pts',(-3.958461808006,1.150039466741,-6.859019611617));
#46565=CARTESIAN_POINT('Ctrl Pts',(-3.234955449255,2.554813868979,-6.905061278284));
#46566=CARTESIAN_POINT('Ctrl Pts',(-2.036095874727,3.584176928104,-6.95110294495));
#46567=CARTESIAN_POINT('Ctrl Pts',(-0.5380468116679,4.086871205575,-6.997144611617));
#46568=CARTESIAN_POINT('Ctrl Pts',(1.039064377895,3.98902947244,-7.043186278284));
#46569=CARTESIAN_POINT('Ctrl Pts',(2.463492398452,3.305028694111,-7.08922794495));
#46570=CARTESIAN_POINT('Ctrl Pts',(3.525928861993,2.135378440328,-7.135269611617));
#46571=CARTESIAN_POINT('Ctrl Pts',(4.070252841003,0.6519479993433,-7.181311278284));
#46572=CARTESIAN_POINT('Ctrl Pts',(4.016493331088,-0.9272746288775,-7.22735294495));
#46573=CARTESIAN_POINT('Ctrl Pts',(3.372499699855,-2.370266500001,-7.273394611617));
#46574=CARTESIAN_POINT('Ctrl Pts',(2.612892894131,-3.100001962842,-7.304089056061));
#46575=CARTESIAN_POINT('Ctrl Pts',(2.178308200468,-3.380072686139,-7.319436278284));
#46576=CARTESIAN_POINT('Ctrl Pts',(0.4830001770654,-3.823340089268,-4.469450245148));
#46577=CARTESIAN_POINT('Ctrl Pts',(-0.008576553896349,-3.885440672149,-4.48479746737));
#46578=CARTESIAN_POINT('Ctrl Pts',(-1.015768594638,-3.817642737768,-4.515491911815));
#46579=CARTESIAN_POINT('Ctrl Pts',(-2.377463978216,-3.154992073467,-4.561533578481));
#46580=CARTESIAN_POINT('Ctrl Pts',(-3.389763509381,-2.028732577009,-4.607575245148));
#46581=CARTESIAN_POINT('Ctrl Pts',(-3.903973908634,-0.604367076473,-4.653616911815));
#46582=CARTESIAN_POINT('Ctrl Pts',(-3.844520476228,0.908806183397,-4.699658578481));
#46583=CARTESIAN_POINT('Ctrl Pts',(-3.220143539338,2.288436865292,-4.745700245148));
#46584=CARTESIAN_POINT('Ctrl Pts',(-2.12258966234,3.331798397039,-4.791741911815));
#46585=CARTESIAN_POINT('Ctrl Pts',(-0.7131367100223,3.885576341192,-4.837783578481));
#46586=CARTESIAN_POINT('Ctrl Pts',(0.8011065197924,3.86839706016,-4.883825245148));
#46587=CARTESIAN_POINT('Ctrl Pts',(2.197632959513,3.282784921885,-4.929866911815));
#46588=CARTESIAN_POINT('Ctrl Pts',(3.27123319567,2.214791378231,-4.975908578481));
#46589=CARTESIAN_POINT('Ctrl Pts',(3.864149468261,0.8213503247539,-5.021950245148));
#46590=CARTESIAN_POINT('Ctrl Pts',(3.88925703704,-0.6927821944998,-5.067991911815));
#46591=CARTESIAN_POINT('Ctrl Pts',(3.342866526991,-2.105115401081,-5.114033578481));
#46592=CARTESIAN_POINT('Ctrl Pts',(2.305266055846,-3.208117186282,-5.160075245148));
#46593=CARTESIAN_POINT('Ctrl Pts',(0.9289234780445,-3.839709447483,-5.206116911815));
#46594=CARTESIAN_POINT('Ctrl Pts',(-0.5839176592511,-3.907084288362,-5.252158578481));
#46595=CARTESIAN_POINT('Ctrl Pts',(-2.01095633678,-3.400341465311,-5.298200245148));
#46596=CARTESIAN_POINT('Ctrl Pts',(-3.142499583669,-2.393943156341,-5.344241911815));
#46597=CARTESIAN_POINT('Ctrl Pts',(-3.812275336764,-1.035772284748,-5.390283578481));
#46598=CARTESIAN_POINT('Ctrl Pts',(-3.921864912888,0.474597802576,-5.436325245148));
#46599=CARTESIAN_POINT('Ctrl Pts',(-3.455164919641,1.915229189219,-5.482366911815));
#46600=CARTESIAN_POINT('Ctrl Pts',(-2.480753531974,3.07443155441,-5.528408578481));
#46601=CARTESIAN_POINT('Ctrl Pts',(-1.14181342738,3.781868528414,-5.574450245148));
#46602=CARTESIAN_POINT('Ctrl Pts',(0.3649078688106,3.933587385127,-5.620491911815));
#46603=CARTESIAN_POINT('Ctrl Pts',(1.818008603547,3.5072941403,-5.666533578481));
#46604=CARTESIAN_POINT('Ctrl Pts',(3.003966175905,2.565629490626,-5.712575245148));
#46605=CARTESIAN_POINT('Ctrl Pts',(3.748512732746,1.246964218249,-5.758616911815));
#46606=CARTESIAN_POINT('Ctrl Pts',(3.942242564249,-0.2549333908657,-5.804658578481));
#46607=CARTESIAN_POINT('Ctrl Pts',(3.55668847849,-1.719370389453,-5.850700245148));
#46608=CARTESIAN_POINT('Ctrl Pts',(2.648504848577,-2.931158394938,-5.896741911815));
#46609=CARTESIAN_POINT('Ctrl Pts',(1.351142663929,-3.712233959607,-5.942783578481));
#46610=CARTESIAN_POINT('Ctrl Pts',(-0.1447601235313,-3.947823701204,-5.988825245148));
#46611=CARTESIAN_POINT('Ctrl Pts',(-1.61939146205,-3.603309417992,-6.034866911815));
#46612=CARTESIAN_POINT('Ctrl Pts',(-2.856064984826,-2.729314982116,-6.080908578481));
#46613=CARTESIAN_POINT('Ctrl Pts',(-3.673060498094,-1.454267529204,-6.126950245148));
#46614=CARTESIAN_POINT('Ctrl Pts',(-3.95032644399,0.03447397660704,-6.172991911815));
#46615=CARTESIAN_POINT('Ctrl Pts',(-3.647120605201,1.518149781897,-6.219033578481));
#46616=CARTESIAN_POINT('Ctrl Pts',(-2.807996877932,2.778744501151,-6.265075245148));
#46617=CARTESIAN_POINT('Ctrl Pts',(-1.556258400404,3.631022894492,-6.311116911815));
#46618=CARTESIAN_POINT('Ctrl Pts',(-0.07583905208719,3.949748841044,-6.357158578481));
#46619=CARTESIAN_POINT('Ctrl Pts',(1.41572429421,3.688087877469,-6.403200245148));
#46620=CARTESIAN_POINT('Ctrl Pts',(2.699257236101,2.884489182249,-6.449241911815));
#46621=CARTESIAN_POINT('Ctrl Pts',(3.58615392846,1.657035748118,-6.495283578481));
#46622=CARTESIAN_POINT('Ctrl Pts',(3.946091342763,0.1860929437699,-6.541325245148));
#46623=CARTESIAN_POINT('Ctrl Pts',(3.726179289751,-1.312194867306,-6.587366911815));
#46624=CARTESIAN_POINT('Ctrl Pts',(2.958732248669,-2.617665171454,-6.633408578481));
#46625=CARTESIAN_POINT('Ctrl Pts',(1.7565209892,-3.53848858747,-6.679450245148));
#46626=CARTESIAN_POINT('Ctrl Pts',(0.2962017257726,-3.939356801155,-6.725491911815));
#46627=CARTESIAN_POINT('Ctrl Pts',(-1.207642230314,-3.761365139508,-6.771533578481));
#46628=CARTESIAN_POINT('Ctrl Pts',(-2.53403193025,-3.030668184684,-6.817575245148));
#46629=CARTESIAN_POINT('Ctrl Pts',(-3.488064039506,-1.854636548043,-6.863616911815));
#46630=CARTESIAN_POINT('Ctrl Pts',(-3.929550467657,-0.4060795386098,-6.909658578481));
#46631=CARTESIAN_POINT('Ctrl Pts',(-3.793617989703,1.102147910351,-6.955700245148));
#46632=CARTESIAN_POINT('Ctrl Pts',(-3.100240897452,2.448422726752,-7.001741911815));
#46633=CARTESIAN_POINT('Ctrl Pts',(-1.951305914712,3.434919605699,-7.047783578481));
#46634=CARTESIAN_POINT('Ctrl Pts',(-0.5156407117324,3.916679983045,-7.093825245148));
#46635=CARTESIAN_POINT('Ctrl Pts',(0.9957942017955,3.822912712584,-7.139866911815));
#46636=CARTESIAN_POINT('Ctrl Pts',(2.360904192978,3.167396053969,-7.185908578481));
#46637=CARTESIAN_POINT('Ctrl Pts',(3.37909718725,2.046454016474,-7.231950245148));
#46638=CARTESIAN_POINT('Ctrl Pts',(3.900753663718,0.6247986664056,-7.277991911815));
#46639=CARTESIAN_POINT('Ctrl Pts',(3.849232882712,-0.8886597582904,-7.324033578481));
#46640=CARTESIAN_POINT('Ctrl Pts',(3.232057337464,-2.271560538139,-7.370075245148));
#46641=CARTESIAN_POINT('Ctrl Pts',(2.504083143683,-2.97090733339,-7.400769689593));
#46642=CARTESIAN_POINT('Ctrl Pts',(2.087596035333,-3.239314958832,-7.416116911815));
#46643=CARTESIAN_POINT('Ctrl Pts',(0.4620124040095,-3.657204758643,-4.566130878679));
#46644=CARTESIAN_POINT('Ctrl Pts',(-0.008203877497198,-3.716606889221,-4.581478100901));
#46645=CARTESIAN_POINT('Ctrl Pts',(-0.9716304726375,-3.65175497376,-4.612172545346));
#46646=CARTESIAN_POINT('Ctrl Pts',(-2.274156201548,-3.017898422626,-4.658214212012));
#46647=CARTESIAN_POINT('Ctrl Pts',(-3.242468351686,-1.94057820163,-4.704255878679));
#46648=CARTESIAN_POINT('Ctrl Pts',(-3.734334802272,-0.5781055559897,-4.750297545346));
#46649=CARTESIAN_POINT('Ctrl Pts',(-3.677464795723,0.8693158916029,-4.796339212012));
#46650=CARTESIAN_POINT('Ctrl Pts',(-3.080218866387,2.188997577561,-4.842380878679));
#46651=CARTESIAN_POINT('Ctrl Pts',(-2.030356921569,3.187021993332,-4.888422545346));
#46652=CARTESIAN_POINT('Ctrl Pts',(-0.6821488302275,3.716736663046,-4.934464212013));
#46653=CARTESIAN_POINT('Ctrl Pts',(0.7662960939803,3.700303872116,-4.980505878679));
#46654=CARTESIAN_POINT('Ctrl Pts',(2.102139367575,3.140138297301,-5.026547545346));
#46655=CARTESIAN_POINT('Ctrl Pts',(3.129088527441,2.11855220272,-5.072589212013));
#46656=CARTESIAN_POINT('Ctrl Pts',(3.696240850532,0.7856602462946,-5.118630878679));
#46657=CARTESIAN_POINT('Ctrl Pts',(3.720257421874,-0.6626787780505,-5.164672545346));
#46658=CARTESIAN_POINT('Ctrl Pts',(3.197609180605,-2.013641968167,-5.210714212013));
#46659=CARTESIAN_POINT('Ctrl Pts',(2.20509549047,-3.068715093613,-5.256755878679));
#46660=CARTESIAN_POINT('Ctrl Pts',(0.8885590308471,-3.672862820275,-5.302797545346));
#46661=CARTESIAN_POINT('Ctrl Pts',(-0.5585447258702,-3.737310026886,-5.348839212013));
#46662=CARTESIAN_POINT('Ctrl Pts',(-1.92357439113,-3.252586664433,-5.394880878679));
#46663=CARTESIAN_POINT('Ctrl Pts',(-3.005948768117,-2.289919311093,-5.440922545346));
#46664=CARTESIAN_POINT('Ctrl Pts',(-3.646620802058,-0.9907649437943,-5.486964212013));
#46665=CARTESIAN_POINT('Ctrl Pts',(-3.751448389963,0.4539751373136,-5.533005878679));
#46666=CARTESIAN_POINT('Ctrl Pts',(-3.30502787902,1.832006868644,-5.579047545346));
#46667=CARTESIAN_POINT('Ctrl Pts',(-2.372957521519,2.940838494192,-5.625089212013));
#46668=CARTESIAN_POINT('Ctrl Pts',(-1.092198288041,3.617535258634,-5.671130878679));
#46669=CARTESIAN_POINT('Ctrl Pts',(0.3490515526009,3.762661486433,-5.717172545346));
#46670=CARTESIAN_POINT('Ctrl Pts',(1.739010802311,3.354891932284,-5.763214212013));
#46671=CARTESIAN_POINT('Ctrl Pts',(2.873435042872,2.454145371051,-5.809255878679));
#46672=CARTESIAN_POINT('Ctrl Pts',(3.585628870032,1.192779968917,-5.855297545346));
#46673=CARTESIAN_POINT('Ctrl Pts',(3.770940572659,-0.2438557879871,-5.901339212013));
#46674=CARTESIAN_POINT('Ctrl Pts',(3.402139941737,-1.644658707665,-5.947380878679));
#46675=CARTESIAN_POINT('Ctrl Pts',(2.533419551845,-2.803790973341,-5.993422545346));
#46676=CARTESIAN_POINT('Ctrl Pts',(1.292431555853,-3.550926515896,-6.039464212013));
#46677=CARTESIAN_POINT('Ctrl Pts',(-0.1384698719652,-3.776279192858,-6.085505878679));
#46678=CARTESIAN_POINT('Ctrl Pts',(-1.549024157631,-3.446735064802,-6.131547545346));
#46679=CARTESIAN_POINT('Ctrl Pts',(-2.731960591949,-2.610718248279,-6.177589212013));
#46680=CARTESIAN_POINT('Ctrl Pts',(-3.513455256077,-1.391075343539,-6.223630878679));
#46681=CARTESIAN_POINT('Ctrl Pts',(-3.778673184137,0.03297598130244,-6.269672545346));
#46682=CARTESIAN_POINT('Ctrl Pts',(-3.488642527544,1.452181725154,-6.315714212013));
#46683=CARTESIAN_POINT('Ctrl Pts',(-2.685981185156,2.657999909866,-6.361755878679));
#46684=CARTESIAN_POINT('Ctrl Pts',(-1.488634412516,3.473244309537,-6.407797545346));
#46685=CARTESIAN_POINT('Ctrl Pts',(-0.07254362303861,3.778120679731,-6.453839212012));
#46686=CARTESIAN_POINT('Ctrl Pts',(1.354206925051,3.527829651783,-6.499880878679));
#46687=CARTESIAN_POINT('Ctrl Pts',(2.581966599408,2.7591496747,-6.545922545346));
#46688=CARTESIAN_POINT('Ctrl Pts',(3.430325031562,1.585032689158,-6.591964212013));
#46689=CARTESIAN_POINT('Ctrl Pts',(3.774622110468,0.1780066600445,-6.638005878679));
#46690=CARTESIAN_POINT('Ctrl Pts',(3.56426588058,-1.255176155123,-6.684047545346));
#46691=CARTESIAN_POINT('Ctrl Pts',(2.830166662326,-2.503919949063,-6.730089212013));
#46692=CARTESIAN_POINT('Ctrl Pts',(1.680195004987,-3.384730889313,-6.776130878679));
#46693=CARTESIAN_POINT('Ctrl Pts',(0.2833308928114,-3.768180204427,-6.822172545346));
#46694=CARTESIAN_POINT('Ctrl Pts',(-1.155166636586,-3.597922802058,-6.868214212013));
#46695=CARTESIAN_POINT('Ctrl Pts',(-2.423920817265,-2.898976771123,-6.914255878679));
#46696=CARTESIAN_POINT('Ctrl Pts',(-3.336497435721,-1.774047155286,-6.960297545346));
#46697=CARTESIAN_POINT('Ctrl Pts',(-3.758799984856,-0.3884341926996,-7.006339212013));
#46698=CARTESIAN_POINT('Ctrl Pts',(-3.6287741714,1.054256353961,-7.052380878679));
#46699=CARTESIAN_POINT('Ctrl Pts',(-2.965526345649,2.342031584525,-7.098422545346));
#46700=CARTESIAN_POINT('Ctrl Pts',(-1.866515954698,3.285662283295,-7.144464212013));
#46701=CARTESIAN_POINT('Ctrl Pts',(-0.4932346117968,3.746488760516,-7.190505878679));
#46702=CARTESIAN_POINT('Ctrl Pts',(0.9525240256962,3.656795952728,-7.236547545346));
#46703=CARTESIAN_POINT('Ctrl Pts',(2.258315987503,3.029763413827,-7.282589212013));
#46704=CARTESIAN_POINT('Ctrl Pts',(3.232265512507,1.957529592619,-7.328630878679));
#46705=CARTESIAN_POINT('Ctrl Pts',(3.731254486433,0.5976493334679,-7.374672545346));
#46706=CARTESIAN_POINT('Ctrl Pts',(3.681972434336,-0.8500448877034,-7.420714212013));
#46707=CARTESIAN_POINT('Ctrl Pts',(3.091614975073,-2.172854576276,-7.466755878679));
#46708=CARTESIAN_POINT('Ctrl Pts',(2.395273393235,-2.841812703939,-7.497450323124));
#46709=CARTESIAN_POINT('Ctrl Pts',(1.996883870199,-3.098557231525,-7.512797545346));
#46710=CARTESIAN_POINT('Ctrl Pts',(0.4410246309536,-3.491069428017,-4.66281151221));
#46711=CARTESIAN_POINT('Ctrl Pts',(-0.007831201098047,-3.547773106292,-4.678158734432));
#46712=CARTESIAN_POINT('Ctrl Pts',(-0.9274923506371,-3.485867209753,-4.708853178877));
#46713=CARTESIAN_POINT('Ctrl Pts',(-2.170848424879,-2.880804771784,-4.754894845544));
#46714=CARTESIAN_POINT('Ctrl Pts',(-3.09517319399,-1.85242382625,-4.80093651221));
#46715=CARTESIAN_POINT('Ctrl Pts',(-3.564695695909,-0.5518440355064,-4.846978178877));
#46716=CARTESIAN_POINT('Ctrl Pts',(-3.510409115218,0.8298255998088,-4.893019845544));
#46717=CARTESIAN_POINT('Ctrl Pts',(-2.940294193437,2.08955828983,-4.93906151221));
#46718=CARTESIAN_POINT('Ctrl Pts',(-1.938124180797,3.042245589626,-4.985103178877));
#46719=CARTESIAN_POINT('Ctrl Pts',(-0.6511609504327,3.5478969849,-5.031144845544));
#46720=CARTESIAN_POINT('Ctrl Pts',(0.7314856681681,3.532210684072,-5.07718651221));
#46721=CARTESIAN_POINT('Ctrl Pts',(2.006645775638,2.997491672717,-5.123228178877));
#46722=CARTESIAN_POINT('Ctrl Pts',(2.986943859211,2.022313027209,-5.169269845544));
#46723=CARTESIAN_POINT('Ctrl Pts',(3.528332232803,0.7499701678353,-5.21531151221));
#46724=CARTESIAN_POINT('Ctrl Pts',(3.551257806707,-0.6325753616011,-5.261353178877));
#46725=CARTESIAN_POINT('Ctrl Pts',(3.052351834218,-1.922168535253,-5.307394845544));
#46726=CARTESIAN_POINT('Ctrl Pts',(2.104924925093,-2.929313000944,-5.35343651221));
#46727=CARTESIAN_POINT('Ctrl Pts',(0.8481945836498,-3.506016193067,-5.399478178877));
#46728=CARTESIAN_POINT('Ctrl Pts',(-0.5331717924892,-3.567535765409,-5.445519845544));
#46729=CARTESIAN_POINT('Ctrl Pts',(-1.836192445479,-3.104831863555,-5.49156151221));
#46730=CARTESIAN_POINT('Ctrl Pts',(-2.869397952564,-2.185895465844,-5.537603178877));
#46731=CARTESIAN_POINT('Ctrl Pts',(-3.480966267353,-0.9457576028406,-5.583644845544));
#46732=CARTESIAN_POINT('Ctrl Pts',(-3.581031867039,0.4333524720513,-5.62968651221));
#46733=CARTESIAN_POINT('Ctrl Pts',(-3.154890838399,1.74878454807,-5.675728178877));
#46734=CARTESIAN_POINT('Ctrl Pts',(-2.265161511065,2.807245433975,-5.721769845544));
#46735=CARTESIAN_POINT('Ctrl Pts',(-1.042583148702,3.453201988854,-5.76781151221));
#46736=CARTESIAN_POINT('Ctrl Pts',(0.3331952363912,3.591735587738,-5.813853178877));
#46737=CARTESIAN_POINT('Ctrl Pts',(1.660013001075,3.202489724268,-5.859894845544));
#46738=CARTESIAN_POINT('Ctrl Pts',(2.742903909839,2.342661251476,-5.90593651221));
#46739=CARTESIAN_POINT('Ctrl Pts',(3.422745007318,1.138595719585,-5.951978178877));
#46740=CARTESIAN_POINT('Ctrl Pts',(3.599638581068,-0.2327781851084,-5.998019845544));
#46741=CARTESIAN_POINT('Ctrl Pts',(3.247591404983,-1.569947025876,-6.04406151221));
#46742=CARTESIAN_POINT('Ctrl Pts',(2.418334255113,-2.676423551744,-6.090103178877));
#46743=CARTESIAN_POINT('Ctrl Pts',(1.233720447776,-3.389619072185,-6.136144845544));
#46744=CARTESIAN_POINT('Ctrl Pts',(-0.1321796203991,-3.604734684513,-6.18218651221));
#46745=CARTESIAN_POINT('Ctrl Pts',(-1.478656853211,-3.290160711611,-6.228228178877));
#46746=CARTESIAN_POINT('Ctrl Pts',(-2.607856199071,-2.492121514442,-6.274269845544));
#46747=CARTESIAN_POINT('Ctrl Pts',(-3.353850014061,-1.327883157873,-6.32031151221));
#46748=CARTESIAN_POINT('Ctrl Pts',(-3.607019924283,0.03147798599784,-6.366353178877));
#46749=CARTESIAN_POINT('Ctrl Pts',(-3.330164449886,1.386213668412,-6.412394845544));
#46750=CARTESIAN_POINT('Ctrl Pts',(-2.563965492379,2.537255318581,-6.45843651221));
#46751=CARTESIAN_POINT('Ctrl Pts',(-1.421010424628,3.315465724582,-6.504478178877));
#46752=CARTESIAN_POINT('Ctrl Pts',(-0.06924819399001,3.606492518418,-6.550519845544));
#46753=CARTESIAN_POINT('Ctrl Pts',(1.292689555892,3.367571426097,-6.59656151221));
#46754=CARTESIAN_POINT('Ctrl Pts',(2.464675962715,2.633810167152,-6.642603178877));
#46755=CARTESIAN_POINT('Ctrl Pts',(3.274496134663,1.513029630198,-6.688644845544));
#46756=CARTESIAN_POINT('Ctrl Pts',(3.603152878174,0.1699203763192,-6.73468651221));
#46757=CARTESIAN_POINT('Ctrl Pts',(3.402352471409,-1.198157442941,-6.780728178877));
#46758=CARTESIAN_POINT('Ctrl Pts',(2.701601075983,-2.390174726673,-6.826769845544));
#46759=CARTESIAN_POINT('Ctrl Pts',(1.603869020775,-3.230973191157,-6.87281151221));
#46760=CARTESIAN_POINT('Ctrl Pts',(0.2704600598501,-3.5970036077,-6.918853178877));
#46761=CARTESIAN_POINT('Ctrl Pts',(-1.102691042857,-3.434480464608,-6.964894845544));
#46762=CARTESIAN_POINT('Ctrl Pts',(-2.313809704281,-2.767285357563,-7.01093651221));
#46763=CARTESIAN_POINT('Ctrl Pts',(-3.184930831936,-1.693457762528,-7.056978178877));
#46764=CARTESIAN_POINT('Ctrl Pts',(-3.588049502055,-0.3707888467895,-7.103019845544));
#46765=CARTESIAN_POINT('Ctrl Pts',(-3.463930353097,1.00636479757,-7.14906151221));
#46766=CARTESIAN_POINT('Ctrl Pts',(-2.830811793846,2.235640442297,-7.195103178877));
#46767=CARTESIAN_POINT('Ctrl Pts',(-1.781725994683,3.136404960891,-7.241144845544));
#46768=CARTESIAN_POINT('Ctrl Pts',(-0.4708285118613,3.576297537987,-7.28718651221));
#46769=CARTESIAN_POINT('Ctrl Pts',(0.9092538495968,3.490679192871,-7.333228178877));
#46770=CARTESIAN_POINT('Ctrl Pts',(2.155727782029,2.892130773684,-7.379269845544));
#46771=CARTESIAN_POINT('Ctrl Pts',(3.085433837764,1.868605168765,-7.42531151221));
#46772=CARTESIAN_POINT('Ctrl Pts',(3.561755309148,0.5705000005301,-7.471353178877));
#46773=CARTESIAN_POINT('Ctrl Pts',(3.514711985961,-0.8114300171164,-7.517394845544));
#46774=CARTESIAN_POINT('Ctrl Pts',(2.951172612682,-2.074148614413,-7.56343651221));
#46775=CARTESIAN_POINT('Ctrl Pts',(2.286463642788,-2.712718074487,-7.594130956655));
#46776=CARTESIAN_POINT('Ctrl Pts',(1.906171705064,-2.957799504219,-7.609478178877));
#46777=CARTESIAN_POINT('',(-1.36802931223802,-3.75862971277667,-4.44175420669655));
#46778=CARTESIAN_POINT('',(-1.36802935610884,-3.75862969680846,-5.19157912663668));
#46779=CARTESIAN_POINT('Ctrl Pts',(-1.36802039437616,-3.75860055108868,
-4.4417004147709));
#46780=CARTESIAN_POINT('Ctrl Pts',(-1.54934259720315,-3.69255062029612,
-4.44743516912771));
#46781=CARTESIAN_POINT('Ctrl Pts',(-1.72591270644782,-3.6134218564521,-4.45314749519308));
#46782=CARTESIAN_POINT('Ctrl Pts',(-2.06238627200896,-3.43244958138755,
-4.46452909116531));
#46783=CARTESIAN_POINT('Ctrl Pts',(-2.22197510880567,-3.33140913413749,
-4.47020811100648));
#46784=CARTESIAN_POINT('Ctrl Pts',(-2.67039775514929,-3.00061382058344,
-4.48693544612448));
#46785=CARTESIAN_POINT('Ctrl Pts',(-2.93619045066687,-2.74087836244429,
-4.49776118719158));
#46786=CARTESIAN_POINT('Ctrl Pts',(-3.32094587933198,-2.24473313507897,
-4.51652534385179));
#46787=CARTESIAN_POINT('Ctrl Pts',(-3.45938490375627,-2.02471873790244,
-4.52434738236671));
#46788=CARTESIAN_POINT('Ctrl Pts',(-3.68290281614523,-1.57848021809534,
-4.53919298992134));
#46789=CARTESIAN_POINT('Ctrl Pts',(-3.77092815157509,-1.35492446506356,
-4.54626688100694));
#46790=CARTESIAN_POINT('Ctrl Pts',(-3.9111203086744,-0.877355368442583,
-4.56112310443606));
#46791=CARTESIAN_POINT('Ctrl Pts',(-3.95946409788148,-0.623612474524625,
-4.56890506844228));
#46792=CARTESIAN_POINT('Ctrl Pts',(-4.00582222878401,-0.117779763933944,
-4.5840291674816));
#46793=CARTESIAN_POINT('Ctrl Pts',(-4.00537282225662,0.132956592148152,
-4.59140521803478));
#46794=CARTESIAN_POINT('Ctrl Pts',(-3.95717640564138,0.637870792459528,
-4.60653661088045));
#46795=CARTESIAN_POINT('Ctrl Pts',(-3.90804180281148,0.890569392092889,
-4.61429431867432));
#46796=CARTESIAN_POINT('Ctrl Pts',(-3.76233568622444,1.38119307228273,-4.62954027014657));
#46797=CARTESIAN_POINT('Ctrl Pts',(-3.66671564796724,1.61808381901511,-4.6370525954201));
#46798=CARTESIAN_POINT('Ctrl Pts',(-3.44683563797407,2.04174570453694,-4.65128932926735));
#46799=CARTESIAN_POINT('Ctrl Pts',(-3.32795075461521,2.23030869406375,-4.65801151888381));
#46800=CARTESIAN_POINT('Ctrl Pts',(-3.11488696706555,2.51264969004533,-4.66857772675018));
#46801=CARTESIAN_POINT('Ctrl Pts',(-3.03104639549336,2.61309949615091,-4.67245981466471));
#46802=CARTESIAN_POINT('Ctrl Pts',(-2.76702348189746,2.89980230975733,-4.68402679092864));
#46803=CARTESIAN_POINT('Ctrl Pts',(-2.57297416693329,3.07355090652908,-4.69171991493211));
#46804=CARTESIAN_POINT('Ctrl Pts',(-2.15293080174829,3.381235303862,-4.70737436130896));
#46805=CARTESIAN_POINT('Ctrl Pts',(-1.92789479525138,3.51419071409789,-4.71514797546484));
#46806=CARTESIAN_POINT('Ctrl Pts',(-1.45736426369289,3.73380167561811,-4.7305573131301));
#46807=CARTESIAN_POINT('Ctrl Pts',(-1.21209415691628,3.82069058044626,-4.73824828416753));
#46808=CARTESIAN_POINT('Ctrl Pts',(-0.707017424571773,3.94561402719561,
-4.7538939255643));
#46809=CARTESIAN_POINT('Ctrl Pts',(-0.448488883432865,3.98309040011465,
-4.76165606365684));
#46810=CARTESIAN_POINT('Ctrl Pts',(0.336804092028381,4.02011287173604,-4.78498496689132));
#46811=CARTESIAN_POINT('Ctrl Pts',(0.859994522360031,3.94156082988392,-4.80064435867064));
#46812=CARTESIAN_POINT('Ctrl Pts',(1.85025226377309,3.5849168365716,-4.83187570141402));
#46813=CARTESIAN_POINT('Ctrl Pts',(2.30357138893829,3.31188808767728,-4.84753994308384));
#46814=CARTESIAN_POINT('Ctrl Pts',(3.08187051358349,2.6033735312351,-4.87877043664423));
#46815=CARTESIAN_POINT('Ctrl Pts',(3.39594107651066,2.17767785925985,-4.89442864532868));
#46816=CARTESIAN_POINT('Ctrl Pts',(3.73051023029279,1.4661277116197,-4.9177611077362));
#46817=CARTESIAN_POINT('Ctrl Pts',(3.81832167123335,1.21993708328814,-4.92552839839978));
#46818=CARTESIAN_POINT('Ctrl Pts',(3.94409941527293,0.714821941134461,-4.94118109301224));
#46819=CARTESIAN_POINT('Ctrl Pts',(3.98197372209973,0.457289881862814,-4.94887423797372));
#46820=CARTESIAN_POINT('Ctrl Pts',(4.00781859492935,-0.0615669812030529,
-4.96429090075327));
#46821=CARTESIAN_POINT('Ctrl Pts',(3.9954657396674,-0.322795341644,-4.97206975219878));
#46822=CARTESIAN_POINT('Ctrl Pts',(3.91975475474618,-0.838118779766908,
-4.98772905643859));
#46823=CARTESIAN_POINT('Ctrl Pts',(3.85683682656876,-1.0909152128301,-4.99542255647908));
#46824=CARTESIAN_POINT('Ctrl Pts',(3.72674843469839,-1.45838615776341,-5.00699162303596));
#46825=CARTESIAN_POINT('Ctrl Pts',(3.67711659488106,-1.57948047247824,-5.01087475438419));
#46826=CARTESIAN_POINT('Ctrl Pts',(3.5273237750208,-1.89927756380344,-5.02142463741197));
#46827=CARTESIAN_POINT('Ctrl Pts',(3.41652238300875,-2.09200988761366,-5.02812865740639));
#46828=CARTESIAN_POINT('Ctrl Pts',(3.14470166249094,-2.48482176617446,-5.04237602217406));
#46829=CARTESIAN_POINT('Ctrl Pts',(2.97934589921149,-2.68083227463917,-5.04991664274165));
#46830=CARTESIAN_POINT('Ctrl Pts',(2.61316026267878,-3.0392638165989,-5.06518203670961));
#46831=CARTESIAN_POINT('Ctrl Pts',(2.41298178294807,-3.20053828557141,-5.07292901109072));
#46832=CARTESIAN_POINT('Ctrl Pts',(1.98803127630066,-3.47983381113735,-5.08809851764534));
#46833=CARTESIAN_POINT('Ctrl Pts',(1.76500032892612,-3.59806928254064,-5.09552353347747));
#46834=CARTESIAN_POINT('Ctrl Pts',(1.29476897682159,-3.79336432465765,-5.11068617323473));
#46835=CARTESIAN_POINT('Ctrl Pts',(1.04821759264496,-3.86879850787193,-5.11845440852111));
#46836=CARTESIAN_POINT('Ctrl Pts',(0.443462743860844,-3.99128966747531,
-5.13686839940374));
#46837=CARTESIAN_POINT('Ctrl Pts',(0.0815921899009596,-4.01521472860259,
-5.14744800540222));
#46838=CARTESIAN_POINT('Ctrl Pts',(-0.46156966433257,-3.97754005871251,
-5.16380287393384));
#46839=CARTESIAN_POINT('Ctrl Pts',(-0.644462573517245,-3.95198255439727,
-5.16934980978426));
#46840=CARTESIAN_POINT('Ctrl Pts',(-1.0095357189814,-3.87487188232507,-5.18046212852935));
#46841=CARTESIAN_POINT('Ctrl Pts',(-1.19104591981548,-3.8229612527995,-5.18603683717925));
#46842=CARTESIAN_POINT('Ctrl Pts',(-1.36801744281564,-3.75860162536828,
-5.1916329185624));
#46843=CARTESIAN_POINT('Ctrl Pts',(-1.3680167762483,-3.75859993758318,-5.19163396445895));
#46844=CARTESIAN_POINT('Ctrl Pts',(-1.52459617763929,-3.70157102288258,
-5.19663239427401));
#46845=CARTESIAN_POINT('Ctrl Pts',(-1.67763499677768,-3.63478957023376,
-5.20164763837071));
#46846=CARTESIAN_POINT('Ctrl Pts',(-1.9724037483695,-3.48366095352311,-5.21156248080557));
#46847=CARTESIAN_POINT('Ctrl Pts',(-2.11391003538115,-3.39971150035342,
-5.21643325110857));
#46848=CARTESIAN_POINT('Ctrl Pts',(-2.51519738783286,-3.12668384635704,
-5.23079642370571));
#46849=CARTESIAN_POINT('Ctrl Pts',(-2.75776227640788,-2.91461075882842,
-5.24042285890803));
#46850=CARTESIAN_POINT('Ctrl Pts',(-3.11317232084341,-2.52027193308931,
-5.25633917223062));
#46851=CARTESIAN_POINT('Ctrl Pts',(-3.24179690154522,-2.35266091526733,
-5.26258710786489));
#46852=CARTESIAN_POINT('Ctrl Pts',(-3.49709704348102,-1.95866745942865,
-5.27648832154417));
#46853=CARTESIAN_POINT('Ctrl Pts',(-3.61609130191531,-1.72870855025888,
-5.28422785733577));
#46854=CARTESIAN_POINT('Ctrl Pts',(-3.80627593895292,-1.25493784223009,
-5.29955595510452));
#46855=CARTESIAN_POINT('Ctrl Pts',(-3.8781817538229,-1.01169864197555,-5.30707268198896));
#46856=CARTESIAN_POINT('Ctrl Pts',(-3.97577832395145,-0.509299016663343,
-5.32222423663731));
#46857=CARTESIAN_POINT('Ctrl Pts',(-4.00018647090875,-0.251353389346759,
-5.32996516501829));
#46858=CARTESIAN_POINT('Ctrl Pts',(-3.99941282800716,0.259916502965717,
-5.34531669247299));
#46859=CARTESIAN_POINT('Ctrl Pts',(-3.97504126814118,0.512996707439322,
-5.35285546694779));
#46860=CARTESIAN_POINT('Ctrl Pts',(-3.85237700186971,1.14468907468732,-5.37190443323698));
#46861=CARTESIAN_POINT('Ctrl Pts',(-3.72197755324421,1.51518481176753,-5.38367582700348));
#46862=CARTESIAN_POINT('Ctrl Pts',(-3.42171503308643,2.08767016397984,-5.40294896079497));
#46863=CARTESIAN_POINT('Ctrl Pts',(-3.28008651051313,2.30373402361474,-5.41050564496186));
#46864=CARTESIAN_POINT('Ctrl Pts',(-2.95281280124014,2.71086590418969,-5.42613976962702));
#46865=CARTESIAN_POINT('Ctrl Pts',(-2.76702159128311,2.90033262756753,-5.43411158232797));
#46866=CARTESIAN_POINT('Ctrl Pts',(-2.46652560831014,3.15151482798791,-5.44577942231872));
#46867=CARTESIAN_POINT('Ctrl Pts',(-2.36491747442529,3.22846771183613,-5.4495401120054));
#46868=CARTESIAN_POINT('Ctrl Pts',(-1.94381052700404,3.51674079037441,-5.46465273838207));
#46869=CARTESIAN_POINT('Ctrl Pts',(-1.59724890420419,3.68683278071615,-5.4762334902682));
#46870=CARTESIAN_POINT('Ctrl Pts',(-1.11260713984251,3.84421077592591,-5.49142073137437));
#46871=CARTESIAN_POINT('Ctrl Pts',(-0.989346965118392,3.87777061807205,
-5.49519140977438));
#46872=CARTESIAN_POINT('Ctrl Pts',(-0.48788725002256,3.98875297609574,-5.51039798290914));
#46873=CARTESIAN_POINT('Ctrl Pts',(-0.0998840500225523,4.01698241598383,
-5.52206340540215));
#46874=CARTESIAN_POINT('Ctrl Pts',(0.541553511551181,3.9715669702806,-5.54123186334516));
#46875=CARTESIAN_POINT('Ctrl Pts',(0.796495603625449,3.92833974663983,-5.54879644134867));
#46876=CARTESIAN_POINT('Ctrl Pts',(1.3008289479688,3.79153197552046,-5.56443837277499));
#46877=CARTESIAN_POINT('Ctrl Pts',(1.54882785835396,3.69722503234154,-5.57240883341697));
#46878=CARTESIAN_POINT('Ctrl Pts',(1.89921194033021,3.52260745940935,-5.58406949732348));
#46879=CARTESIAN_POINT('Ctrl Pts',(2.01032628479411,3.46040397279558,-5.58782611686486));
#46880=CARTESIAN_POINT('Ctrl Pts',(2.44205040257394,3.19081613267549,-5.60290025125967));
#46881=CARTESIAN_POINT('Ctrl Pts',(2.73594967962277,2.94238494043527,-5.61444615201412));
#46882=CARTESIAN_POINT('Ctrl Pts',(3.07387903455474,2.56263769339478,-5.62959619280945));
#46883=CARTESIAN_POINT('Ctrl Pts',(3.15408797273173,2.46325642878526,-5.63336560536742));
#46884=CARTESIAN_POINT('Ctrl Pts',(3.38181256332884,2.15160932363914,-5.64479408180919));
#46885=CARTESIAN_POINT('Ctrl Pts',(3.51351655055612,1.9286688339332,-5.65253364414412));
#46886=CARTESIAN_POINT('Ctrl Pts',(3.72998420409793,1.4662368945807,-5.66786396860653));
#46887=CARTESIAN_POINT('Ctrl Pts',(3.81542441089416,1.22735248319645,-5.67538288269108));
#46888=CARTESIAN_POINT('Ctrl Pts',(3.94102102926835,0.731136667957038,-5.69053657193643));
#46889=CARTESIAN_POINT('Ctrl Pts',(3.97983677196199,0.474949937533666,-5.69827764011206));
#46890=CARTESIAN_POINT('Ctrl Pts',(4.00769347520972,-0.0356116245477114,
-5.71363073144215));
#46891=CARTESIAN_POINT('Ctrl Pts',(3.9975257069734,-0.289698829082997,-5.72117093343997));
#46892=CARTESIAN_POINT('Ctrl Pts',(3.92812752775653,-0.797572025267891,
-5.73634483642131));
#46893=CARTESIAN_POINT('Ctrl Pts',(3.86816682449722,-1.04978870033432,-5.74408698466635));
#46894=CARTESIAN_POINT('Ctrl Pts',(3.70261992673624,-1.53416648463589,-5.75945760919759));
#46895=CARTESIAN_POINT('Ctrl Pts',(3.59782540191802,-1.76635316566549,-5.76701419549071));
#46896=CARTESIAN_POINT('Ctrl Pts',(3.34287429023877,-2.21169068286263,-5.78220371996438));
#46897=CARTESIAN_POINT('Ctrl Pts',(3.19268979435998,-2.42313361991924,-5.7899466526353));
#46898=CARTESIAN_POINT('Ctrl Pts',(2.85735490357643,-2.81046749263772,-5.80533084590177));
#46899=CARTESIAN_POINT('Ctrl Pts',(2.67289578558032,-2.98666099838215,-5.81290010971133));
#46900=CARTESIAN_POINT('Ctrl Pts',(2.1642681873338,-3.38662787238639,-5.83205224148432));
#46901=CARTESIAN_POINT('Ctrl Pts',(1.82075453294885,-3.58271215277965,-5.84390150196588));
#46902=CARTESIAN_POINT('Ctrl Pts',(1.21643196960817,-3.81925402722105,-5.86325194063489));
#46903=CARTESIAN_POINT('Ctrl Pts',(0.968030972362526,-3.88960136599096,
-5.87080284188523));
#46904=CARTESIAN_POINT('Ctrl Pts',(0.454171773558271,-3.98266811030524,
-5.8864311843829));
#46905=CARTESIAN_POINT('Ctrl Pts',(0.189647694887073,-4.00404421823235,
-5.8944039810315));
#46906=CARTESIAN_POINT('Ctrl Pts',(-0.3334185648329,-3.99446656653653,-5.90999161466257));
#46907=CARTESIAN_POINT('Ctrl Pts',(-0.590853825580882,-3.96451728937445,
-5.91757656825456));
#46908=CARTESIAN_POINT('Ctrl Pts',(-1.10209122846833,-3.85398501839706,
-5.93323826433512));
#46909=CARTESIAN_POINT('Ctrl Pts',(-1.35457594056273,-3.77272824853405,
-5.94120524380203));
#46910=CARTESIAN_POINT('Ctrl Pts',(-1.77075753827486,-3.59168027698949,
-5.95471659289937));
#46911=CARTESIAN_POINT('Ctrl Pts',(-1.93915946751059,-3.50362800106389,
-5.96029162353956));
#46912=CARTESIAN_POINT('Ctrl Pts',(-2.21205485324292,-3.33508683258783,
-5.96984947866373));
#46913=CARTESIAN_POINT('Ctrl Pts',(-2.31990375583759,-3.26092839606414,
-5.9737702070383));
#46914=CARTESIAN_POINT('Ctrl Pts',(-2.6301565877348,-3.02452409995926,-5.98548165134658));
#46915=CARTESIAN_POINT('Ctrl Pts',(-2.82134464511646,-2.84728377151697,
-5.9932720609891));
#46916=CARTESIAN_POINT('Ctrl Pts',(-3.16682767687751,-2.45742090293799,
-6.00869433715144));
#46917=CARTESIAN_POINT('Ctrl Pts',(-3.32004506728904,-2.24581849689792,
-6.01643731867248));
#46918=CARTESIAN_POINT('Ctrl Pts',(-3.58251530840628,-1.79748282676246,
-6.03203711468279));
#46919=CARTESIAN_POINT('Ctrl Pts',(-3.69184159328838,-1.56115840039459,
-6.03981172763717));
#46920=CARTESIAN_POINT('Ctrl Pts',(-3.86307243977381,-1.06969754939593,
-6.055217035039));
#46921=CARTESIAN_POINT('Ctrl Pts',(-3.92434285512731,-0.815931314990128,
-6.06296225403942));
#46922=CARTESIAN_POINT('Ctrl Pts',(-4.03406563442041,-0.037214853224006,
-6.08657768116259));
#46923=CARTESIAN_POINT('Ctrl Pts',(-4.00430017251761,0.491396238184421,
-6.10188288702623));
#46924=CARTESIAN_POINT('Ctrl Pts',(-3.74064529529872,1.51094508957726,-6.13350865285382));
#46925=CARTESIAN_POINT('Ctrl Pts',(-3.51050440416036,1.98791707408525,-6.14881710089216));
#46926=CARTESIAN_POINT('Ctrl Pts',(-2.87658037467787,2.82858535128957,-6.18043719471254));
#46927=CARTESIAN_POINT('Ctrl Pts',(-2.48146635415407,3.18076522952212,-6.19573752053965));
#46928=CARTESIAN_POINT('Ctrl Pts',(-1.80808528881573,3.57693292985488,-6.21919924901615));
#46929=CARTESIAN_POINT('Ctrl Pts',(-1.57602875290289,3.68525790641758,-6.22680560757718));
#46930=CARTESIAN_POINT('Ctrl Pts',(-1.09046514191568,3.85715392422301,-6.24205021209597));
#46931=CARTESIAN_POINT('Ctrl Pts',(-0.838128636157874,3.9195341748809,-6.2498027116221));
#46932=CARTESIAN_POINT('Ctrl Pts',(-0.324784493721326,3.99508605519258,
-6.26538453238125));
#46933=CARTESIAN_POINT('Ctrl Pts',(-0.0639985411799379,4.00792889648622,
-6.27313412863224));
#46934=CARTESIAN_POINT('Ctrl Pts',(0.455831514449376,3.98235304377092,-6.28853920799261));
#46935=CARTESIAN_POINT('Ctrl Pts',(0.713374235138799,3.9441684530238,-6.29631043639614));
#46936=CARTESIAN_POINT('Ctrl Pts',(1.21755827403787,3.81889215063033,-6.3119106595662));
#46937=CARTESIAN_POINT('Ctrl Pts',(1.4638408333804,3.73160747445902,-6.3196580212283));
#46938=CARTESIAN_POINT('Ctrl Pts',(1.93538621191033,3.51017181965194,-6.33508018020164));
#46939=CARTESIAN_POINT('Ctrl Pts',(2.15936014956644,3.3767799996088,-6.34286768747215));
#46940=CARTESIAN_POINT('Ctrl Pts',(2.47370387509418,3.14585174539135,-6.35457938315572));
#46941=CARTESIAN_POINT('Ctrl Pts',(2.57528063181982,3.06331535930681,-6.35850050731362));
#46942=CARTESIAN_POINT('Ctrl Pts',(2.81644751835964,2.84686502890774,-6.36815901024042));
#46943=CARTESIAN_POINT('Ctrl Pts',(2.95056536148859,2.70761623303713,-6.3738297545191));
#46944=CARTESIAN_POINT('Ctrl Pts',(3.242968070882,2.35616404170762,-6.38744184306815));
#46945=CARTESIAN_POINT('Ctrl Pts',(3.39164237499895,2.13648822658386,-6.39540961772807));
#46946=CARTESIAN_POINT('Ctrl Pts',(3.64069060839852,1.67682637413702,-6.41106253356384));
#46947=CARTESIAN_POINT('Ctrl Pts',(3.7413926191674,1.43832135217425,-6.41863869330694));
#46948=CARTESIAN_POINT('Ctrl Pts',(3.89697770694004,0.939097436878513,-6.43422035595438));
#46949=CARTESIAN_POINT('Ctrl Pts',(3.95053109180025,0.679145432974062,-6.44219401913166));
#46950=CARTESIAN_POINT('Ctrl Pts',(4.00503852306483,0.160037776789208,-6.4578136851245));
#46951=CARTESIAN_POINT('Ctrl Pts',(4.00707960659604,-0.0978392793946785,
-6.46535594156364));
#46952=CARTESIAN_POINT('Ctrl Pts',(3.94935809009518,-0.744053604171874,
-6.48470221438685));
#46953=CARTESIAN_POINT('Ctrl Pts',(3.85734458348044,-1.12884509202111,-6.49655343292719));
#46954=CARTESIAN_POINT('Ctrl Pts',(3.6156412195022,-1.72971237807858,-6.51572318010026));
#46955=CARTESIAN_POINT('Ctrl Pts',(3.49789688270283,-1.95656801441268,-6.52330862450278));
#46956=CARTESIAN_POINT('Ctrl Pts',(3.07420677216998,-2.61227115933583,-6.54675135106245));
#46957=CARTESIAN_POINT('Ctrl Pts',(2.70595697537982,-2.99224488648191,-6.56204832520248));
#46958=CARTESIAN_POINT('Ctrl Pts',(1.83958567158901,-3.59042937177047,-6.59366554939926));
#46959=CARTESIAN_POINT('Ctrl Pts',(1.35350869025928,-3.80046903462749,-6.6089719068721));
#46960=CARTESIAN_POINT('Ctrl Pts',(0.323857924712615,-4.02129459570999,
-6.64059730443942));
#46961=CARTESIAN_POINT('Ctrl Pts',(-0.205618287062566,-4.02901476468918,
-6.65590426094551));
#46962=CARTESIAN_POINT('Ctrl Pts',(-0.979034883079649,-3.88684859441061,
-6.67951960433248));
#46963=CARTESIAN_POINT('Ctrl Pts',(-1.22996724620899,-3.81506200049018,
-6.68726999926218));
#46964=CARTESIAN_POINT('Ctrl Pts',(-1.71359054806626,-3.62359490712295,
-6.70266480560325));
#46965=CARTESIAN_POINT('Ctrl Pts',(-1.94493551396776,-3.50464134143606,
-6.71042605173161));
#46966=CARTESIAN_POINT('Ctrl Pts',(-2.38168882276234,-3.22394798047734,
-6.72601655674101));
#46967=CARTESIAN_POINT('Ctrl Pts',(-2.58670753680856,-3.06212275004188,
-6.73376526482012));
#46968=CARTESIAN_POINT('Ctrl Pts',(-2.96175735836674,-2.70092027443588,
-6.74917855593458));
#46969=CARTESIAN_POINT('Ctrl Pts',(-3.13080861264775,-2.5026913412351,-6.75695767350024));
#46970=CARTESIAN_POINT('Ctrl Pts',(-3.35408055590606,-2.18305165860493,
-6.76866529572382));
#46971=CARTESIAN_POINT('Ctrl Pts',(-3.42370238331577,-2.07224527451541,
-6.77258657284991));
#46972=CARTESIAN_POINT('Ctrl Pts',(-3.58435262239504,-1.786325901136,-6.78236449836579));
#46973=CARTESIAN_POINT('Ctrl Pts',(-3.66795560240138,-1.60768666132749,
-6.78814844247439));
#46974=CARTESIAN_POINT('Ctrl Pts',(-3.83192874197579,-1.17672052423941,
-6.80187824847632));
#46975=CARTESIAN_POINT('Ctrl Pts',(-3.90130361899299,-0.920683776449137,
-6.80984649243886));
#46976=CARTESIAN_POINT('Ctrl Pts',(-3.98775544337577,-0.405152609759138,
-6.82549680080856));
#46977=CARTESIAN_POINT('Ctrl Pts',(-4.00563982581271,-0.146956557846932,
-6.83307024502416));
#46978=CARTESIAN_POINT('Ctrl Pts',(-3.9908900606506,0.375680334170695,-6.84865101421972));
#46979=CARTESIAN_POINT('Ctrl Pts',(-3.95723043335599,0.638961096328632,
-6.85662513993275));
#46980=CARTESIAN_POINT('Ctrl Pts',(-3.84042797784801,1.14761618106337,-6.87224211503868));
#46981=CARTESIAN_POINT('Ctrl Pts',(-3.75874590502152,1.39213689705194,-6.87978169477132));
#46982=CARTESIAN_POINT('Ctrl Pts',(-3.494082173173,1.98580787585089,-6.89916494719082));
#46983=CARTESIAN_POINT('Ctrl Pts',(-3.28138689292828,2.32097973033577,-6.91105332540699));
#46984=CARTESIAN_POINT('Ctrl Pts',(-2.85631112735569,2.81183723359036,-6.9302717397664));
#46985=CARTESIAN_POINT('Ctrl Pts',(-2.67089507302673,2.98829611630492,-6.93787084862123));
#46986=CARTESIAN_POINT('Ctrl Pts',(-2.05651220821157,3.47067870185686,-6.96132757815569));
#46987=CARTESIAN_POINT('Ctrl Pts',(-1.58453026772136,3.71011770819878,-6.97662703430569));
#46988=CARTESIAN_POINT('Ctrl Pts',(-0.570552308223067,3.99372362689401,
-7.00824687910573));
#46989=CARTESIAN_POINT('Ctrl Pts',(-0.0425135651029989,4.03406360844439,
-7.02355492652206));
#46990=CARTESIAN_POINT('Ctrl Pts',(1.00294575768625,3.90766901147879,-7.05518045364007));
#46991=CARTESIAN_POINT('Ctrl Pts',(1.50603691010037,3.74259279021727,-7.07048619951904));
#46992=CARTESIAN_POINT('Ctrl Pts',(2.19110922183819,3.35637086647038,-7.09410318036229));
#46993=CARTESIAN_POINT('Ctrl Pts',(2.40507091361469,3.20674516340418,-7.10185290577662));
#46994=CARTESIAN_POINT('Ctrl Pts',(2.80020366411324,2.86805997546332,-7.11725674565276));
#46995=CARTESIAN_POINT('Ctrl Pts',(2.98033225870797,2.68010786110962,-7.12502675988284));
#46996=CARTESIAN_POINT('Ctrl Pts',(3.3020231442549,2.27222704406893,-7.14062577316418));
#46997=CARTESIAN_POINT('Ctrl Pts',(3.44318468809885,2.05236308725259,-7.14837326832889));
#46998=CARTESIAN_POINT('Ctrl Pts',(3.68018495053807,1.5884768372515,-7.16379425838034));
#46999=CARTESIAN_POINT('Ctrl Pts',(3.77546949052777,1.34584612505591,-7.17158073678445));
#47000=CARTESIAN_POINT('Ctrl Pts',(3.88242319580831,0.970762049803752,-7.18329206091474));
#47001=CARTESIAN_POINT('Ctrl Pts',(3.91213631086002,0.843299989361819,-7.18721324150571));
#47002=CARTESIAN_POINT('Ctrl Pts',(3.97026086590606,0.523763264771169,-7.19689389874605));
#47003=CARTESIAN_POINT('Ctrl Pts',(3.99097361089814,0.330812765971013,-7.20258586806465));
#47004=CARTESIAN_POINT('Ctrl Pts',(4.00652839568716,-0.1268409864058,-7.21622055359675));
#47005=CARTESIAN_POINT('Ctrl Pts',(3.9893015001724,-0.39154413335847,-7.22418862353994));
#47006=CARTESIAN_POINT('Ctrl Pts',(3.90728476653639,-0.88888007669014,-7.23927958026253));
#47007=CARTESIAN_POINT('Ctrl Pts',(3.84710144367332,-1.12121155500227,-7.24631748009599));
#47008=CARTESIAN_POINT('Ctrl Pts',(3.68534768752621,-1.57312408692967,-7.26059183626647));
#47009=CARTESIAN_POINT('Ctrl Pts',(3.58396937038137,-1.79191386936569,-7.26782957759934));
#47010=CARTESIAN_POINT('Ctrl Pts',(3.46394390204312,-1.99990900584449,-7.27503265522596));
#47011=CARTESIAN_POINT('',(-1.2107513073724,-3.3265118775804,-4.70724779054699));
#47012=CARTESIAN_POINT('Ctrl Pts',(-1.21071383810565,-3.32640900566591,
-4.70724779141669));
#47013=CARTESIAN_POINT('Ctrl Pts',(-1.39219287918788,-3.26025710940742,
-4.71376120107113));
#47014=CARTESIAN_POINT('Ctrl Pts',(-1.56825188079738,-3.17927104752986,
-4.72027461072506));
#47015=CARTESIAN_POINT('Ctrl Pts',(-1.73659924449935,-3.08457088033829,
-4.72678802037908));
#47016=CARTESIAN_POINT('Ctrl Pts',(-1.87338108397249,-3.00762721586959,
-4.732080150497));
#47017=CARTESIAN_POINT('Ctrl Pts',(-2.00508361696359,-2.92162011815734,
-4.73737228061497));
#47018=CARTESIAN_POINT('Ctrl Pts',(-2.13042518195858,-2.827169705567,-4.74266441073295));
#47019=CARTESIAN_POINT('Ctrl Pts',(-2.15935060962041,-2.80537311656542,
-4.74388569057664));
#47020=CARTESIAN_POINT('Ctrl Pts',(-2.18793730334398,-2.78312691895196,
-4.74510697042032));
#47021=CARTESIAN_POINT('Ctrl Pts',(-2.21617354772985,-2.76044407979828,
-4.74632825026401));
#47022=CARTESIAN_POINT('Ctrl Pts',(-2.36676494282521,-2.63947047062431,
-4.75284166022567));
#47023=CARTESIAN_POINT('Ctrl Pts',(-2.50737055352154,-2.50609287961651,
-4.75935507018733));
#47024=CARTESIAN_POINT('Ctrl Pts',(-2.63627091172052,-2.36224216903429,
-4.76586848014899));
#47025=CARTESIAN_POINT('Ctrl Pts',(-2.76517126991969,-2.21839145845186,
-4.77238189011066));
#47026=CARTESIAN_POINT('Ctrl Pts',(-2.88238227181575,-2.06404968982843,
-4.77889530007233));
#47027=CARTESIAN_POINT('Ctrl Pts',(-2.98616562034842,-1.90113425254753,
-4.785408710034));
#47028=CARTESIAN_POINT('Ctrl Pts',(-3.0036792827206,-1.87364192353623,-4.78650786191697));
#47029=CARTESIAN_POINT('Ctrl Pts',(-3.02081015796238,-1.84590601958711,
-4.78760701379993));
#47030=CARTESIAN_POINT('Ctrl Pts',(-3.03754976626217,-1.81793603228567,
-4.7887061656829));
#47031=CARTESIAN_POINT('Ctrl Pts',(-3.12000657762367,-1.6801600505903,-4.7941204237616));
#47032=CARTESIAN_POINT('Ctrl Pts',(-3.1929686605663,-1.53670385765163,-4.7995346818403));
#47033=CARTESIAN_POINT('Ctrl Pts',(-3.25592170098541,-1.38899996899466,
-4.804948939919));
#47034=CARTESIAN_POINT('Ctrl Pts',(-3.3316548770961,-1.21131062250045,-4.81146234988067));
#47035=CARTESIAN_POINT('Ctrl Pts',(-3.39291563048331,-1.0274545075206,-4.81797575984233));
#47036=CARTESIAN_POINT('Ctrl Pts',(-3.4388318118105,-0.839831766260492,
-4.824489169804));
#47037=CARTESIAN_POINT('Ctrl Pts',(-3.46293778073547,-0.741329934450789,
-4.82790870630711));
#47038=CARTESIAN_POINT('Ctrl Pts',(-3.48281390249413,-0.641787444045981,
-4.83132824281022));
#47039=CARTESIAN_POINT('Ctrl Pts',(-3.49832847032117,-0.541569860445466,
-4.83474777931332));
#47040=CARTESIAN_POINT('Ctrl Pts',(-3.51236549246657,-0.450896600574981,
-4.83784165277189));
#47041=CARTESIAN_POINT('Ctrl Pts',(-3.52283219794054,-0.359670757793759,
-4.84093552623045));
#47042=CARTESIAN_POINT('Ctrl Pts',(-3.52973959895587,-0.268179901742102,
-4.84402939968901));
#47043=CARTESIAN_POINT('Ctrl Pts',(-3.54428147831359,-0.0755678052264873,
-4.85054280965067));
#47044=CARTESIAN_POINT('Ctrl Pts',(-3.54305196908429,0.118222685023444,
-4.85705621961233));
#47045=CARTESIAN_POINT('Ctrl Pts',(-3.52615816121155,0.3106374510054,-4.86356962957399));
#47046=CARTESIAN_POINT('Ctrl Pts',(-3.51127051610728,0.480202700612879,
-4.86930956320283));
#47047=CARTESIAN_POINT('Ctrl Pts',(-3.48421326830643,0.648717483567016,
-4.87504949683167));
#47048=CARTESIAN_POINT('Ctrl Pts',(-3.44505320963117,0.814376069645967,
-4.8807894304605));
#47049=CARTESIAN_POINT('Ctrl Pts',(-3.43977625339156,0.836699149309945,
-4.88156290679333));
#47050=CARTESIAN_POINT('Ctrl Pts',(-3.4342795483969,0.85897036558526,-4.88233638312617));
#47051=CARTESIAN_POINT('Ctrl Pts',(-3.42856490437154,0.881185686590716,
-4.883109859459));
#47052=CARTESIAN_POINT('Ctrl Pts',(-3.38044213998663,1.06825992144005,-4.88962326942067));
#47053=CARTESIAN_POINT('Ctrl Pts',(-3.31687241555554,1.25134319073251,-4.89613667938233));
#47054=CARTESIAN_POINT('Ctrl Pts',(-3.23893637138191,1.42807546042492,-4.90265008934417));
#47055=CARTESIAN_POINT('Ctrl Pts',(-3.16100032720827,1.60480773011733,-4.909163499306));
#47056=CARTESIAN_POINT('Ctrl Pts',(-3.06868910928958,1.77521130597631,-4.915676909268));
#47057=CARTESIAN_POINT('Ctrl Pts',(-2.96305546573071,1.93693229393157,-4.92219031922984));
#47058=CARTESIAN_POINT('Ctrl Pts',(-2.93796716681119,1.97534150098615,-4.92373727312258));
#47059=CARTESIAN_POINT('Ctrl Pts',(-2.91212788447957,2.01326000353812,-4.92528422701531));
#47060=CARTESIAN_POINT('Ctrl Pts',(-2.88555239687917,2.05065535009337,-4.92683118090804));
#47061=CARTESIAN_POINT('Ctrl Pts',(-2.80023247086108,2.1707121576857,-4.93179763697708));
#47062=CARTESIAN_POINT('Ctrl Pts',(-2.70732368293247,2.28537607124037,-4.93676409304604));
#47063=CARTESIAN_POINT('Ctrl Pts',(-2.60768233598873,2.39383487273625,-4.94173054911501));
#47064=CARTESIAN_POINT('Ctrl Pts',(-2.47700465903675,2.53607646881263,-4.94824395907667));
#47065=CARTESIAN_POINT('Ctrl Pts',(-2.3347360735518,2.66766424466987,-4.95475736903833));
#47066=CARTESIAN_POINT('Ctrl Pts',(-2.18272371894347,2.78683825766546,-4.96127077899999));
#47067=CARTESIAN_POINT('Ctrl Pts',(-2.09246668450921,2.85759759181515,-4.9651381032626));
#47068=CARTESIAN_POINT('Ctrl Pts',(-1.99876997137404,2.92398232168098,-4.96900542752521));
#47069=CARTESIAN_POINT('Ctrl Pts',(-1.90204061354772,2.98560571817767,-4.97287275178782));
#47070=CARTESIAN_POINT('Ctrl Pts',(-1.83585682521188,3.02776944098037,-4.97551883748687));
#47071=CARTESIAN_POINT('Ctrl Pts',(-1.7682533936754,3.06770422962763,-4.97816492318592));
#47072=CARTESIAN_POINT('Ctrl Pts',(-1.69939760621079,3.10534408721984,-4.98081100888498));
#47073=CARTESIAN_POINT('Ctrl Pts',(-1.52990726349332,3.19799559260592,-4.98732441884667));
#47074=CARTESIAN_POINT('Ctrl Pts',(-1.35283221159455,3.27674344861159,-4.99383782880837));
#47075=CARTESIAN_POINT('Ctrl Pts',(-1.1705592811959,3.34065903690989,-5.00035123877007));
#47076=CARTESIAN_POINT('Ctrl Pts',(-0.997400068785245,3.40137882073238,
-5.00653897567983));
#47077=CARTESIAN_POINT('Ctrl Pts',(-0.819528440494076,3.44871677050005,
-5.01272671258958));
#47078=CARTESIAN_POINT('Ctrl Pts',(-0.639037774186981,3.4818430066795,-5.01891444949934));
#47079=CARTESIAN_POINT('Ctrl Pts',(-0.629538187021195,3.48358650718565,
-5.01924012255123));
#47080=CARTESIAN_POINT('Ctrl Pts',(-0.62003134595265,3.48529064171064,-5.01956579560311));
#47081=CARTESIAN_POINT('Ctrl Pts',(-0.61051757907874,3.48695541282214,-5.019891468655));
#47082=CARTESIAN_POINT('Ctrl Pts',(-0.420243733667227,3.52025057396201,
-5.02640487861664));
#47083=CARTESIAN_POINT('Ctrl Pts',(-0.227230723008247,3.53779512210829,
-5.03291828857827));
#47084=CARTESIAN_POINT('Ctrl Pts',(-0.0340855960367684,3.53962915369353,
-5.03943169853991));
#47085=CARTESIAN_POINT('Ctrl Pts',(0.159059530937512,3.54146318527879,-5.04594510850163));
#47086=CARTESIAN_POINT('Ctrl Pts',(0.352360719567761,3.52758887010852,-5.05245851846337));
#47087=CARTESIAN_POINT('Ctrl Pts',(0.543247550769443,3.4980247813142,-5.05897192842508));
#47088=CARTESIAN_POINT('Ctrl Pts',(0.601707228720348,3.48897068837889,-5.06096668021768));
#47089=CARTESIAN_POINT('Ctrl Pts',(0.659939301890289,3.47844500445235,-5.06296143201029));
#47090=CARTESIAN_POINT('Ctrl Pts',(0.717867025561981,3.466448749601,-5.06495618380289));
#47091=CARTESIAN_POINT('Ctrl Pts',(0.849089156932971,3.43927395262494,-5.0694748419719));
#47092=CARTESIAN_POINT('Ctrl Pts',(0.978749296819402,3.40455233357054,-5.07399350014091));
#47093=CARTESIAN_POINT('Ctrl Pts',(1.10602473720318,3.36262936004284,-5.07851215830992));
#47094=CARTESIAN_POINT('Ctrl Pts',(1.28948564313355,3.30219958129296,-5.08502556827163));
#47095=CARTESIAN_POINT('Ctrl Pts',(1.46801104029239,3.22680554536042,-5.09153897823337));
#47096=CARTESIAN_POINT('Ctrl Pts',(1.63924880370262,3.13743299108219,-5.09805238819509));
#47097=CARTESIAN_POINT('Ctrl Pts',(1.75269332737295,3.07822393200914,-5.10236750348195));
#47098=CARTESIAN_POINT('Ctrl Pts',(1.86294511722153,3.01287435802278,-5.1066826187688));
#47099=CARTESIAN_POINT('Ctrl Pts',(1.96928647887088,2.941685021231,-5.11099773405565));
#47100=CARTESIAN_POINT('Ctrl Pts',(2.02346107989141,2.90541828684098,-5.11319602873044));
#47101=CARTESIAN_POINT('Ctrl Pts',(2.07662086897177,2.86763609085749,-5.11539432340522));
#47102=CARTESIAN_POINT('Ctrl Pts',(2.12869278492199,2.82841085585619,-5.11759261808));
#47103=CARTESIAN_POINT('Ctrl Pts',(2.28297862292286,2.71218893195501,-5.12410602804164));
#47104=CARTESIAN_POINT('Ctrl Pts',(2.42770829556085,2.58330600898348,-5.13061943800327));
#47105=CARTESIAN_POINT('Ctrl Pts',(2.56106883516398,2.44357975449348,-5.1371328479649));
#47106=CARTESIAN_POINT('Ctrl Pts',(2.69442937476905,2.30385350000145,-5.14364625792664));
#47107=CARTESIAN_POINT('Ctrl Pts',(2.81643557043219,2.1532649176556,-5.15015966788837));
#47108=CARTESIAN_POINT('Ctrl Pts',(2.92522794721502,1.99364991391056,-5.15667307785009));
#47109=CARTESIAN_POINT('Ctrl Pts',(2.92726781554804,1.99065711605796,-5.15679520496151));
#47110=CARTESIAN_POINT('Ctrl Pts',(2.92930303206135,1.98766115426643,-5.15691733207293));
#47111=CARTESIAN_POINT('Ctrl Pts',(2.9313335845635,1.984662040754,-5.15703945918435));
#47112=CARTESIAN_POINT('Ctrl Pts',(3.03759856727369,1.82770931719371,-5.16343074203457));
#47113=CARTESIAN_POINT('Ctrl Pts',(3.13108925869377,1.66212467796123,-5.16982202488478));
#47114=CARTESIAN_POINT('Ctrl Pts',(3.21084406279643,1.49018936490803,-5.176213307735));
#47115=CARTESIAN_POINT('Ctrl Pts',(3.29212285262701,1.31496864521171,-5.18272671769664));
#47116=CARTESIAN_POINT('Ctrl Pts',(3.35914855060852,1.13313177099434,-5.18924012765827));
#47117=CARTESIAN_POINT('Ctrl Pts',(3.41090884185987,0.947034149938319,-5.19575353761991));
#47118=CARTESIAN_POINT('Ctrl Pts',(3.43031907907144,0.877247081862021,-5.19819608246181));
#47119=CARTESIAN_POINT('Ctrl Pts',(3.4475820095095,0.806861453565564,-5.20063862730372));
#47120=CARTESIAN_POINT('Ctrl Pts',(3.46264250659767,0.736007385494901,-5.20308117214562));
#47121=CARTESIAN_POINT('Ctrl Pts',(3.48774307025223,0.617918517950802,-5.20715203726545));
#47122=CARTESIAN_POINT('Ctrl Pts',(3.50672549247776,0.498528446452136,-5.21122290238527));
#47123=CARTESIAN_POINT('Ctrl Pts',(3.51957889593106,0.378491351196591,-5.21529376750508));
#47124=CARTESIAN_POINT('Ctrl Pts',(3.54014442282263,0.186431238913331,-5.2218071774667));
#47125=CARTESIAN_POINT('Ctrl Pts',(3.54502560134987,-0.00730000610566984,
-5.2283205874283));
#47126=CARTESIAN_POINT('Ctrl Pts',(3.53418198158554,-0.200151998238902,
-5.23483399739009));
#47127=CARTESIAN_POINT('Ctrl Pts',(3.52625261802275,-0.341174423652751,
-5.23959690836843));
#47128=CARTESIAN_POINT('Ctrl Pts',(3.50991175822703,-0.481737410954006,
-5.24435981934687));
#47129=CARTESIAN_POINT('Ctrl Pts',(3.48514125710933,-0.620798210365567,
-5.24912273032526));
#47130=CARTESIAN_POINT('Ctrl Pts',(3.47603742602251,-0.671906826320724,
-5.25087322930883));
#47131=CARTESIAN_POINT('Ctrl Pts',(3.46579506342518,-0.722812536677146,
-5.25262372829238));
#47132=CARTESIAN_POINT('Ctrl Pts',(3.45443274215295,-0.7734670235766,-5.25437422727593));
#47133=CARTESIAN_POINT('Ctrl Pts',(3.41215482182319,-0.961946675768368,
-5.26088763723773));
#47134=CARTESIAN_POINT('Ctrl Pts',(3.35437640811406,-1.1469330851341,-5.26740104719937));
#47135=CARTESIAN_POINT('Ctrl Pts',(3.28203684521707,-1.32602898115537,-5.273914457161));
#47136=CARTESIAN_POINT('Ctrl Pts',(3.20969728232009,-1.50512487717664,-5.28042786712264));
#47137=CARTESIAN_POINT('Ctrl Pts',(3.12278631763227,-1.67835197646303,-5.28694127708427));
#47138=CARTESIAN_POINT('Ctrl Pts',(3.02223197295951,-1.8432806479056,-5.29345468704591));
#47139=CARTESIAN_POINT('Ctrl Pts',(3.01343337877785,-1.85771205267151,-5.294024616184));
#47140=CARTESIAN_POINT('Ctrl Pts',(3.00453044323614,-1.8720797233967,-5.2945945453221));
#47141=CARTESIAN_POINT('Ctrl Pts',(2.9955238080915,-1.8863820172901,-5.2951644744602));
#47142=CARTESIAN_POINT('Ctrl Pts',(2.90159851161271,-2.03553285694236,-5.30110795528383));
#47143=CARTESIAN_POINT('Ctrl Pts',(2.79639484911094,-2.17757303830368,-5.30705143610746));
#47144=CARTESIAN_POINT('Ctrl Pts',(2.68128796199762,-2.31104848987915,-5.31299491693108));
#47145=CARTESIAN_POINT('Ctrl Pts',(2.55514330578951,-2.45732309927445,-5.3195083268927));
#47146=CARTESIAN_POINT('Ctrl Pts',(2.41709243724114,-2.5933320851481,-5.3260217368543));
#47147=CARTESIAN_POINT('Ctrl Pts',(2.26888276917332,-2.71720685314313,-5.33253514681592));
#47148=CARTESIAN_POINT('Ctrl Pts',(2.20311454325284,-2.77217643666326,-5.33542548064808));
#47149=CARTESIAN_POINT('Ctrl Pts',(2.13534527838208,-2.82475626413618,-5.33831581448023));
#47150=CARTESIAN_POINT('Ctrl Pts',(2.06573588820082,-2.874775685197,-5.34120614831239));
#47151=CARTESIAN_POINT('Ctrl Pts',(1.97847948994207,-2.93747576795006,-5.34482922444196));
#47152=CARTESIAN_POINT('Ctrl Pts',(1.8883316623885,-2.99615253300867,-5.34845230057153));
#47153=CARTESIAN_POINT('Ctrl Pts',(1.79571220403399,-3.05061307565962,-5.3520753767011));
#47154=CARTESIAN_POINT('Ctrl Pts',(1.62920493752531,-3.14851988974053,-5.35858878666273));
#47155=CARTESIAN_POINT('Ctrl Pts',(1.45470238311939,-3.23280915686397,-5.36510219662437));
#47156=CARTESIAN_POINT('Ctrl Pts',(1.2745261419347,-3.30242008610374,-5.371615606586));
#47157=CARTESIAN_POINT('Ctrl Pts',(1.13038560964148,-3.3581086515221,-5.37682631790255));
#47158=CARTESIAN_POINT('Ctrl Pts',(0.982599582851898,-3.40440558395331,
-5.3820370292191));
#47159=CARTESIAN_POINT('Ctrl Pts',(0.83240308038325,-3.440741942048,-5.38724774053564));
#47160=CARTESIAN_POINT('Ctrl Pts',(0.794853354755298,-3.44982617672956,
-5.38855043918073));
#47161=CARTESIAN_POINT('Ctrl Pts',(0.757152994147713,-3.45828791657969,
-5.38985313782582));
#47162=CARTESIAN_POINT('Ctrl Pts',(0.719323216056953,-3.46612616198879,
-5.39115583647091));
#47163=CARTESIAN_POINT('Ctrl Pts',(0.530176743543513,-3.5053168880425,-5.39766924643264));
#47164=CARTESIAN_POINT('Ctrl Pts',(0.33781692832025,-3.52891744226118,-5.40418265639437));
#47165=CARTESIAN_POINT('Ctrl Pts',(0.144825265577312,-3.53682450849308,
-5.4106960663561));
#47166=CARTESIAN_POINT('Ctrl Pts',(-0.0481663971628301,-3.54473157472486,
-5.41720947631773));
#47167=CARTESIAN_POINT('Ctrl Pts',(-0.24181388703863,-3.53694580387158,
-5.42372288627936));
#47168=CARTESIAN_POINT('Ctrl Pts',(-0.433530449310566,-3.51334032191244,
-5.430236296241));
#47169=CARTESIAN_POINT('Ctrl Pts',(-0.463486537026677,-3.5096519192008,
-5.4312540292831));
#47170=CARTESIAN_POINT('Ctrl Pts',(-0.493394854987601,-3.50557733750051,
-5.4322717623252));
#47171=CARTESIAN_POINT('Ctrl Pts',(-0.52324531539875,-3.50111615630133,
-5.4332894953673));
#47172=CARTESIAN_POINT('Ctrl Pts',(-0.684435410967214,-3.4770261351111,
-5.43878517228683));
#47173=CARTESIAN_POINT('Ctrl Pts',(-0.843938087347221,-3.44166213854163,
-5.44428084920637));
#47174=CARTESIAN_POINT('Ctrl Pts',(-1.00025566879186,-3.39555923162819,
-5.44977652612591));
#47175=CARTESIAN_POINT('Ctrl Pts',(-1.1855213798375,-3.34091862273664,-5.45628993608763));
#47176=CARTESIAN_POINT('Ctrl Pts',(-1.36633644531483,-3.2711909851405,-5.46280334604936));
#47177=CARTESIAN_POINT('Ctrl Pts',(-1.54029195487117,-3.18722583254678,
-5.46931675601108));
#47178=CARTESIAN_POINT('Ctrl Pts',(-1.62944410370728,-3.1441937158856,-5.47265487675137));
#47179=CARTESIAN_POINT('Ctrl Pts',(-1.71679583817647,-3.09742028661071,
-5.47599299749165));
#47180=CARTESIAN_POINT('Ctrl Pts',(-1.80200661175619,-3.04702677559417,
-5.47933111823193));
#47181=CARTESIAN_POINT('Ctrl Pts',(-1.88306085512836,-2.99909142968991,
-5.48250640745326));
#47182=CARTESIAN_POINT('Ctrl Pts',(-1.96217788986922,-2.94788060262952,
-5.48568169667459));
#47183=CARTESIAN_POINT('Ctrl Pts',(-2.03912504838554,-2.89360083987272,
-5.48885698589592));
#47184=CARTESIAN_POINT('Ctrl Pts',(-2.19696528084021,-2.78225780217885,
-5.49537039585763));
#47185=CARTESIAN_POINT('Ctrl Pts',(-2.34568157844476,-2.65800144637073,
-5.50188380581937));
#47186=CARTESIAN_POINT('Ctrl Pts',(-2.48336853770675,-2.52253489439242,
-5.50839721578109));
#47187=CARTESIAN_POINT('Ctrl Pts',(-2.60298386808918,-2.40484853936279,
-5.51405573049203));
#47188=CARTESIAN_POINT('Ctrl Pts',(-2.71428549057575,-2.27868697184984,
-5.51971424520297));
#47189=CARTESIAN_POINT('Ctrl Pts',(-2.81597612222633,-2.14519893694035,
-5.52537275991391));
#47190=CARTESIAN_POINT('Ctrl Pts',(-2.83133966592628,-2.12503140307353,
-5.52622765516461));
#47191=CARTESIAN_POINT('Ctrl Pts',(-2.84648385104755,-2.10469665766999,
-5.52708255041531));
#47192=CARTESIAN_POINT('Ctrl Pts',(-2.86140601976011,-2.08420004970933,
-5.527937445666));
#47193=CARTESIAN_POINT('Ctrl Pts',(-2.97509737816046,-1.92803727963656,
-5.53445085562764));
#47194=CARTESIAN_POINT('Ctrl Pts',(-3.07588539103572,-1.76250130618686,
-5.54096426558927));
#47195=CARTESIAN_POINT('Ctrl Pts',(-3.16263326328894,-1.58992343651983,
-5.54747767555091));
#47196=CARTESIAN_POINT('Ctrl Pts',(-3.24938113554341,-1.4173455668503,-5.55399108551264));
#47197=CARTESIAN_POINT('Ctrl Pts',(-3.32210027300758,-1.23770469083994,
-5.56050449547437));
#47198=CARTESIAN_POINT('Ctrl Pts',(-3.37963916765126,-1.05330980373386,
-5.56701790543609));
#47199=CARTESIAN_POINT('Ctrl Pts',(-3.39258558113939,-1.01182043435414,
-5.56848344103779));
#47200=CARTESIAN_POINT('Ctrl Pts',(-3.40476309979245,-0.970091329658437,
-5.56994897663948));
#47201=CARTESIAN_POINT('Ctrl Pts',(-3.41615839043217,-0.928149692388579,
-5.57141451224117));
#47202=CARTESIAN_POINT('Ctrl Pts',(-3.45540820147598,-0.783686388225696,
-5.57646238660112));
#47203=CARTESIAN_POINT('Ctrl Pts',(-3.48537682874472,-0.636701514870851,
-5.58151026096109));
#47204=CARTESIAN_POINT('Ctrl Pts',(-3.50597617628425,-0.488430196162447,
-5.58655813532117));
#47205=CARTESIAN_POINT('Ctrl Pts',(-3.53255607623814,-0.297111669702389,
-5.59307154528297));
#47206=CARTESIAN_POINT('Ctrl Pts',(-3.54354418974018,-0.103630424635091,
-5.59958495524494));
#47207=CARTESIAN_POINT('Ctrl Pts',(-3.53875253925765,0.089468803271073,
-5.60609836520674));
#47208=CARTESIAN_POINT('Ctrl Pts',(-3.53596740081211,0.201707391082333,
-5.60988427333219));
#47209=CARTESIAN_POINT('Ctrl Pts',(-3.52784953284791,0.313821101074286,
-5.61367018145759));
#47210=CARTESIAN_POINT('Ctrl Pts',(-3.51436099043,0.425284409474744,-5.61745608958296));
#47211=CARTESIAN_POINT('Ctrl Pts',(-3.50464336839674,0.505586510921572,
-5.62018359141934));
#47212=CARTESIAN_POINT('Ctrl Pts',(-3.49213834393737,0.585551019147991,
-5.62291109325571));
#47213=CARTESIAN_POINT('Ctrl Pts',(-3.47690638446997,0.66499043379555,-5.62563859509208));
#47214=CARTESIAN_POINT('Ctrl Pts',(-3.44053170812434,0.854695704681691,
-5.6321520050537));
#47215=CARTESIAN_POINT('Ctrl Pts',(-3.38860921956519,1.04140602837934,-5.6386654150153));
#47216=CARTESIAN_POINT('Ctrl Pts',(-3.32193574191479,1.22268842298407,-5.64517882497692));
#47217=CARTESIAN_POINT('Ctrl Pts',(-3.25942939273935,1.3926405697123,-5.65128514328716));
#47218=CARTESIAN_POINT('Ctrl Pts',(-3.18394820657006,1.55784068731747,-5.65739146159741));
#47219=CARTESIAN_POINT('Ctrl Pts',(-3.09615376327333,1.71622605567233,-5.66349777990766));
#47220=CARTESIAN_POINT('Ctrl Pts',(-3.09030074626759,1.7267851778631,-5.66390487155914));
#47221=CARTESIAN_POINT('Ctrl Pts',(-3.08439300690686,1.73731401277661,-5.66431196321062));
#47222=CARTESIAN_POINT('Ctrl Pts',(-3.0784309562568,1.74781206796055,-5.6647190548621));
#47223=CARTESIAN_POINT('Ctrl Pts',(-2.98303897276905,1.91577949486414,-5.67123246482373));
#47224=CARTESIAN_POINT('Ctrl Pts',(-2.87375899624301,2.0758403789111,-5.67774587478537));
#47225=CARTESIAN_POINT('Ctrl Pts',(-2.75227553257105,2.22600746165049,-5.684259284747));
#47226=CARTESIAN_POINT('Ctrl Pts',(-2.63079206889909,2.37617454438987,-5.69077269470864));
#47227=CARTESIAN_POINT('Ctrl Pts',(-2.49709140537515,2.51646756267748,-5.69728610467027));
#47228=CARTESIAN_POINT('Ctrl Pts',(-2.35282015491859,2.64491088381421,-5.70379951463191));
#47229=CARTESIAN_POINT('Ctrl Pts',(-2.31044002818164,2.6826415072826,-5.70571284898501));
#47230=CARTESIAN_POINT('Ctrl Pts',(-2.26714849820321,2.71934870346318,-5.70762618333811));
#47231=CARTESIAN_POINT('Ctrl Pts',(-2.222989224079,2.754980745782,-5.70953951769122));
#47232=CARTESIAN_POINT('Ctrl Pts',(-2.11682063965784,2.84064799389807,-5.71413959329984));
#47233=CARTESIAN_POINT('Ctrl Pts',(-2.00563588372431,2.92009993133965,-5.71873966890847));
#47234=CARTESIAN_POINT('Ctrl Pts',(-1.89026706688281,2.99289754536391,-5.7233397445171));
#47235=CARTESIAN_POINT('Ctrl Pts',(-1.72691227343801,3.09597426512039,-5.72985315447873));
#47236=CARTESIAN_POINT('Ctrl Pts',(-1.55515506607057,3.18572418961666,-5.73636656444037));
#47237=CARTESIAN_POINT('Ctrl Pts',(-1.37724999191978,3.26095501036923,-5.742879974402));
#47238=CARTESIAN_POINT('Ctrl Pts',(-1.26161218703416,3.30985483525111,-5.74711367281605));
#47239=CARTESIAN_POINT('Ctrl Pts',(-1.14336967917686,3.35262137178841,-5.7513473712301));
#47240=CARTESIAN_POINT('Ctrl Pts',(-1.02317256118377,3.3889110212635,-5.75558106964415));
#47241=CARTESIAN_POINT('Ctrl Pts',(-0.958450247245203,3.40845183992259,
-5.75786078119174));
#47242=CARTESIAN_POINT('Ctrl Pts',(-0.89316126230264,3.42611482909649,-5.76014049273932));
#47243=CARTESIAN_POINT('Ctrl Pts',(-0.827419800164984,3.44188829366148,
-5.76242020428691));
#47244=CARTESIAN_POINT('Ctrl Pts',(-0.639588539302361,3.48695497823277,
-5.76893361424864));
#47245=CARTESIAN_POINT('Ctrl Pts',(-0.448071840368298,3.51659792381025,
-5.77544702421037));
#47246=CARTESIAN_POINT('Ctrl Pts',(-0.255423787889024,3.53056979807231,
-5.78196043417208));
#47247=CARTESIAN_POINT('Ctrl Pts',(-0.0627757354125469,3.54454167233417,
-5.7884738441337));
#47248=CARTESIAN_POINT('Ctrl Pts',(0.131027743644164,3.54284160663298,-5.7949872540953));
#47249=CARTESIAN_POINT('Ctrl Pts',(0.323385332326859,3.52519811655209,-5.80150066405692));
#47250=CARTESIAN_POINT('Ctrl Pts',(0.515742921012346,3.50755462647096,-5.80801407401864));
#47251=CARTESIAN_POINT('Ctrl Pts',(0.706621482692652,3.47396442994213,-5.81452748398037));
#47252=CARTESIAN_POINT('Ctrl Pts',(0.893511611909647,3.42517311385951,-5.8210408939421));
#47253=CARTESIAN_POINT('Ctrl Pts',(1.08040174112393,3.3763817977776,-5.82755430390373));
#47254=CARTESIAN_POINT('Ctrl Pts',(1.26332731289825,3.31238606054051,-5.83406771386537));
#47255=CARTESIAN_POINT('Ctrl Pts',(1.43982452056484,3.23389875855054,-5.840581123827));
#47256=CARTESIAN_POINT('Ctrl Pts',(1.50380522324394,3.20544690484081,-5.84294225209465));
#47257=CARTESIAN_POINT('Ctrl Pts',(1.56694025449916,3.17509076695823,-5.8453033803623));
#47258=CARTESIAN_POINT('Ctrl Pts',(1.62910723813456,3.14286646338266,-5.84766450862994));
#47259=CARTESIAN_POINT('Ctrl Pts',(1.73843413564225,3.08619678233581,-5.85181679032393));
#47260=CARTESIAN_POINT('Ctrl Pts',(1.84476690245898,3.02374911182526,-5.85596907201792));
#47261=CARTESIAN_POINT('Ctrl Pts',(1.94756203567169,2.95595504167199,-5.8601213537119));
#47262=CARTESIAN_POINT('Ctrl Pts',(2.10880996970625,2.84961096281966,-5.86663476367363));
#47263=CARTESIAN_POINT('Ctrl Pts',(2.26136901605629,2.73010640649609,-5.87314817363537));
#47264=CARTESIAN_POINT('Ctrl Pts',(2.40324259782627,2.59902847899996,-5.87966158359708));
#47265=CARTESIAN_POINT('Ctrl Pts',(2.50521379478413,2.50481662507491,-5.88434307680947));
#47266=CARTESIAN_POINT('Ctrl Pts',(2.60167081814559,2.40461726441304,-5.88902457002185));
#47267=CARTESIAN_POINT('Ctrl Pts',(2.69183711822383,2.2990460910885,-5.89370606323423));
#47268=CARTESIAN_POINT('Ctrl Pts',(2.72712012469975,2.25773499826505,-5.89553797998346));
#47269=CARTESIAN_POINT('Ctrl Pts',(2.76143995124405,2.2156014429839,-5.89736989673269));
#47270=CARTESIAN_POINT('Ctrl Pts',(2.79476729971627,2.17269706292566,-5.89920181348192));
#47271=CARTESIAN_POINT('Ctrl Pts',(2.91326323225658,2.02014983795509,-5.90571522344363));
#47272=CARTESIAN_POINT('Ctrl Pts',(3.01920517514468,1.85787088053258,-5.91222863340537));
#47273=CARTESIAN_POINT('Ctrl Pts',(3.11133748932251,1.68810632525813,-5.91874204336726));
#47274=CARTESIAN_POINT('Ctrl Pts',(3.203469803499,1.51834176998613,-5.92525545332906));
#47275=CARTESIAN_POINT('Ctrl Pts',(3.28180255010409,1.34106980168587,-5.93176886329103));
#47276=CARTESIAN_POINT('Ctrl Pts',(3.34504642056238,1.15855163970423,-5.93828227325283));
#47277=CARTESIAN_POINT('Ctrl Pts',(3.34978975557038,1.14486264848577,-5.938770783606));
#47278=CARTESIAN_POINT('Ctrl Pts',(3.35444815655005,1.1311443095087,-5.93925929395917));
#47279=CARTESIAN_POINT('Ctrl Pts',(3.35902108122167,1.11739759079248,-5.93974780431234));
#47280=CARTESIAN_POINT('Ctrl Pts',(3.41541991061322,0.94785645481421,-5.94577270392095));
#47281=CARTESIAN_POINT('Ctrl Pts',(3.45881608303693,0.773998449359656,-5.95179760352943));
#47282=CARTESIAN_POINT('Ctrl Pts',(3.48894891305953,0.597889911087293,-5.95782250313791));
#47283=CARTESIAN_POINT('Ctrl Pts',(3.52152497042123,0.407502156590185,-5.96433591309964));
#47284=CARTESIAN_POINT('Ctrl Pts',(3.53860724556339,0.214461276056274,-5.97084932306137));
#47285=CARTESIAN_POINT('Ctrl Pts',(3.53986050381078,0.021304435887652,-5.97736273302309));
#47286=CARTESIAN_POINT('Ctrl Pts',(3.54040097332149,-0.061994742963288,
-5.98017165089967));
#47287=CARTESIAN_POINT('Ctrl Pts',(3.53799699077534,-0.145315513407627,
-5.98298056877624));
#47288=CARTESIAN_POINT('Ctrl Pts',(3.53262128868333,-0.22844437121557,-5.98578948665281));
#47289=CARTESIAN_POINT('Ctrl Pts',(3.5255316382462,-0.338077407609597,-5.98949397873787));
#47290=CARTESIAN_POINT('Ctrl Pts',(3.51327303496331,-0.447376576378206,
-5.99319847082294));
#47291=CARTESIAN_POINT('Ctrl Pts',(3.49597098000898,-0.555864346356779,
-5.996902962908));
#47292=CARTESIAN_POINT('Ctrl Pts',(3.46554970375613,-0.746612579979145,
-6.00341637286964));
#47293=CARTESIAN_POINT('Ctrl Pts',(3.41953925747835,-0.934864572484402,
-6.00992978283127));
#47294=CARTESIAN_POINT('Ctrl Pts',(3.35859301744289,-1.11815333279855,-6.01644319279291));
#47295=CARTESIAN_POINT('Ctrl Pts',(3.31059801777636,-1.2624927372481,-6.02157248557216));
#47296=CARTESIAN_POINT('Ctrl Pts',(3.25333356013243,-1.40376624524555,-6.02670177835142));
#47297=CARTESIAN_POINT('Ctrl Pts',(3.18712845076366,-1.54071809177819,-6.03183107113067));
#47298=CARTESIAN_POINT('Ctrl Pts',(3.16926329207835,-1.57767394751018,-6.03321518831314));
#47299=CARTESIAN_POINT('Ctrl Pts',(3.15074717578934,-1.61431513677177,-6.03459930549561));
#47300=CARTESIAN_POINT('Ctrl Pts',(3.13159534362019,-1.65062121645643,-6.03598342267808));
#47301=CARTESIAN_POINT('Ctrl Pts',(3.04147021836802,-1.82147118788974,-6.0424968326397));
#47302=CARTESIAN_POINT('Ctrl Pts',(2.93727842881738,-1.98488223342344,-6.04901024260131));
#47303=CARTESIAN_POINT('Ctrl Pts',(2.82057762917812,-2.13879529781198,-6.05552365256292));
#47304=CARTESIAN_POINT('Ctrl Pts',(2.70387682953718,-2.29270836220275,-6.06203706252464));
#47305=CARTESIAN_POINT('Ctrl Pts',(2.57465211340251,-2.43714224335224,-6.06855047248637));
#47306=CARTESIAN_POINT('Ctrl Pts',(2.43444850641693,-2.57001604546182,-6.0750638824481));
#47307=CARTESIAN_POINT('Ctrl Pts',(2.41429399083976,-2.58911688867116,-6.07600019660831));
#47308=CARTESIAN_POINT('Ctrl Pts',(2.39391298941519,-2.60797845638822,-6.07693651076853));
#47309=CARTESIAN_POINT('Ctrl Pts',(2.37331023111434,-2.62659447705366,-6.07787282492875));
#47310=CARTESIAN_POINT('Ctrl Pts',(2.25059121040597,-2.73747962127514,-6.08344992073017));
#47311=CARTESIAN_POINT('Ctrl Pts',(2.12000384287054,-2.839652015463,-6.08902701653158));
#47312=CARTESIAN_POINT('Ctrl Pts',(1.98297254939446,-2.93225806317012,-6.094604112333));
#47313=CARTESIAN_POINT('Ctrl Pts',(1.82293567289756,-3.04041133417721,-6.10111752229464));
#47314=CARTESIAN_POINT('Ctrl Pts',(1.65409266030275,-3.13553304456699,-6.10763093225627));
#47315=CARTESIAN_POINT('Ctrl Pts',(1.47862930850234,-3.2163003073892,-6.11414434221791));
#47316=CARTESIAN_POINT('Ctrl Pts',(1.390897632601,-3.25668393880083,-6.11740104719877));
#47317=CARTESIAN_POINT('Ctrl Pts',(1.30150905535828,-3.29347875878619,-6.12065775217963));
#47318=CARTESIAN_POINT('Ctrl Pts',(1.21075130737302,-3.32651187758184,-6.12391445716049));
#47319=CARTESIAN_POINT('Ctrl Pts',(1.1199935593875,-3.35954499637758,-6.12717116214136));
#47320=CARTESIAN_POINT('Ctrl Pts',(1.02786668212491,-3.3888163988914,-6.13042786712223));
#47321=CARTESIAN_POINT('Ctrl Pts',(0.934702221409373,-3.414273576702,-6.1336845721031));
#47322=CARTESIAN_POINT('Ctrl Pts',(0.748373299981275,-3.46518793232237,
-6.14019798206473));
#47323=CARTESIAN_POINT('Ctrl Pts',(0.557888991572958,-3.50085067113629,
-6.14671139202637));
#47324=CARTESIAN_POINT('Ctrl Pts',(0.365774049088018,-3.52087018018125,
-6.153224801988));
#47325=CARTESIAN_POINT('Ctrl Pts',(0.20127596813921,-3.53801184952169,-6.15880189778942));
#47326=CARTESIAN_POINT('Ctrl Pts',(0.0355650918612497,-3.54368319654726,
-6.16437899359083));
#47327=CARTESIAN_POINT('Ctrl Pts',(-0.1297187288212,-3.53762251397617,-6.16995608939225));
#47328=CARTESIAN_POINT('Ctrl Pts',(-0.157467504755981,-3.53660501255357,
-6.17089240355247));
#47329=CARTESIAN_POINT('Ctrl Pts',(-0.185204239670332,-3.53525686860412,
-6.17182871771269));
#47330=CARTESIAN_POINT('Ctrl Pts',(-0.212921279681585,-3.53357984669696,
-6.17276503187291));
#47331=CARTESIAN_POINT('Ctrl Pts',(-0.405733107366116,-3.52191375035853,
-6.17927844183464));
#47332=CARTESIAN_POINT('Ctrl Pts',(-0.597565292296506,-3.49433502470254,
-6.18579185179637));
#47333=CARTESIAN_POINT('Ctrl Pts',(-0.785896702128393,-3.45144460505232,
-6.19230526175808));
#47334=CARTESIAN_POINT('Ctrl Pts',(-0.97422811195755,-3.40855418540273,
-6.1988186717197));
#47335=CARTESIAN_POINT('Ctrl Pts',(-1.15908224871662,-3.35034725338159,
-6.2053320816813));
#47336=CARTESIAN_POINT('Ctrl Pts',(-1.33794234485403,-3.27739989599169,
-6.21184549164292));
#47337=CARTESIAN_POINT('Ctrl Pts',(-1.37595059764031,-3.26189838581898,
-6.21322960882539));
#47338=CARTESIAN_POINT('Ctrl Pts',(-1.41368726809313,-3.24573153652599,
-6.21461372600786));
#47339=CARTESIAN_POINT('Ctrl Pts',(-1.4511275397993,-3.22890521124983,-6.21599784319033));
#47340=CARTESIAN_POINT('Ctrl Pts',(-1.58987454601214,-3.16654983423889,
-6.22112713596958));
#47341=CARTESIAN_POINT('Ctrl Pts',(-1.72455052609608,-3.09513693232657,
-6.22625642874884));
#47342=CARTESIAN_POINT('Ctrl Pts',(-1.85409640965779,-3.01541712473751,
-6.2313857215281));
#47343=CARTESIAN_POINT('Ctrl Pts',(-2.01859968229062,-2.91418527636456,
-6.23789913148973));
#47344=CARTESIAN_POINT('Ctrl Pts',(-2.17485177726832,-2.79955082838338,
-6.24441254145137));
#47345=CARTESIAN_POINT('Ctrl Pts',(-2.32076642803647,-2.67298362342837,
-6.250925951413));
#47346=CARTESIAN_POINT('Ctrl Pts',(-2.40375516543355,-2.60099871663665,
-6.25463044349806));
#47347=CARTESIAN_POINT('Ctrl Pts',(-2.48340195179236,-2.52515037406617,
-6.25833493558313));
#47348=CARTESIAN_POINT('Ctrl Pts',(-2.55930369651983,-2.44572373521217,
-6.26203942766823));
#47349=CARTESIAN_POINT('Ctrl Pts',(-2.61685592304164,-2.38549877032363,
-6.26484834554482));
#47350=CARTESIAN_POINT('Ctrl Pts',(-2.67225503938364,-2.32321660732287,
-6.26765726342143));
#47351=CARTESIAN_POINT('Ctrl Pts',(-2.72538469578074,-2.25905832714279,
-6.27046618129807));
#47352=CARTESIAN_POINT('Ctrl Pts',(-2.84858346785115,-2.11028602420789,
-6.27697959125997));
#47353=CARTESIAN_POINT('Ctrl Pts',(-2.95958197207277,-1.95142785557342,
-6.28349300122203));
#47354=CARTESIAN_POINT('Ctrl Pts',(-3.05700615397888,-1.7846428881584,-6.29000641118393));
#47355=CARTESIAN_POINT('Ctrl Pts',(-3.14712345334602,-1.63036691124576,
-6.29603131079256));
#47356=CARTESIAN_POINT('Ctrl Pts',(-3.22563382835918,-1.46928943033375,
-6.30205621040104));
#47357=CARTESIAN_POINT('Ctrl Pts',(-3.29140876004433,-1.30316091650401,
-6.30808111000952));
#47358=CARTESIAN_POINT('Ctrl Pts',(-3.29674191697551,-1.28969089970129,
-6.30856962036268));
#47359=CARTESIAN_POINT('Ctrl Pts',(-3.3019913531112,-1.2761876799283,-6.30905813071584));
#47360=CARTESIAN_POINT('Ctrl Pts',(-3.30715686163083,-1.26265234730167,
-6.309546641069));
#47361=CARTESIAN_POINT('Ctrl Pts',(-3.37602965916945,-1.08218294722828,
-6.31606005103064));
#47362=CARTESIAN_POINT('Ctrl Pts',(-3.42997151868652,-0.896033422041063,
-6.32257346099227));
#47363=CARTESIAN_POINT('Ctrl Pts',(-3.46851662407281,-0.70676471783212,
-6.32908687095391));
#47364=CARTESIAN_POINT('Ctrl Pts',(-3.50706172945967,-0.517496013620443,
-6.33560028091564));
#47365=CARTESIAN_POINT('Ctrl Pts',(-3.53021639596121,-0.325084951817086,
-6.34211369087737));
#47366=CARTESIAN_POINT('Ctrl Pts',(-3.53749871140976,-0.132059280579995,
-6.34862710083908));
#47367=CARTESIAN_POINT('Ctrl Pts',(-3.53954688521147,-0.077770211989136,
-6.35045901758832));
#47368=CARTESIAN_POINT('Ctrl Pts',(-3.5403393000852,-0.0234336768277718,
-6.35229093433755));
#47369=CARTESIAN_POINT('Ctrl Pts',(-3.53986520764733,0.0308919356641406,
-6.35412285108679));
#47370=CARTESIAN_POINT('Ctrl Pts',(-3.53865365666893,0.16972192684437,-6.35880434429916));
#47371=CARTESIAN_POINT('Ctrl Pts',(-3.52917019745509,0.308480469767329,
-6.36348583751154));
#47372=CARTESIAN_POINT('Ctrl Pts',(-3.51161394105595,0.446196758891979,
-6.36816733072392));
#47373=CARTESIAN_POINT('Ctrl Pts',(-3.48718773981356,0.637802857369739,
-6.37468074068564));
#47374=CARTESIAN_POINT('Ctrl Pts',(-3.4471367782153,0.827411723408661,-6.38119415064737));
#47375=CARTESIAN_POINT('Ctrl Pts',(-3.39197035063338,1.01252418815714,-6.38770756060909));
#47376=CARTESIAN_POINT('Ctrl Pts',(-3.35680189836082,1.13053289683955,-6.39185984230308));
#47377=CARTESIAN_POINT('Ctrl Pts',(-3.31548686207736,1.2467199728331,-6.39601212399706));
#47378=CARTESIAN_POINT('Ctrl Pts',(-3.26816416858,1.3604054422155,-6.40016440569104));
#47379=CARTESIAN_POINT('Ctrl Pts',(-3.2412548792897,1.42505085771546,-6.40252553395869));
#47380=CARTESIAN_POINT('Ctrl Pts',(-3.21240318873926,1.48888742428309,-6.40488666222635));
#47381=CARTESIAN_POINT('Ctrl Pts',(-3.1816796260222,1.55180881165512,-6.407247790494));
#47382=CARTESIAN_POINT('Ctrl Pts',(-3.0969255861,1.72538379143208,-6.41376120045564));
#47383=CARTESIAN_POINT('Ctrl Pts',(-2.9979321353066,1.89198966135704,-6.42027461041727));
#47384=CARTESIAN_POINT('Ctrl Pts',(-2.88612844378586,2.04949663734564,-6.42678802037891));
#47385=CARTESIAN_POINT('Ctrl Pts',(-2.7743247522635,2.20700361333651,-6.43330143034064));
#47386=CARTESIAN_POINT('Ctrl Pts',(-2.64969465291328,2.3554295711336,-6.43981484030237));
#47387=CARTESIAN_POINT('Ctrl Pts',(-2.51368120782473,2.4925903433037,-6.44632825026408));
#47388=CARTESIAN_POINT('Ctrl Pts',(-2.37766776273814,2.62975111547182,-6.4528416602257));
#47389=CARTESIAN_POINT('Ctrl Pts',(-2.23029846571805,2.75562791640694,-6.4593550701873));
#47390=CARTESIAN_POINT('Ctrl Pts',(-2.07374054798118,2.86875662093084,-6.46586848014892));
#47391=CARTESIAN_POINT('Ctrl Pts',(-1.91718263024204,2.98188532545637,-6.47238189011064));
#47392=CARTESIAN_POINT('Ctrl Pts',(-1.7514182091273,3.08228207284204,-6.47889530007237));
#47393=CARTESIAN_POINT('Ctrl Pts',(-1.57856280904735,3.16849459675079,-6.4854087100341));
#47394=CARTESIAN_POINT('Ctrl Pts',(-1.51806293971028,3.19866921917673,-6.48768842158167));
#47395=CARTESIAN_POINT('Ctrl Pts',(-1.45669512500733,3.22710553504123,-6.48996813312925));
#47396=CARTESIAN_POINT('Ctrl Pts',(-1.39455435995192,3.25373910096334,-6.49224784467683));
#47397=CARTESIAN_POINT('Ctrl Pts',(-1.27915148859172,3.30320083480635,-6.49648154309089));
#47398=CARTESIAN_POINT('Ctrl Pts',(-1.16108267271159,3.34644458612958,-6.50071524150494));
#47399=CARTESIAN_POINT('Ctrl Pts',(-1.04106677331438,3.38331569520124,-6.504948939919));
#47400=CARTESIAN_POINT('Ctrl Pts',(-0.856426140412246,3.44004072037697,
-6.51146234988064));
#47401=CARTESIAN_POINT('Ctrl Pts',(-0.667162346706343,3.48169169421644,
-6.51797575984227));
#47402=CARTESIAN_POINT('Ctrl Pts',(-0.475768876624549,3.5077327830413,-6.52448916980391));
#47403=CARTESIAN_POINT('Ctrl Pts',(-0.340597831264554,3.5261242213556,-6.52908924541253));
#47404=CARTESIAN_POINT('Ctrl Pts',(-0.204354645869283,3.53672868968354,
-6.53368932102115));
#47405=CARTESIAN_POINT('Ctrl Pts',(-0.0679589460948733,3.53934762091083,
-6.53828939662977));
#47406=CARTESIAN_POINT('Ctrl Pts',(-0.0112271442293264,3.54043692715533,
-6.54020273098288));
#47407=CARTESIAN_POINT('Ctrl Pts',(0.045531022636131,3.54014484257323,-6.54211606533599));
#47408=CARTESIAN_POINT('Ctrl Pts',(0.102248860493038,3.53848292849331,-6.5440293996891));
#47409=CARTESIAN_POINT('Ctrl Pts',(0.295328825580803,3.53282540830823,-6.55054280965073));
#47410=CARTESIAN_POINT('Ctrl Pts',(0.487928089795479,3.51129585116066,-6.55705621961237));
#47411=CARTESIAN_POINT('Ctrl Pts',(0.677515362239871,3.47434925711893,-6.563569629574));
#47412=CARTESIAN_POINT('Ctrl Pts',(0.867102634684262,3.43740266307719,-6.57008303953564));
#47413=CARTESIAN_POINT('Ctrl Pts',(1.053701106507,3.38503272719013,-6.57659644949727));
#47414=CARTESIAN_POINT('Ctrl Pts',(1.23474298622044,3.31767899823506,-6.58310985945891));
#47415=CARTESIAN_POINT('Ctrl Pts',(1.24605820178868,3.31346935368399,-6.58351695111039));
#47416=CARTESIAN_POINT('Ctrl Pts',(1.25735159732433,3.30920121986826,-6.58392404276187));
#47417=CARTESIAN_POINT('Ctrl Pts',(1.26862254139057,3.30487470980033,-6.58433113441336));
#47418=CARTESIAN_POINT('Ctrl Pts',(1.43768513914876,3.2399776588513,-6.5904374527236));
#47419=CARTESIAN_POINT('Ctrl Pts',(1.60169567108907,3.16194539799143,-6.59654377103386));
#47420=CARTESIAN_POINT('Ctrl Pts',(1.75882144669102,3.07193280717094,-6.60265008934425));
#47421=CARTESIAN_POINT('Ctrl Pts',(1.92642237085479,2.97591932147712,-6.60916349930603));
#47422=CARTESIAN_POINT('Ctrl Pts',(2.08621238736183,2.86626604784555,-6.61567690926797));
#47423=CARTESIAN_POINT('Ctrl Pts',(2.23601720366442,2.74432457051421,-6.62219031922976));
#47424=CARTESIAN_POINT('Ctrl Pts',(2.29874823302859,2.6932613631756,-6.6249178210662));
#47425=CARTESIAN_POINT('Ctrl Pts',(2.3597278326295,2.64004307078317,-6.62764532290262));
#47426=CARTESIAN_POINT('Ctrl Pts',(2.41878915883033,2.5847744592375,-6.63037282473902));
#47427=CARTESIAN_POINT('Ctrl Pts',(2.50076921536961,2.50805887916477,-6.6341587328644));
#47428=CARTESIAN_POINT('Ctrl Pts',(2.57905316667217,2.42739285957258,-6.63794464098975));
#47429=CARTESIAN_POINT('Ctrl Pts',(2.65333228007531,2.34320336556039,-6.64173054911509));
#47430=CARTESIAN_POINT('Ctrl Pts',(2.78112468843889,2.19836078861232,-6.64824395907673));
#47431=CARTESIAN_POINT('Ctrl Pts',(2.89707465218622,2.04308253276765,-6.65475736903837));
#47432=CARTESIAN_POINT('Ctrl Pts',(2.9996904458398,1.87943880835007,-6.661270779));
#47433=CARTESIAN_POINT('Ctrl Pts',(3.07921739666291,1.75261538321336,-6.66631865335995));
#47434=CARTESIAN_POINT('Ctrl Pts',(3.15074015167961,1.62075497546953,-6.6713665277199));
#47435=CARTESIAN_POINT('Ctrl Pts',(3.21353227400634,1.48486037185928,-6.67641440207985));
#47436=CARTESIAN_POINT('Ctrl Pts',(3.23176253970101,1.44540646206153,-6.67787993768153));
#47437=CARTESIAN_POINT('Ctrl Pts',(3.2492569706675,1.40561255518628,-6.67934547328322));
#47438=CARTESIAN_POINT('Ctrl Pts',(3.26600829512753,1.36550806014452,-6.68081100888491));
#47439=CARTESIAN_POINT('Ctrl Pts',(3.34045769334387,1.18726809298532,-6.68732441884663));
#47440=CARTESIAN_POINT('Ctrl Pts',(3.4002225314738,1.00291223761149,-6.69383782880837));
#47441=CARTESIAN_POINT('Ctrl Pts',(3.44470072231061,0.814949462094048,-6.70035123877009));
#47442=CARTESIAN_POINT('Ctrl Pts',(3.48917891314677,0.626986686579336,-6.70686464873173));
#47443=CARTESIAN_POINT('Ctrl Pts',(3.51837528864164,0.435393488100818,-6.71337805869337));
#47444=CARTESIAN_POINT('Ctrl Pts',(3.53166214900558,0.242686469356258,-6.719891468655));
#47445=CARTESIAN_POINT('Ctrl Pts',(3.53340607022177,0.217393371567027,-6.7207463639057));
#47446=CARTESIAN_POINT('Ctrl Pts',(3.53487587375559,0.192081558293536,-6.7216012591564));
#47447=CARTESIAN_POINT('Ctrl Pts',(3.53607015736517,0.16675683551214,-6.7224561544071));
#47448=CARTESIAN_POINT('Ctrl Pts',(3.54397506895323,-0.000866409899313997,
-6.72811466911803));
#47449=CARTESIAN_POINT('Ctrl Pts',(3.53980817195322,-0.169055081500192,
-6.73377318382897));
#47450=CARTESIAN_POINT('Ctrl Pts',(3.52382484364409,-0.336095312099889,
-6.73943169853991));
#47451=CARTESIAN_POINT('Ctrl Pts',(3.50542673475007,-0.52837218290042,-6.74594510850164));
#47452=CARTESIAN_POINT('Ctrl Pts',(3.47137388730705,-0.719151067248053,
-6.75245851846337));
#47453=CARTESIAN_POINT('Ctrl Pts',(3.42203117938897,-0.905902528285193,
-6.75897192842508));
#47454=CARTESIAN_POINT('Ctrl Pts',(3.39797659515054,-0.99694391901358,-6.76214721764641));
#47455=CARTESIAN_POINT('Ctrl Pts',(3.37028711544748,-1.08702913815711,-6.76532250686773));
#47456=CARTESIAN_POINT('Ctrl Pts',(3.33900820913433,-1.17585040686805,-6.76849779608906));
#47457=CARTESIAN_POINT('Ctrl Pts',(3.30612529402972,-1.2692265054204,-6.77183591682935));
#47458=CARTESIAN_POINT('Ctrl Pts',(3.2692753640432,-1.3612056436035,-6.77517403756963));
#47459=CARTESIAN_POINT('Ctrl Pts',(3.2286413672435,-1.45147605409633,-6.77851215830992));
#47460=CARTESIAN_POINT('Ctrl Pts',(3.14935547553055,-1.62761353883595,-6.78502556827164));
#47461=CARTESIAN_POINT('Ctrl Pts',(3.05566316088876,-1.79725369188204,-6.79153897823337));
#47462=CARTESIAN_POINT('Ctrl Pts',(2.94886369882296,-1.95819733025196,-6.79805238819509));
#47463=CARTESIAN_POINT('Ctrl Pts',(2.85875186152997,-2.09399321043342,-6.80354806511463));
#47464=CARTESIAN_POINT('Ctrl Pts',(2.75929726145042,-2.22360994758072,-6.80904374203417));
#47465=CARTESIAN_POINT('Ctrl Pts',(2.65130325159267,-2.34567497068367,-6.81453941895371));
#47466=CARTESIAN_POINT('Ctrl Pts',(2.63130406426958,-2.36827993984675,-6.8155571519958));
#47467=CARTESIAN_POINT('Ctrl Pts',(2.61101205412421,-2.39062594672813,-6.8165748850379));
#47468=CARTESIAN_POINT('Ctrl Pts',(2.5904352191543,-2.41270682914795,-6.81759261808));
#47469=CARTESIAN_POINT('Ctrl Pts',(2.45874512329616,-2.55402270822995,-6.82410602804164));
#47470=CARTESIAN_POINT('Ctrl Pts',(2.3154071367893,-2.68446116186662,-6.83061943800327));
#47471=CARTESIAN_POINT('Ctrl Pts',(2.1624843817763,-2.80245664730059,-6.83713284796491));
#47472=CARTESIAN_POINT('Ctrl Pts',(2.00956162676109,-2.92045213273626,-6.84364625792664));
#47473=CARTESIAN_POINT('Ctrl Pts',(1.84703531539659,-3.02601956514964,-6.85015966788837));
#47474=CARTESIAN_POINT('Ctrl Pts',(1.67694939807015,-3.11757873618206,-6.8566730778501));
#47475=CARTESIAN_POINT('Ctrl Pts',(1.64293177974845,-3.13589080447667,-6.85797577649519));
#47476=CARTESIAN_POINT('Ctrl Pts',(1.60861252646917,-3.15364206036475,-6.85927847514029));
#47477=CARTESIAN_POINT('Ctrl Pts',(1.57400853431423,-3.17081963124785,-6.86058117378538));
#47478=CARTESIAN_POINT('Ctrl Pts',(1.43559477745792,-3.2395288168513,-6.86579188510192));
#47479=CARTESIAN_POINT('Ctrl Pts',(1.29262501833188,-3.29905833593406,-6.87100259641846));
#47480=CARTESIAN_POINT('Ctrl Pts',(1.14641104468838,-3.34905016806174,-6.876213307735));
#47481=CARTESIAN_POINT('Ctrl Pts',(0.963642993532519,-3.41154015793072,
-6.88272671769664));
#47482=CARTESIAN_POINT('Ctrl Pts',(0.775786184883246,-3.45913891306697,
-6.88924012765827));
#47483=CARTESIAN_POINT('Ctrl Pts',(0.585300931640267,-3.49116675003133,
-6.89575353761991));
#47484=CARTESIAN_POINT('Ctrl Pts',(0.479343748210392,-3.50898219421044,
-6.89937661374947));
#47485=CARTESIAN_POINT('Ctrl Pts',(0.372569808297704,-3.52197909098866,
-6.90299968987904));
#47486=CARTESIAN_POINT('Ctrl Pts',(0.265424692965157,-3.53003537267917,
-6.9066227660086));
#47487=CARTESIAN_POINT('Ctrl Pts',(0.1799489423262,-3.53646232665386,-6.90951309984076));
#47488=CARTESIAN_POINT('Ctrl Pts',(0.0942370119385343,-3.53974508577457,
-6.91240343367292));
#47489=CARTESIAN_POINT('Ctrl Pts',(0.00852186074184726,-3.53991094251116,
-6.91529376750508));
#47490=CARTESIAN_POINT('Ctrl Pts',(-0.184638497918042,-3.54028470311567,
-6.9218071774667));
#47491=CARTESIAN_POINT('Ctrl Pts',(-0.377816489562962,-3.52483316308227,
-6.9283205874283));
#47492=CARTESIAN_POINT('Ctrl Pts',(-0.568472409011395,-3.49386453342436,
-6.93483399739009));
#47493=CARTESIAN_POINT('Ctrl Pts',(-0.742445766719096,-3.46560568627825,
-6.94077747821385));
#47494=CARTESIAN_POINT('Ctrl Pts',(-0.914338116430782,-3.42442020539666,
-6.94672095903777));
#47495=CARTESIAN_POINT('Ctrl Pts',(-1.08216137956925,-3.37053805030733,
-6.95266443986157));
#47496=CARTESIAN_POINT('Ctrl Pts',(-1.09825419967799,-3.36537121102231,
-6.95323436899969));
#47497=CARTESIAN_POINT('Ctrl Pts',(-1.11430960469959,-3.3600876333587,-6.95380429813781));
#47498=CARTESIAN_POINT('Ctrl Pts',(-1.13032604705382,-3.35468816325393,
-6.95437422727593));
#47499=CARTESIAN_POINT('Ctrl Pts',(-1.31336925050718,-3.29298055784017,
-6.96088763723773));
#47500=CARTESIAN_POINT('Ctrl Pts',(-1.49129514513555,-3.21614619228149,
-6.96740104719937));
#47501=CARTESIAN_POINT('Ctrl Pts',(-1.66183108821857,-3.12544975106934,
-6.973914457161));
#47502=CARTESIAN_POINT('Ctrl Pts',(-1.83236703130161,-3.0347533098572,-6.98042786712264));
#47503=CARTESIAN_POINT('Ctrl Pts',(-1.99553483595644,-2.93018474734963,
-6.98694127708427));
#47504=CARTESIAN_POINT('Ctrl Pts',(-2.14907398699859,-2.81297668049842,
-6.99345468704591));
#47505=CARTESIAN_POINT('Ctrl Pts',(-2.19033810662407,-2.78147665162115,
-6.99520518602941));
#47506=CARTESIAN_POINT('Ctrl Pts',(-2.23090577145553,-2.74906427885111,
-6.99695568501291));
#47507=CARTESIAN_POINT('Ctrl Pts',(-2.27073169575485,-2.71576463742649,
-6.99870618399641));
#47508=CARTESIAN_POINT('Ctrl Pts',(-2.37909355934424,-2.62516005598574,
-7.00346909497464));
#47509=CARTESIAN_POINT('Ctrl Pts',(-2.48196353080434,-2.52798626286371,
-7.00823200595286));
#47510=CARTESIAN_POINT('Ctrl Pts',(-2.57868524344307,-2.42505371417111,
-7.01299491693108));
#47511=CARTESIAN_POINT('Ctrl Pts',(-2.71095480915343,-2.28429066168171,
-7.0195083268927));
#47512=CARTESIAN_POINT('Ctrl Pts',(-2.83174365337413,-2.13274635689841,
-7.0260217368543));
#47513=CARTESIAN_POINT('Ctrl Pts',(-2.93944340626971,-1.97240050926644,
-7.03253514681592));
#47514=CARTESIAN_POINT('Ctrl Pts',(-3.00675548551217,-1.8721847509957,-7.03660601193573));
#47515=CARTESIAN_POINT('Ctrl Pts',(-3.0689565651283,-1.76852498435215,-7.04067687705556));
#47516=CARTESIAN_POINT('Ctrl Pts',(-3.12563447872083,-1.66192933226244,
-7.04474774217538));
#47517=CARTESIAN_POINT('Ctrl Pts',(-3.15964158566754,-1.59797126622053,
-7.04719028701728));
#47518=CARTESIAN_POINT('Ctrl Pts',(-3.19166042350247,-1.53295634899612,
-7.04963283185919));
#47519=CARTESIAN_POINT('Ctrl Pts',(-3.22164958182273,-1.467019693314,-7.0520753767011));
#47520=CARTESIAN_POINT('Ctrl Pts',(-3.30162014334238,-1.29118977093615,
-7.05858878666273));
#47521=CARTESIAN_POINT('Ctrl Pts',(-3.36715796958855,-1.10881135569454,
-7.06510219662437));
#47522=CARTESIAN_POINT('Ctrl Pts',(-3.41752451187652,-0.92233949801837,
-7.071615606586));
#47523=CARTESIAN_POINT('Ctrl Pts',(-3.46694667627976,-0.739364006987898,
-7.07800688943621));
#47524=CARTESIAN_POINT('Ctrl Pts',(-3.50176440608703,-0.552424156172237,
-7.08439817228643));
#47525=CARTESIAN_POINT('Ctrl Pts',(-3.52124797259483,-0.363885580226897,
-7.09078945513664));
#47526=CARTESIAN_POINT('Ctrl Pts',(-3.52162027213994,-0.360282911997128,
-7.09091158224806));
#47527=CARTESIAN_POINT('Ctrl Pts',(-3.52198697295808,-0.35667966015706,
-7.09103370935948));
#47528=CARTESIAN_POINT('Ctrl Pts',(-3.52234807653483,-0.353075841902743,
-7.09115583647091));
#47529=CARTESIAN_POINT('Ctrl Pts',(-3.54160682757397,-0.160873263421083,
-7.09766924643264));
#47530=CARTESIAN_POINT('Ctrl Pts',(-3.54494113425226,0.0329083541594109,
-7.10418265639437));
#47531=CARTESIAN_POINT('Ctrl Pts',(-3.53259533909181,0.22566737745008,-7.11069606635609));
#47532=CARTESIAN_POINT('Ctrl Pts',(-3.52024954393154,0.418426400737956,
-7.11720947631773));
#47533=CARTESIAN_POINT('Ctrl Pts',(-3.49222452843905,0.610186888018826,
-7.12372288627936));
#47534=CARTESIAN_POINT('Ctrl Pts',(-3.44874073224416,0.798391072008908,
-7.130236296241));
#47535=CARTESIAN_POINT('Ctrl Pts',(-3.43406482543378,0.861910527697223,
-7.13243459091578));
#47536=CARTESIAN_POINT('Ctrl Pts',(-3.4176279918563,0.925023822733724,-7.13463288559057));
#47537=CARTESIAN_POINT('Ctrl Pts',(-3.399439647296,0.987628515379085,-7.13683118026536));
#47538=CARTESIAN_POINT('Ctrl Pts',(-3.36373706176239,1.11051762090298,-7.14114629555221));
#47539=CARTESIAN_POINT('Ctrl Pts',(-3.32128518726173,1.23144678337572,-7.14546141083906));
#47540=CARTESIAN_POINT('Ctrl Pts',(-3.27244048985516,1.34972428826295,-7.14977652612591));
#47541=CARTESIAN_POINT('Ctrl Pts',(-3.19871232327865,1.52825714946575,-7.15628993608764));
#47542=CARTESIAN_POINT('Ctrl Pts',(-3.11041628697104,1.7007662450445,-7.16280334604937));
#47543=CARTESIAN_POINT('Ctrl Pts',(-3.00872059248994,1.86498453844867,-7.16931675601108));
#47544=CARTESIAN_POINT('Ctrl Pts',(-2.9381695165832,1.97891047545466,-7.17383541418009));
#47545=CARTESIAN_POINT('Ctrl Pts',(-2.86116271344563,2.08885271017646,-7.1783540723491));
#47546=CARTESIAN_POINT('Ctrl Pts',(-2.77810835168668,2.19401777255465,-7.18287273051811));
#47547=CARTESIAN_POINT('Ctrl Pts',(-2.74144418484653,2.24044265995526,-7.18486748231071));
#47548=CARTESIAN_POINT('Ctrl Pts',(-2.70360160799484,2.2859366567572,-7.18686223410332));
#47549=CARTESIAN_POINT('Ctrl Pts',(-2.66463875530979,2.33044965099088,-7.18885698589592));
#47550=CARTESIAN_POINT('Ctrl Pts',(-2.53741438897186,2.47579674687627,-7.19537039585764));
#47551=CARTESIAN_POINT('Ctrl Pts',(-2.39825532545772,2.61067669790369,-7.20188380581937));
#47552=CARTESIAN_POINT('Ctrl Pts',(-2.24911868144474,2.73342304268973,-7.20839721578109));
#47553=CARTESIAN_POINT('Ctrl Pts',(-2.09998203743392,2.85616938747399,-7.21491062574273));
#47554=CARTESIAN_POINT('Ctrl Pts',(-1.94084807500285,2.96679585561946,-7.22142403570437));
#47555=CARTESIAN_POINT('Ctrl Pts',(-1.7736881360114,3.06359595272342,-7.227937445666));
#47556=CARTESIAN_POINT('Ctrl Pts',(-1.76533007352107,3.0684359955324,-7.22826311871789));
#47557=CARTESIAN_POINT('Ctrl Pts',(-1.75695201419097,3.07324143239533,-7.22858879176977));
#47558=CARTESIAN_POINT('Ctrl Pts',(-1.74855420770786,3.07801205044834,-7.22891446482166));
#47559=CARTESIAN_POINT('Ctrl Pts',(-1.58899720157694,3.16865304526785,-7.23510220173141));
#47560=CARTESIAN_POINT('Ctrl Pts',(-1.42231138155771,3.24672375067996,-7.24128993864116));
#47561=CARTESIAN_POINT('Ctrl Pts',(-1.25063380441199,3.31151429393604,-7.24747767555091));
#47562=CARTESIAN_POINT('Ctrl Pts',(-1.0699204907246,3.37971489393329,-7.25399108551264));
#47563=CARTESIAN_POINT('Ctrl Pts',(-0.883654985072044,3.43321218577804,
-7.26050449547437));
#47564=CARTESIAN_POINT('Ctrl Pts',(-0.69426261018899,3.47118330719089,-7.2670179054361));
#47565=CARTESIAN_POINT('Ctrl Pts',(-0.61732158273511,3.48660915047991,-7.26966399113513));
#47566=CARTESIAN_POINT('Ctrl Pts',(-0.539864762333473,3.49947197571339,
-7.27231007683416));
#47567=CARTESIAN_POINT('Ctrl Pts',(-0.462062720458959,3.5097148092635,-7.2749561625332));
#47568=CARTESIAN_POINT('Ctrl Pts',(-0.34835297767497,3.52468498151477,-7.27882348679582));
#47569=CARTESIAN_POINT('Ctrl Pts',(-0.233905849409282,3.53405841436472,
-7.28269081105846));
#47570=CARTESIAN_POINT('Ctrl Pts',(-0.119281726467647,3.53786972306194,
-7.28655813532117));
#47571=CARTESIAN_POINT('Ctrl Pts',(0.0737700720151849,3.54428879070397,
-7.29307154528297));
#47572=CARTESIAN_POINT('Ctrl Pts',(0.267337123262925,3.53493519022353,-7.29958495524494));
#47573=CARTESIAN_POINT('Ctrl Pts',(0.45887316707087,3.50996979757638,-7.30609836520674));
#47574=CARTESIAN_POINT('Ctrl Pts',(0.604918840965994,3.49093375861096,-7.31106482127587));
#47575=CARTESIAN_POINT('Ctrl Pts',(0.749795644587637,3.46281672251746,-7.3160312773449));
#47576=CARTESIAN_POINT('Ctrl Pts',(0.892325528180709,3.42569046350633,-7.3209977334139));
#47577=CARTESIAN_POINT('Ctrl Pts',(0.936720798206521,3.4141263602299,-7.32254468730663));
#47578=CARTESIAN_POINT('Ctrl Pts',(0.98088838046976,3.40168827258433,-7.32409164119935));
#47579=CARTESIAN_POINT('Ctrl Pts',(1.02479609483758,3.38839156064891,-7.32563859509208));
#47580=CARTESIAN_POINT('Ctrl Pts',(1.2096684077747,3.33240609373605,-7.3321520050537));
#47581=CARTESIAN_POINT('Ctrl Pts',(1.38991621050558,3.26120588847558,-7.3386654150153));
#47582=CARTESIAN_POINT('Ctrl Pts',(1.56321999725237,3.17591743890142,-7.34517882497692));
#47583=CARTESIAN_POINT('Ctrl Pts',(1.73652378400167,3.09062898932603,-7.35169223493864));
#47584=CARTESIAN_POINT('Ctrl Pts',(1.90290467519647,2.99124089947101,-7.35820564490037));
#47585=CARTESIAN_POINT('Ctrl Pts',(2.06001785169516,2.87886643810324,-7.3647190548621));
#47586=CARTESIAN_POINT('Ctrl Pts',(2.07867525608196,2.86552181726869,-7.3654925311949));
#47587=CARTESIAN_POINT('Ctrl Pts',(2.09720163827227,2.85199428966467,-7.3662660075277));
#47588=CARTESIAN_POINT('Ctrl Pts',(2.11559302029352,2.83828578062299,-7.3670394838605));
#47589=CARTESIAN_POINT('Ctrl Pts',(2.25207465220354,2.73655554181339,-7.37277941748934));
#47590=CARTESIAN_POINT('Ctrl Pts',(2.38112092105923,2.62485779238668,-7.37851935111817));
#47591=CARTESIAN_POINT('Ctrl Pts',(2.50151996034344,2.50453286898932,-7.384259284747));
#47592=CARTESIAN_POINT('Ctrl Pts',(2.63814319548082,2.36799373711636,-7.39077269470864));
#47593=CARTESIAN_POINT('Ctrl Pts',(2.76365118020096,2.22033192223027,-7.39728610467027));
#47594=CARTESIAN_POINT('Ctrl Pts',(2.87632012344211,2.06343515614491,-7.40379951463191));
#47595=CARTESIAN_POINT('Ctrl Pts',(2.92983793594804,1.98890910248192,-7.40689338809049));
#47596=CARTESIAN_POINT('Ctrl Pts',(2.98045881580538,1.91229818395693,-7.40998726154908));
#47597=CARTESIAN_POINT('Ctrl Pts',(3.02798948096801,1.83381561318099,-7.41308113500767));
#47598=CARTESIAN_POINT('Ctrl Pts',(3.08052325350839,1.74707191819124,-7.41650067151081));
#47599=CARTESIAN_POINT('Ctrl Pts',(3.12928194035441,1.65804182176638,-7.41992020801395));
#47600=CARTESIAN_POINT('Ctrl Pts',(3.17413145383252,1.5670900227261,-7.4233397445171));
#47601=CARTESIAN_POINT('Ctrl Pts',(3.25955919165442,1.39384831194062,-7.42985315447873));
#47602=CARTESIAN_POINT('Ctrl Pts',(3.33081116461456,1.21362870349055,-7.43636656444037));
#47603=CARTESIAN_POINT('Ctrl Pts',(3.38701269619474,1.02883041976208,-7.442879974402));
#47604=CARTESIAN_POINT('Ctrl Pts',(3.43373009893555,0.87521724225577,-7.44829423248071));
#47605=CARTESIAN_POINT('Ctrl Pts',(3.47004976409285,0.718424299931465,-7.45370849055942));
#47606=CARTESIAN_POINT('Ctrl Pts',(3.49544487589833,0.559879558080886,-7.45912274863812));
#47607=CARTESIAN_POINT('Ctrl Pts',(3.50060035326059,0.527693291929511,-7.46022190052105));
#47608=CARTESIAN_POINT('Ctrl Pts',(3.50530563687768,0.495434842487014,-7.46132105240398));
#47609=CARTESIAN_POINT('Ctrl Pts',(3.50956112158859,0.463116931447565,-7.46242020428691));
#47610=CARTESIAN_POINT('Ctrl Pts',(3.53477848866818,0.271605815489876,-7.46893361424864));
#47611=CARTESIAN_POINT('Ctrl Pts',(3.54419862852173,0.0780313815552228,
-7.47544702421037));
#47612=CARTESIAN_POINT('Ctrl Pts',(3.53792067981413,-0.115020209061044,
-7.48196043417208));
#47613=CARTESIAN_POINT('Ctrl Pts',(3.53164273110663,-0.308071799674505,
-7.4884738441337));
#47614=CARTESIAN_POINT('Ctrl Pts',(3.50966604727128,-0.500624506508935,
-7.4949872540953));
#47615=CARTESIAN_POINT('Ctrl Pts',(3.47206668295341,-0.690093950472241,
-7.50150066405692));
#47616=CARTESIAN_POINT('Ctrl Pts',(3.46501671280743,-0.725619921396251,
-7.50272194390064));
#47617=CARTESIAN_POINT('Ctrl Pts',(3.45741761512174,-0.761036669986838,
-7.50394322374436));
#47618=CARTESIAN_POINT('Ctrl Pts',(3.44927002934,-0.796326732377223,-7.50516450358807));
#47619=CARTESIAN_POINT('Ctrl Pts',(3.41396437492646,-0.949247951050361,
-7.51045663370608));
#47620=CARTESIAN_POINT('Ctrl Pts',(3.36835867813816,-1.09978996669337,-7.51574876382412));
#47621=CARTESIAN_POINT('Ctrl Pts',(3.31303614425419,-1.24665390493681,-7.52104089394225));
#47622=CARTESIAN_POINT('Ctrl Pts',(3.24494668166318,-1.42741002594109,-7.52755430304353));
#47623=CARTESIAN_POINT('Ctrl Pts',(3.16213450723209,-1.60261747901651,-7.53406771214497));
#47624=CARTESIAN_POINT('Ctrl Pts',(3.06563512605655,-1.76994523770567,-7.54058112124546));
#47625=CARTESIAN_POINT('',(-1.368080573303,-3.758770483144,-4.441666666667));
#47626=CARTESIAN_POINT('Ctrl Pts',(-3.361449115544,-1.040542320116,-2.023855154456));
#47627=CARTESIAN_POINT('Ctrl Pts',(-3.495234334804,-0.6083521071266,-2.039202376679));
#47628=CARTESIAN_POINT('Ctrl Pts',(-3.593966410624,0.3080871692045,-2.069896821123));
#47629=CARTESIAN_POINT('Ctrl Pts',(-3.214002747139,1.6376218606,-2.11593848779));
#47630=CARTESIAN_POINT('Ctrl Pts',(-2.361752530656,2.726480536661,-2.161980154456));
#47631=CARTESIAN_POINT('Ctrl Pts',(-1.162463196152,3.414713247338,-2.208021821123));
#47632=CARTESIAN_POINT('Ctrl Pts',(0.2076425386167,3.6011758161,-2.25406348779));
#47633=CARTESIAN_POINT('Ctrl Pts',(1.5472364757,3.258472506991,-2.300105154456));
#47634=CARTESIAN_POINT('Ctrl Pts',(2.659475311144,2.436960122203,-2.346146821123));
#47635=CARTESIAN_POINT('Ctrl Pts',(3.380923545207,1.257354198423,-2.39218848779));
#47636=CARTESIAN_POINT('Ctrl Pts',(3.605569620214,-0.1070108088044,-2.438230154456));
#47637=CARTESIAN_POINT('Ctrl Pts',(3.300403421044,-1.455651350858,-2.484271821123));
#47638=CARTESIAN_POINT('Ctrl Pts',(2.510266906159,-2.590394498517,-2.53031348779));
#47639=CARTESIAN_POINT('Ctrl Pts',(1.351264898242,-3.344497985119,-2.576355154456));
#47640=CARTESIAN_POINT('Ctrl Pts',(-0.006295673909096,-3.607151779769,-2.622396821123));
#47641=CARTESIAN_POINT('Ctrl Pts',(-1.362931142503,-3.339760814575,-2.66843848779));
#47642=CARTESIAN_POINT('Ctrl Pts',(-2.519293776961,-2.581616250171,-2.714480154456));
#47643=CARTESIAN_POINT('Ctrl Pts',(-3.305464485361,-1.444121924838,-2.760521821123));
#47644=CARTESIAN_POINT('Ctrl Pts',(-3.605921191072,-0.09442436949411,-2.80656348779));
#47645=CARTESIAN_POINT('Ctrl Pts',(-3.376513963031,1.269148161262,-2.852605154456));
#47646=CARTESIAN_POINT('Ctrl Pts',(-2.650952527502,2.446228585948,-2.898646821123));
#47647=CARTESIAN_POINT('Ctrl Pts',(-1.535852868594,3.263853483815,-2.94468848779));
#47648=CARTESIAN_POINT('Ctrl Pts',(-0.1950707836154,3.601878813503,-2.990730154456));
#47649=CARTESIAN_POINT('Ctrl Pts',(1.174375536461,3.410634207467,-3.036771821123));
#47650=CARTESIAN_POINT('Ctrl Pts',(2.371255899469,2.718221671795,-3.08281348779));
#47651=CARTESIAN_POINT('Ctrl Pts',(3.219697427502,1.626386200482,-3.128855154456));
#47652=CARTESIAN_POINT('Ctrl Pts',(3.595027799181,0.2955650874075,-3.174896821123));
#47653=CARTESIAN_POINT('Ctrl Pts',(3.442094941941,-1.078687168943,-3.22093848779));
#47654=CARTESIAN_POINT('Ctrl Pts',(2.783371228594,-2.294434178968,-3.266980154456));
#47655=CARTESIAN_POINT('Ctrl Pts',(1.715651325333,-3.173030747985,-3.313021821123));
#47656=CARTESIAN_POINT('Ctrl Pts',(0.3958289184352,-3.585373490323,-3.35906348779));
#47657=CARTESIAN_POINT('Ctrl Pts',(-0.9821576736188,-3.470871634321,-3.405105154456));
#47658=CARTESIAN_POINT('Ctrl Pts',(-2.215823327712,-2.846350396235,-3.451146821123));
#47659=CARTESIAN_POINT('Ctrl Pts',(-3.123889834539,-1.80357863689,-3.49718848779));
#47660=CARTESIAN_POINT('Ctrl Pts',(-3.572923415067,-0.4957840939792,-3.543230154456));
#47661=CARTESIAN_POINT('Ctrl Pts',(-3.496941845406,0.8848623212845,-3.589271821123));
#47662=CARTESIAN_POINT('Ctrl Pts',(-2.907110065457,2.135484644079,-3.63531348779));
#47663=CARTESIAN_POINT('Ctrl Pts',(-1.890099572078,3.072313005768,-3.681355154456));
#47664=CARTESIAN_POINT('Ctrl Pts',(-0.5953526720002,3.557687281609,-3.727396821123));
#47665=CARTESIAN_POINT('Ctrl Pts',(0.7868769799293,3.520285246431,-3.77343848779));
#47666=CARTESIAN_POINT('Ctrl Pts',(2.053480773757,2.965602857698,-3.819480154456));
#47667=CARTESIAN_POINT('Ctrl Pts',(3.018340479732,1.975146664475,-3.865521821123));
#47668=CARTESIAN_POINT('Ctrl Pts',(3.539676970626,0.6944570119162,-3.91156348779));
#47669=CARTESIAN_POINT('Ctrl Pts',(3.540883634913,-0.688278055575,-3.957605154456));
#47670=CARTESIAN_POINT('Ctrl Pts',(3.021783162039,-1.969875660898,-4.003646821123));
#47671=CARTESIAN_POINT('Ctrl Pts',(2.058653596917,-2.962014342585,-4.04968848779));
#47672=CARTESIAN_POINT('Ctrl Pts',(0.7930198351441,-3.518906526017,-4.095730154456));
#47673=CARTESIAN_POINT('Ctrl Pts',(-0.5891424326969,-3.558720948849,-4.141771821123));
#47674=CARTESIAN_POINT('Ctrl Pts',(-1.884734498254,-3.075607170766,-4.18781348779));
#47675=CARTESIAN_POINT('Ctrl Pts',(-2.903378515752,-2.140555253211,-4.233855154456));
#47676=CARTESIAN_POINT('Ctrl Pts',(-3.495392143951,-0.890964285359,-4.279896821123));
#47677=CARTESIAN_POINT('Ctrl Pts',(-3.573783279237,0.4895474142708,-4.32593848779));
#47678=CARTESIAN_POINT('Ctrl Pts',(-3.127032913541,1.798123676345,-4.371980154456));
#47679=CARTESIAN_POINT('Ctrl Pts',(-2.220787768898,2.842478721679,-4.418021821123));
#47680=CARTESIAN_POINT('Ctrl Pts',(-0.9882139884594,3.469152160271,-4.46406348779));
#47681=CARTESIAN_POINT('Ctrl Pts',(0.3895706616256,3.58605888079,-4.510105154456));
#47682=CARTESIAN_POINT('Ctrl Pts',(1.710110731203,3.176020290621,-4.556146821123));
#47683=CARTESIAN_POINT('Ctrl Pts',(2.779362449993,2.299288579191,-4.60218848779));
#47684=CARTESIAN_POINT('Ctrl Pts',(3.440207029409,1.084693119086,-4.648230154456));
#47685=CARTESIAN_POINT('Ctrl Pts',(3.595538206437,-0.2892901598772,-4.694271821123));
#47686=CARTESIAN_POINT('Ctrl Pts',(3.222531009545,-1.620764194701,-4.74031348779));
#47687=CARTESIAN_POINT('Ctrl Pts',(2.375996820758,-2.714079282501,-4.786355154456));
#47688=CARTESIAN_POINT('Ctrl Pts',(1.180325142345,-3.408577957331,-4.832396821123));
#47689=CARTESIAN_POINT('Ctrl Pts',(-0.1887792404969,-3.602218957155,-4.87843848779));
#47690=CARTESIAN_POINT('Ctrl Pts',(-1.530171890201,-3.26650979655,-4.924480154456));
#47691=CARTESIAN_POINT('Ctrl Pts',(-2.27446554662,-2.722785672557,-4.955174598901));
#47692=CARTESIAN_POINT('Ctrl Pts',(-2.581860640706,-2.390829167532,-4.970521821123));
#47693=CARTESIAN_POINT('Ctrl Pts',(-3.521415988649,-1.090060339149,-2.120535787988));
#47694=CARTESIAN_POINT('Ctrl Pts',(-3.66156786778,-0.6373027712535,-2.13588301021));
#47695=CARTESIAN_POINT('Ctrl Pts',(-3.764998471199,0.3227486260367,-2.166577454654));
#47696=CARTESIAN_POINT('Ctrl Pts',(-3.366952844534,1.715554097372,-2.212619121321));
#47697=CARTESIAN_POINT('Ctrl Pts',(-2.474145178704,2.856230103303,-2.258660787988));
#47698=CARTESIAN_POINT('Ctrl Pts',(-1.217783266811,3.577214889324,-2.304702454654));
#47699=CARTESIAN_POINT('Ctrl Pts',(0.2175239696557,3.772550962651,-2.350744121321));
#47700=CARTESIAN_POINT('Ctrl Pts',(1.620867392743,3.413538860853,-2.396785787988));
#47701=CARTESIAN_POINT('Ctrl Pts',(2.78603618861,2.552931799069,-2.442827454654));
#47702=CARTESIAN_POINT('Ctrl Pts',(3.541817180406,1.317190005122,-2.488869121321));
#47703=CARTESIAN_POINT('Ctrl Pts',(3.777153862034,-0.1121033102479,-2.534910787988));
#47704=CARTESIAN_POINT('Ctrl Pts',(3.457465211094,-1.524923854152,-2.580952454654));
#47705=CARTESIAN_POINT('Ctrl Pts',(2.629727154949,-2.71366791239,-2.626994121321));
#47706=CARTESIAN_POINT('Ctrl Pts',(1.415569789697,-3.50365817657,-2.673035787988));
#47707=CARTESIAN_POINT('Ctrl Pts',(-0.006595276620518,-3.778811314449,-2.719077454654));
#47708=CARTESIAN_POINT('Ctrl Pts',(-1.427791214939,-3.498695570408,-2.765119121321));
#47709=CARTESIAN_POINT('Ctrl Pts',(-2.639183602474,-2.704471918932,-2.811160787988));
#47710=CARTESIAN_POINT('Ctrl Pts',(-3.462767124701,-1.512845758149,-2.857202454654));
#47711=CARTESIAN_POINT('Ctrl Pts',(-3.77752216368,-0.09891789910402,-2.903244121321));
#47712=CARTESIAN_POINT('Ctrl Pts',(-3.537197752104,1.329545226898,-2.949285787988));
#47713=CARTESIAN_POINT('Ctrl Pts',(-2.77710781708,2.562641336623,-2.995327454654));
#47714=CARTESIAN_POINT('Ctrl Pts',(-1.608942054981,3.419175911177,-3.041369121321));
#47715=CARTESIAN_POINT('Ctrl Pts',(-0.2043539416274,3.773287414762,-3.087410787988));
#47716=CARTESIAN_POINT('Ctrl Pts',(1.230262499482,3.572941733393,-3.133452454654));
#47717=CARTESIAN_POINT('Ctrl Pts',(2.484100800144,2.84757821009,-3.179494121321));
#47718=CARTESIAN_POINT('Ctrl Pts',(3.372918527128,1.703783747197,-3.225535787988));
#47719=CARTESIAN_POINT('Ctrl Pts',(3.76611036982,0.3096306350943,-3.271577454654));
#47720=CARTESIAN_POINT('Ctrl Pts',(3.605899642196,-1.130020450377,-3.317619121321));
#47721=CARTESIAN_POINT('Ctrl Pts',(2.915828147269,-2.403623236585,-3.363660787988));
#47722=CARTESIAN_POINT('Ctrl Pts',(1.797296880098,-3.324031042672,-3.409702454654));
#47723=CARTESIAN_POINT('Ctrl Pts',(0.4146658879059,-3.7559966253,-3.455744121321));
#47724=CARTESIAN_POINT('Ctrl Pts',(-1.028897245317,-3.636045778925,-3.501785787988));
#47725=CARTESIAN_POINT('Ctrl Pts',(-2.321271399928,-2.981804409369,-3.547827454654));
#47726=CARTESIAN_POINT('Ctrl Pts',(-3.272551578798,-1.889408534956,-3.593869121321));
#47727=CARTESIAN_POINT('Ctrl Pts',(-3.742954067594,-0.5193777967315,-3.639910787988));
#47728=CARTESIAN_POINT('Ctrl Pts',(-3.66335663653,0.9269717371343,-3.685952454654));
#47729=CARTESIAN_POINT('Ctrl Pts',(-3.045455550085,2.237109505659,-3.731994121321));
#47730=CARTESIAN_POINT('Ctrl Pts',(-1.980046885873,3.218520277643,-3.778035787988));
#47731=CARTESIAN_POINT('Ctrl Pts',(-0.6236847103744,3.726992866897,-3.824077454654));
#47732=CARTESIAN_POINT('Ctrl Pts',(0.8243234042752,3.687810918827,-3.870119121321));
#47733=CARTESIAN_POINT('Ctrl Pts',(2.151203180692,3.106731936173,-3.916160787988));
#47734=CARTESIAN_POINT('Ctrl Pts',(3.161979271192,2.06914125579,-3.962202454654));
#47735=CARTESIAN_POINT('Ctrl Pts',(3.708125469273,0.7275052934411,-4.008244121321));
#47736=CARTESIAN_POINT('Ctrl Pts',(3.709389557102,-0.7210322888216,-4.054285787988));
#47737=CARTESIAN_POINT('Ctrl Pts',(3.16558578615,-2.063619412194,-4.100327454654));
#47738=CARTESIAN_POINT('Ctrl Pts',(2.156622171596,-3.102972648419,-4.146369121321));
#47739=CARTESIAN_POINT('Ctrl Pts',(0.8307585897638,-3.686366586951,-4.192410787987));
#47740=CARTESIAN_POINT('Ctrl Pts',(-0.6171789340784,-3.72807572498,-4.238452454654));
#47741=CARTESIAN_POINT('Ctrl Pts',(-1.974426495353,-3.221971207554,-4.284494121321));
#47742=CARTESIAN_POINT('Ctrl Pts',(-3.041546420915,-2.242421418306,-4.330535787987));
#47743=CARTESIAN_POINT('Ctrl Pts',(-3.661733186854,-0.9333640855279,-4.376577454654));
#47744=CARTESIAN_POINT('Ctrl Pts',(-3.743854851551,0.5128443217669,-4.422619121321));
#47745=CARTESIAN_POINT('Ctrl Pts',(-3.275844232732,1.883693980126,-4.468660787987));
#47746=CARTESIAN_POINT('Ctrl Pts',(-2.326472092238,2.977748486993,-4.514702454654));
#47747=CARTESIAN_POINT('Ctrl Pts',(-1.03524177209,3.634244477402,-4.560744121321));
#47748=CARTESIAN_POINT('Ctrl Pts',(0.4081098090146,3.756714632584,-4.606785787988));
#47749=CARTESIAN_POINT('Ctrl Pts',(1.791492616494,3.327162853648,-4.652827454654));
#47750=CARTESIAN_POINT('Ctrl Pts',(2.911628596249,2.40870865123,-4.698869121321));
#47751=CARTESIAN_POINT('Ctrl Pts',(3.603921886428,1.136312215665,-4.744910787988));
#47752=CARTESIAN_POINT('Ctrl Pts',(3.766645066676,-0.303057092145,-4.790952454654));
#47753=CARTESIAN_POINT('Ctrl Pts',(3.375886955555,-1.697894197672,-4.836994121321));
#47754=CARTESIAN_POINT('Ctrl Pts',(2.489067335545,-2.843238690024,-4.883035787988));
#47755=CARTESIAN_POINT('Ctrl Pts',(1.236495239162,-3.570787629061,-4.929077454654));
#47756=CARTESIAN_POINT('Ctrl Pts',(-0.1977629923763,-3.773643745397,-4.975119121321));
#47757=CARTESIAN_POINT('Ctrl Pts',(-1.602990726415,-3.421958634286,-5.021160787987));
#47758=CARTESIAN_POINT('Ctrl Pts',(-2.382704323698,-2.852359405552,-5.051855232432));
#47759=CARTESIAN_POINT('Ctrl Pts',(-2.704727939686,-2.504605533888,-5.067202454654));
#47760=CARTESIAN_POINT('Ctrl Pts',(-3.681382861754,-1.139578358183,-2.217216421519));
#47761=CARTESIAN_POINT('Ctrl Pts',(-3.827901400756,-0.6662534353805,-2.232563643741));
#47762=CARTESIAN_POINT('Ctrl Pts',(-3.936030531775,0.337410082869,-2.263258088185));
#47763=CARTESIAN_POINT('Ctrl Pts',(-3.519902941929,1.793486334144,-2.309299754852));
#47764=CARTESIAN_POINT('Ctrl Pts',(-2.586537826753,2.985979669946,-2.355341421519));
#47765=CARTESIAN_POINT('Ctrl Pts',(-1.27310333747,3.739716531309,-2.401383088185));
#47766=CARTESIAN_POINT('Ctrl Pts',(0.2274054006946,3.943926109203,-2.447424754852));
#47767=CARTESIAN_POINT('Ctrl Pts',(1.694498309787,3.568605214716,-2.493466421519));
#47768=CARTESIAN_POINT('Ctrl Pts',(2.912597066077,2.668903475936,-2.539508088185));
#47769=CARTESIAN_POINT('Ctrl Pts',(3.702710815604,1.377025811821,-2.585549754852));
#47770=CARTESIAN_POINT('Ctrl Pts',(3.948738103854,-0.1171958116913,-2.631591421519));
#47771=CARTESIAN_POINT('Ctrl Pts',(3.614527001144,-1.594196357445,-2.677633088185));
#47772=CARTESIAN_POINT('Ctrl Pts',(2.749187403738,-2.836941326264,-2.723674754852));
#47773=CARTESIAN_POINT('Ctrl Pts',(1.479874681153,-3.662818368022,-2.769716421519));
#47774=CARTESIAN_POINT('Ctrl Pts',(-0.006894879331943,-3.950470849129,-2.815758088185));
#47775=CARTESIAN_POINT('Ctrl Pts',(-1.492651287375,-3.657630326242,-2.861799754852));
#47776=CARTESIAN_POINT('Ctrl Pts',(-2.759073427987,-2.827327587693,-2.907841421519));
#47777=CARTESIAN_POINT('Ctrl Pts',(-3.620069764041,-1.581569591459,-2.953883088185));
#47778=CARTESIAN_POINT('Ctrl Pts',(-3.949123136288,-0.1034114287139,-2.999924754852));
#47779=CARTESIAN_POINT('Ctrl Pts',(-3.697881541177,1.389942292534,-3.045966421519));
#47780=CARTESIAN_POINT('Ctrl Pts',(-2.903263106658,2.679054087298,-3.092008088185));
#47781=CARTESIAN_POINT('Ctrl Pts',(-1.682031241369,3.574498338538,-3.138049754852));
#47782=CARTESIAN_POINT('Ctrl Pts',(-0.2136370996395,3.944696016021,-3.184091421519));
#47783=CARTESIAN_POINT('Ctrl Pts',(1.286149462504,3.73524925932,-3.230133088185));
#47784=CARTESIAN_POINT('Ctrl Pts',(2.59694570082,2.976934748386,-3.276174754852));
#47785=CARTESIAN_POINT('Ctrl Pts',(3.526139626754,1.781181293913,-3.322216421519));
#47786=CARTESIAN_POINT('Ctrl Pts',(3.93719294046,0.3236961827811,-3.368258088185));
#47787=CARTESIAN_POINT('Ctrl Pts',(3.76970434245,-1.181353731811,-3.414299754852));
#47788=CARTESIAN_POINT('Ctrl Pts',(3.048285065944,-2.512812294202,-3.460341421519));
#47789=CARTESIAN_POINT('Ctrl Pts',(1.878942434863,-3.475031337359,-3.506383088185));
#47790=CARTESIAN_POINT('Ctrl Pts',(0.4335028573765,-3.926619760277,-3.552424754852));
#47791=CARTESIAN_POINT('Ctrl Pts',(-1.075636817015,-3.801219923529,-3.598466421519));
#47792=CARTESIAN_POINT('Ctrl Pts',(-2.426719472144,-3.117258422503,-3.644508088185));
#47793=CARTESIAN_POINT('Ctrl Pts',(-3.421213323057,-1.975238433022,-3.690549754852));
#47794=CARTESIAN_POINT('Ctrl Pts',(-3.912984720121,-0.5429714994837,-3.736591421519));
#47795=CARTESIAN_POINT('Ctrl Pts',(-3.829771427655,0.969081152984,-3.782633088185));
#47796=CARTESIAN_POINT('Ctrl Pts',(-3.183801034714,2.33873436724,-3.828674754852));
#47797=CARTESIAN_POINT('Ctrl Pts',(-2.069994199668,3.364727549519,-3.874716421519));
#47798=CARTESIAN_POINT('Ctrl Pts',(-0.6520167487486,3.896298452185,-3.920758088185));
#47799=CARTESIAN_POINT('Ctrl Pts',(0.861769828621,3.855336591224,-3.966799754852));
#47800=CARTESIAN_POINT('Ctrl Pts',(2.248925587626,3.247861014648,-4.012841421519));
#47801=CARTESIAN_POINT('Ctrl Pts',(3.305618062651,2.163135847104,-4.058883088185));
#47802=CARTESIAN_POINT('Ctrl Pts',(3.87657396792,0.760553574966,-4.104924754852));
#47803=CARTESIAN_POINT('Ctrl Pts',(3.87789547929,-0.7537865220682,-4.150966421519));
#47804=CARTESIAN_POINT('Ctrl Pts',(3.309388410261,-2.157363163489,-4.197008088185));
#47805=CARTESIAN_POINT('Ctrl Pts',(2.254590746275,-3.243930954253,-4.243049754852));
#47806=CARTESIAN_POINT('Ctrl Pts',(0.8684973443836,-3.853826647885,-4.289091421519));
#47807=CARTESIAN_POINT('Ctrl Pts',(-0.64521543546,-3.897430501112,-4.335133088185));
#47808=CARTESIAN_POINT('Ctrl Pts',(-2.064118492452,-3.368335244341,-4.381174754852));
#47809=CARTESIAN_POINT('Ctrl Pts',(-3.179714326077,-2.344287583402,-4.427216421519));
#47810=CARTESIAN_POINT('Ctrl Pts',(-3.828074229756,-0.9757638856968,-4.473258088185));
#47811=CARTESIAN_POINT('Ctrl Pts',(-3.913926423865,0.5361412292629,-4.519299754852));
#47812=CARTESIAN_POINT('Ctrl Pts',(-3.424655551922,1.969264283907,-4.565341421519));
#47813=CARTESIAN_POINT('Ctrl Pts',(-2.432156415579,3.113018252307,-4.611383088185));
#47814=CARTESIAN_POINT('Ctrl Pts',(-1.082269555721,3.799336794534,-4.657424754852));
#47815=CARTESIAN_POINT('Ctrl Pts',(0.4266489564036,3.927370384378,-4.703466421519));
#47816=CARTESIAN_POINT('Ctrl Pts',(1.872874501785,3.478305416675,-4.749508088185));
#47817=CARTESIAN_POINT('Ctrl Pts',(3.043894742506,2.51812872327,-4.795549754852));
#47818=CARTESIAN_POINT('Ctrl Pts',(3.767636743447,1.187931312243,-4.841591421519));
#47819=CARTESIAN_POINT('Ctrl Pts',(3.937751926915,-0.3168240244129,-4.887633088185));
#47820=CARTESIAN_POINT('Ctrl Pts',(3.529242901566,-1.775024200642,-4.933674754852));
#47821=CARTESIAN_POINT('Ctrl Pts',(2.602137850332,-2.972398097546,-4.979716421519));
#47822=CARTESIAN_POINT('Ctrl Pts',(1.29266533598,-3.73299730079,-5.025758088185));
#47823=CARTESIAN_POINT('Ctrl Pts',(-0.2067467442558,-3.945068533638,-5.071799754852));
#47824=CARTESIAN_POINT('Ctrl Pts',(-1.67580956263,-3.577407472023,-5.117841421519));
#47825=CARTESIAN_POINT('Ctrl Pts',(-2.490943100776,-2.981933138547,-5.148535865963));
#47826=CARTESIAN_POINT('Ctrl Pts',(-2.827595238666,-2.618381900244,-5.163883088185));
#47827=CARTESIAN_POINT('Ctrl Pts',(-3.841349734859,-1.189096377216,-2.31389705505));
#47828=CARTESIAN_POINT('Ctrl Pts',(-3.994234933732,-0.6952040995074,-2.329244277272));
#47829=CARTESIAN_POINT('Ctrl Pts',(-4.10706259235,0.3520715397013,-2.359938721716));
#47830=CARTESIAN_POINT('Ctrl Pts',(-3.672853039324,1.871418570915,-2.405980388383));
#47831=CARTESIAN_POINT('Ctrl Pts',(-2.698930474802,3.115729236588,-2.45202205505));
#47832=CARTESIAN_POINT('Ctrl Pts',(-1.328423408128,3.902218173295,-2.498063721716));
#47833=CARTESIAN_POINT('Ctrl Pts',(0.2372868317335,4.115301255755,-2.544105388383));
#47834=CARTESIAN_POINT('Ctrl Pts',(1.76812922683,3.723671568578,-2.59014705505));
#47835=CARTESIAN_POINT('Ctrl Pts',(3.039157943544,2.784875152802,-2.636188721716));
#47836=CARTESIAN_POINT('Ctrl Pts',(3.863604450802,1.43686161852,-2.682230388383));
#47837=CARTESIAN_POINT('Ctrl Pts',(4.120322345675,-0.1222883131347,-2.72827205505));
#47838=CARTESIAN_POINT('Ctrl Pts',(3.771588791194,-1.663468860739,-2.774313721716));
#47839=CARTESIAN_POINT('Ctrl Pts',(2.868647652528,-2.960214740138,-2.820355388383));
#47840=CARTESIAN_POINT('Ctrl Pts',(1.544179572608,-3.821978559474,-2.86639705505));
#47841=CARTESIAN_POINT('Ctrl Pts',(-0.007194482043365,-4.122130383809,-2.912438721716));
#47842=CARTESIAN_POINT('Ctrl Pts',(-1.557511359811,-3.816565082075,-2.958480388383));
#47843=CARTESIAN_POINT('Ctrl Pts',(-2.8789632535,-2.950183256454,-3.00452205505));
#47844=CARTESIAN_POINT('Ctrl Pts',(-3.777372403381,-1.65029342477,-3.050563721716));
#47845=CARTESIAN_POINT('Ctrl Pts',(-4.120724108895,-0.1079049583238,-3.096605388383));
#47846=CARTESIAN_POINT('Ctrl Pts',(-3.85856533025,1.45033935817,-3.14264705505));
#47847=CARTESIAN_POINT('Ctrl Pts',(-3.029418396237,2.795466837973,-3.188688721716));
#47848=CARTESIAN_POINT('Ctrl Pts',(-1.755120427756,3.7298207659,-3.234730388383));
#47849=CARTESIAN_POINT('Ctrl Pts',(-0.2229202576515,4.11610461728,-3.28077205505));
#47850=CARTESIAN_POINT('Ctrl Pts',(1.342036425525,3.897556785247,-3.326813721716));
#47851=CARTESIAN_POINT('Ctrl Pts',(2.709790601495,3.106291286681,-3.372855388383));
#47852=CARTESIAN_POINT('Ctrl Pts',(3.679360726381,1.858578840628,-3.41889705505));
#47853=CARTESIAN_POINT('Ctrl Pts',(4.108275511099,0.337761730468,-3.464938721716));
#47854=CARTESIAN_POINT('Ctrl Pts',(3.933509042705,-1.232687013245,-3.510980388383));
#47855=CARTESIAN_POINT('Ctrl Pts',(3.180741984619,-2.622001351819,-3.55702205505));
#47856=CARTESIAN_POINT('Ctrl Pts',(1.960587989627,-3.626031632045,-3.603063721716));
#47857=CARTESIAN_POINT('Ctrl Pts',(0.4523398268471,-4.097242895254,-3.649105388383));
#47858=CARTESIAN_POINT('Ctrl Pts',(-1.122376388713,-3.966394068133,-3.69514705505));
#47859=CARTESIAN_POINT('Ctrl Pts',(-2.532167544361,-3.252712435637,-3.741188721716));
#47860=CARTESIAN_POINT('Ctrl Pts',(-3.569875067316,-2.061068331088,-3.787230388383));
#47861=CARTESIAN_POINT('Ctrl Pts',(-4.083015372648,-0.566565202236,-3.83327205505));
#47862=CARTESIAN_POINT('Ctrl Pts',(-3.99618621878,1.011190568834,-3.879313721716));
#47863=CARTESIAN_POINT('Ctrl Pts',(-3.322146519342,2.44035922882,-3.925355388383));
#47864=CARTESIAN_POINT('Ctrl Pts',(-2.159941513463,3.510934821395,-3.97139705505));
#47865=CARTESIAN_POINT('Ctrl Pts',(-0.6803487871228,4.065604037474,-4.017438721716));
#47866=CARTESIAN_POINT('Ctrl Pts',(0.8992162529668,4.022862263621,-4.063480388383));
#47867=CARTESIAN_POINT('Ctrl Pts',(2.346647994561,3.388990093123,-4.10952205505));
#47868=CARTESIAN_POINT('Ctrl Pts',(3.44925685411,2.257130438418,-4.155563721716));
#47869=CARTESIAN_POINT('Ctrl Pts',(4.045022466568,0.7936018564908,-4.201605388383));
#47870=CARTESIAN_POINT('Ctrl Pts',(4.046401401479,-0.7865407553148,-4.24764705505));
#47871=CARTESIAN_POINT('Ctrl Pts',(3.453191034373,-2.251106914784,-4.293688721716));
#47872=CARTESIAN_POINT('Ctrl Pts',(2.352559320954,-3.384889260088,-4.339730388383));
#47873=CARTESIAN_POINT('Ctrl Pts',(0.9062360990033,-4.021286708819,-4.38577205505));
#47874=CARTESIAN_POINT('Ctrl Pts',(-0.6732519368415,-4.066785277243,-4.431813721716));
#47875=CARTESIAN_POINT('Ctrl Pts',(-2.15381048955,-3.514699281129,-4.477855388383));
#47876=CARTESIAN_POINT('Ctrl Pts',(-3.31788223124,-2.446153748497,-4.52389705505));
#47877=CARTESIAN_POINT('Ctrl Pts',(-3.994415272659,-1.018163685866,-4.569938721716));
#47878=CARTESIAN_POINT('Ctrl Pts',(-4.083997996179,0.559438136759,-4.615980388383));
#47879=CARTESIAN_POINT('Ctrl Pts',(-3.573466871112,2.054834587688,-4.66202205505));
#47880=CARTESIAN_POINT('Ctrl Pts',(-2.537840738919,3.248288017621,-4.708063721716));
#47881=CARTESIAN_POINT('Ctrl Pts',(-1.129297339352,3.964429111665,-4.754105388383));
#47882=CARTESIAN_POINT('Ctrl Pts',(0.4451881037926,4.098026136172,-4.80014705505));
#47883=CARTESIAN_POINT('Ctrl Pts',(1.954256387077,3.629447979702,-4.846188721716));
#47884=CARTESIAN_POINT('Ctrl Pts',(3.176160888763,2.627548795309,-4.892230388383));
#47885=CARTESIAN_POINT('Ctrl Pts',(3.931351600467,1.239550408822,-4.93827205505));
#47886=CARTESIAN_POINT('Ctrl Pts',(4.108858787154,-0.3305909566808,-4.984313721716));
#47887=CARTESIAN_POINT('Ctrl Pts',(3.682598847576,-1.852154203613,-5.030355388383));
#47888=CARTESIAN_POINT('Ctrl Pts',(2.715208365118,-3.101557505068,-5.07639705505));
#47889=CARTESIAN_POINT('Ctrl Pts',(1.348835432798,-3.89520697252,-5.122438721716));
#47890=CARTESIAN_POINT('Ctrl Pts',(-0.2157304961352,-4.116493321879,-5.168480388383));
#47891=CARTESIAN_POINT('Ctrl Pts',(-1.748628398844,-3.732856309759,-5.21452205505));
#47892=CARTESIAN_POINT('Ctrl Pts',(-2.599181877855,-3.111506871542,-5.245216499494));
#47893=CARTESIAN_POINT('Ctrl Pts',(-2.950462537646,-2.7321582666,-5.260563721716));
#47894=CARTESIAN_POINT('',(-3.93909072274296,0.694567964780147,-2.35825152239436));
#47895=CARTESIAN_POINT('Ctrl Pts',(-1.36801982010901,-3.75859882970906,
-4.44169936887435));
#47896=CARTESIAN_POINT('Ctrl Pts',(-1.16576578312669,-3.83216333246039,
-4.43524390841633));
#47897=CARTESIAN_POINT('Ctrl Pts',(-0.957575527497493,-3.88947208452673,
-4.42876047910253));
#47898=CARTESIAN_POINT('Ctrl Pts',(-0.536796172629159,-3.96949863700133,
-4.41599000469032));
#47899=CARTESIAN_POINT('Ctrl Pts',(-0.324896257588679,-3.99243262327782,
-4.40974678199487));
#47900=CARTESIAN_POINT('Ctrl Pts',(0.308796827379884,-4.00997416051721,
-4.39084393819084));
#47901=CARTESIAN_POINT('Ctrl Pts',(0.731667503869158,-3.95512345077563,
-4.37811939203431));
#47902=CARTESIAN_POINT('Ctrl Pts',(1.5146514617827,-3.72296528639292,-4.35394723701022));
#47903=CARTESIAN_POINT('Ctrl Pts',(1.87461764815377,-3.55500354569365,-4.34205069592721));
#47904=CARTESIAN_POINT('Ctrl Pts',(2.41773986304984,-3.19701093090743,-4.32265348722271));
#47905=CARTESIAN_POINT('Ctrl Pts',(2.61842108636455,-3.03478219072031,-4.31510650260857));
#47906=CARTESIAN_POINT('Ctrl Pts',(2.99084947506056,-2.66884817888097,-4.29948206288811));
#47907=CARTESIAN_POINT('Ctrl Pts',(3.16094151410186,-2.46511362780033,-4.29150861837212));
#47908=CARTESIAN_POINT('Ctrl Pts',(3.45486522391036,-2.03243284581852,-4.27592206267503));
#47909=CARTESIAN_POINT('Ctrl Pts',(3.57889457870004,-1.80498630056301,-4.26834080484933));
#47910=CARTESIAN_POINT('Ctrl Pts',(3.78358421801442,-1.32374735077988,-4.25268267517954));
#47911=CARTESIAN_POINT('Ctrl Pts',(3.86291241695182,-1.07063456334499,-4.24471507975128));
#47912=CARTESIAN_POINT('Ctrl Pts',(3.9562346792498,-0.621236099015068,-4.23104966239667));
#47913=CARTESIAN_POINT('Ctrl Pts',(3.98179879462672,-0.42778244620501,-4.22532655594778));
#47914=CARTESIAN_POINT('Ctrl Pts',(4.0006808351246,-0.102475082871344,-4.21561255270373));
#47915=CARTESIAN_POINT('Ctrl Pts',(4.00184602497239,0.0283802363947507,
-4.2116916302295));
#47916=CARTESIAN_POINT('Ctrl Pts',(3.98631881005115,0.417925330358341,-4.19998549294754));
#47917=CARTESIAN_POINT('Ctrl Pts',(3.95094450054871,0.676006772840593,-4.19220583507454));
#47918=CARTESIAN_POINT('Ctrl Pts',(3.83009212472557,1.18237705257788,-4.17679517875193));
#47919=CARTESIAN_POINT('Ctrl Pts',(3.74482524678116,1.42917791521534,-4.16905051371582));
#47920=CARTESIAN_POINT('Ctrl Pts',(3.41725214324585,2.14415260468746,-4.14543441353372));
#47921=CARTESIAN_POINT('Ctrl Pts',(3.10715307845772,2.57323464944538,-4.13013006234986));
#47922=CARTESIAN_POINT('Ctrl Pts',(2.33529076991263,3.28964516038514,-4.09850418891609));
#47923=CARTESIAN_POINT('Ctrl Pts',(1.88427861435023,3.56721619917969,-4.08319599107816));
#47924=CARTESIAN_POINT('Ctrl Pts',(0.897021813530376,3.93331136940216,-4.05157410615685));
#47925=CARTESIAN_POINT('Ctrl Pts',(0.374300849531254,4.01683103674258,-4.03627217052875));
#47926=CARTESIAN_POINT('Ctrl Pts',(-0.406700731577845,3.98726923128037,
-4.0128015836215));
#47927=CARTESIAN_POINT('Ctrl Pts',(-0.66077444767884,3.95328764135642,-4.00518628092756));
#47928=CARTESIAN_POINT('Ctrl Pts',(-1.29629263820266,3.80479144684892,-3.98587135179335));
#47929=CARTESIAN_POINT('Ctrl Pts',(-1.66787074979849,3.65684562290541,-3.97389855805407));
#47930=CARTESIAN_POINT('Ctrl Pts',(-2.23256055970333,3.32895355733969,-3.95442486435378));
#47931=CARTESIAN_POINT('Ctrl Pts',(-2.44198852664714,3.17846702206362,-3.946883162998));
#47932=CARTESIAN_POINT('Ctrl Pts',(-2.83449224071045,2.83436117767312,-3.93126411001548));
#47933=CARTESIAN_POINT('Ctrl Pts',(-3.0158923819255,2.6405924163579,-3.92328975695283));
#47934=CARTESIAN_POINT('Ctrl Pts',(-3.25419004520932,2.32939589011373,-3.9116087917026));
#47935=CARTESIAN_POINT('Ctrl Pts',(-3.32684711275221,2.22440626126068,-3.90784050717486));
#47936=CARTESIAN_POINT('Ctrl Pts',(-3.53098322623027,1.8968969600739,-3.8964136633248));
#47937=CARTESIAN_POINT('Ctrl Pts',(-3.64591334087103,1.66489092518052,-3.88867432414806));
#47938=CARTESIAN_POINT('Ctrl Pts',(-3.82773226754075,1.18788211445012,-3.87334723842088));
#47939=CARTESIAN_POINT('Ctrl Pts',(-3.89534807804564,0.943441021874519,
-3.86583135445027));
#47940=CARTESIAN_POINT('Ctrl Pts',(-3.98410455565061,0.439436441188183,
-3.85068053490909));
#47941=CARTESIAN_POINT('Ctrl Pts',(-4.00398113926887,0.181108493150542,
-3.84293962576666));
#47942=CARTESIAN_POINT('Ctrl Pts',(-3.99423618289338,-0.330039477952322,
-3.82758902240187));
#47943=CARTESIAN_POINT('Ctrl Pts',(-3.96543189641876,-0.58262904558535,
-3.82005114587486));
#47944=CARTESIAN_POINT('Ctrl Pts',(-3.85892978523262,-1.08395434249013,
-3.80487945555321));
#47945=CARTESIAN_POINT('Ctrl Pts',(-3.78060972657924,-1.33107125885623,
-3.79713742203396));
#47946=CARTESIAN_POINT('Ctrl Pts',(-3.57995899763623,-1.80192518325927,
-3.78176871778775));
#47947=CARTESIAN_POINT('Ctrl Pts',(-3.45842129682671,-2.0257467495555,-3.77421392571749));
#47948=CARTESIAN_POINT('Ctrl Pts',(-3.17149943533642,-2.45111546943147,
-3.75902611469025));
#47949=CARTESIAN_POINT('Ctrl Pts',(-3.00620636341425,-2.65095450340893,
-3.75128326582865));
#47950=CARTESIAN_POINT('Ctrl Pts',(-2.6433796264621,-3.01259572402451,-3.73590056199311));
#47951=CARTESIAN_POINT('Ctrl Pts',(-2.44651657896266,-3.17475265057089,
-3.72833268979306));
#47952=CARTESIAN_POINT('Ctrl Pts',(-1.91004887642632,-3.53622917907652,
-3.70918533237558));
#47953=CARTESIAN_POINT('Ctrl Pts',(-1.5531977730994,-3.70654199789545,-3.69733967918743));
#47954=CARTESIAN_POINT('Ctrl Pts',(-0.93327777387392,-3.8981283944329,-3.6779928280832));
#47955=CARTESIAN_POINT('Ctrl Pts',(-0.680381380773941,-3.95008448602936,
-3.67044165819892));
#47956=CARTESIAN_POINT('Ctrl Pts',(-0.161076721039697,-4.0052428935594,
-3.65481304613054));
#47957=CARTESIAN_POINT('Ctrl Pts',(0.104301390506375,-4.00717576675699,
-3.64684029502901));
#47958=CARTESIAN_POINT('Ctrl Pts',(0.625265129427227,-3.95929015152296,
-3.63125258223983));
#47959=CARTESIAN_POINT('Ctrl Pts',(0.87982060422287,-3.91055295484658,-3.62366736051567));
#47960=CARTESIAN_POINT('Ctrl Pts',(1.38158822702633,-3.76284716596401,-3.60800540595417));
#47961=CARTESIAN_POINT('Ctrl Pts',(1.62743767511326,-3.66330469915853,-3.60003846977951));
#47962=CARTESIAN_POINT('Ctrl Pts',(2.02885592414387,-3.45243856135319,-3.58653982988137));
#47963=CARTESIAN_POINT('Ctrl Pts',(2.19000915014392,-3.35252857713794,-3.58097703367505));
#47964=CARTESIAN_POINT('Ctrl Pts',(2.44953544757942,-3.16477022048459,-3.5714321033113));
#47965=CARTESIAN_POINT('Ctrl Pts',(2.55168647331349,-3.08293791440222,-3.56751139854109));
#47966=CARTESIAN_POINT('Ctrl Pts',(2.8438699920888,-2.82451366131099,-3.55579962007338));
#47967=CARTESIAN_POINT('Ctrl Pts',(3.02162263004526,-2.63378253177322,-3.54800841374717));
#47968=CARTESIAN_POINT('Ctrl Pts',(3.33774443191726,-2.21972629663611,-3.53258525939748));
#47969=CARTESIAN_POINT('Ctrl Pts',(3.47511454605587,-1.99749597997082,-3.52484244301243));
#47970=CARTESIAN_POINT('Ctrl Pts',(3.70417329294106,-1.53116578729521,-3.50924166680827));
#47971=CARTESIAN_POINT('Ctrl Pts',(3.79596336309501,-1.28747036077039,-3.5014660396352));
#47972=CARTESIAN_POINT('Ctrl Pts',(3.93086443146694,-0.784789241119805,
-3.48605966099206));
#47973=CARTESIAN_POINT('Ctrl Pts',(3.97344498876691,-0.527215712248708,
-3.47831454476549));
#47974=CARTESIAN_POINT('Ctrl Pts',(4.02601313000844,0.257441192337123,-3.45469896792346));
#47975=CARTESIAN_POINT('Ctrl Pts',(3.95773352554131,0.782460838811398,-3.43939392117451));
#47976=CARTESIAN_POINT('Ctrl Pts',(3.70638867520848,1.52560960247683,-3.41583418645671));
#47977=CARTESIAN_POINT('Ctrl Pts',(3.60030600780396,1.76184934909529,-3.4081188962284));
#47978=CARTESIAN_POINT('Ctrl Pts',(3.21249126105984,2.43978950749078,-3.38500568355129));
#47979=CARTESIAN_POINT('Ctrl Pts',(2.8656607839029,2.83911477915266,-3.36926436353717));
#47980=CARTESIAN_POINT('Ctrl Pts',(2.0402068906059,3.47995424644701,-3.33833955282941));
#47981=CARTESIAN_POINT('Ctrl Pts',(1.56730987495655,3.71703270463164,-3.32259648616218));
#47982=CARTESIAN_POINT('Ctrl Pts',(0.813701158858086,3.92485852491073,-3.29946126283233));
#47983=CARTESIAN_POINT('Ctrl Pts',(0.557869758702243,3.96911471734924,-3.2917213834433));
#47984=CARTESIAN_POINT('Ctrl Pts',(0.040895471393891,4.0080431421574,-3.27615229447875));
#47985=CARTESIAN_POINT('Ctrl Pts',(-0.220021179035145,4.00238598974046,
-3.26840176631272));
#47986=CARTESIAN_POINT('Ctrl Pts',(-0.736359771982586,3.94012535110111,
-3.25300910270255));
#47987=CARTESIAN_POINT('Ctrl Pts',(-0.990294423548421,3.88388772859838,
-3.24524995137463));
#47988=CARTESIAN_POINT('Ctrl Pts',(-1.48398117232706,3.72344751635879,-3.22966151377038));
#47989=CARTESIAN_POINT('Ctrl Pts',(-1.72338094316868,3.61905993450343,-3.22191257145241));
#47990=CARTESIAN_POINT('Ctrl Pts',(-2.17787908259835,3.36508644455266,-3.20650121339441));
#47991=CARTESIAN_POINT('Ctrl Pts',(-2.39173715943083,3.21636544996632,-3.19872394421881));
#47992=CARTESIAN_POINT('Ctrl Pts',(-2.78788754242832,2.87995408720518,-3.18311797697578));
#47993=CARTESIAN_POINT('Ctrl Pts',(-2.96976345003142,2.69226206636054,-3.17537166592776));
#47994=CARTESIAN_POINT('Ctrl Pts',(-3.2938413076201,2.2842181674067,-3.15994447507618));
#47995=CARTESIAN_POINT('Ctrl Pts',(-3.43523185049853,2.06511106675781,-3.15215229730507));
#47996=CARTESIAN_POINT('Ctrl Pts',(-3.61420770737158,1.71846211251952,-3.14043876845689));
#47997=CARTESIAN_POINT('Ctrl Pts',(-3.66851681395888,1.59936773833699,-3.1365177963949));
#47998=CARTESIAN_POINT('Ctrl Pts',(-3.78741883704035,1.30058477932089,-3.12693529515567));
#47999=CARTESIAN_POINT('Ctrl Pts',(-3.84508629152518,1.11864882035746,-3.12133642896898));
#48000=CARTESIAN_POINT('Ctrl Pts',(-3.95104286114496,0.676470454311608,
-3.10779894402269));
#48001=CARTESIAN_POINT('Ctrl Pts',(-3.98706500780911,0.413676356601029,
-3.09983141354669));
#48002=CARTESIAN_POINT('Ctrl Pts',(-4.00681406888649,-0.108778943815362,
-3.08417712951966));
#48003=CARTESIAN_POINT('Ctrl Pts',(-3.99148210100408,-0.36725844207694,
-3.07659954287649));
#48004=CARTESIAN_POINT('Ctrl Pts',(-3.9098912479272,-0.883792825718099,
-3.0610174220215));
#48005=CARTESIAN_POINT('Ctrl Pts',(-3.84278805097487,-1.14057416481873,
-3.05304400200963));
#48006=CARTESIAN_POINT('Ctrl Pts',(-3.66176050597667,-1.63017617463855,
-3.037422922239));
#48007=CARTESIAN_POINT('Ctrl Pts',(-3.54936799047195,-1.86232897513618,
-3.02987925632651));
#48008=CARTESIAN_POINT('Ctrl Pts',(-3.2117528499792,-2.41560879945962,-3.01055241293434));
#48009=CARTESIAN_POINT('Ctrl Pts',(-2.95935888672256,-2.71938297014093,
-2.9987207473539));
#48010=CARTESIAN_POINT('Ctrl Pts',(-2.47742066852805,-3.15072353736212,
-2.97957666314663));
#48011=CARTESIAN_POINT('Ctrl Pts',(-2.27163322531345,-3.3019753608914,-2.97199852589408));
#48012=CARTESIAN_POINT('Ctrl Pts',(-1.83154094554953,-3.56516244550671,
-2.95660050003261));
#48013=CARTESIAN_POINT('Ctrl Pts',(-1.59707594248354,-3.67638616105042,
-2.94885314655851));
#48014=CARTESIAN_POINT('Ctrl Pts',(-1.11367518200821,-3.85023145239489,
-2.93364721253502));
#48015=CARTESIAN_POINT('Ctrl Pts',(-0.866403969682855,-3.91313184871958,
-2.92607812745012));
#48016=CARTESIAN_POINT('Ctrl Pts',(-0.360022481771758,-3.99189874134353,
-2.91068981694937));
#48017=CARTESIAN_POINT('Ctrl Pts',(-0.101032384666768,-4.00701925018241,
-2.90294304494526));
#48018=CARTESIAN_POINT('Ctrl Pts',(0.411881876223697,-3.9868228340172,-2.88774824810053));
#48019=CARTESIAN_POINT('Ctrl Pts',(0.664378073671907,-3.95243301126028,
-2.88019081295765));
#48020=CARTESIAN_POINT('Ctrl Pts',(1.1629544280647,-3.83566694225597,-2.86481501077947));
#48021=CARTESIAN_POINT('Ctrl Pts',(1.40862781016742,-3.75261330799575,-2.85706902662035));
#48022=CARTESIAN_POINT('Ctrl Pts',(1.87609365122038,-3.54181851853787,-2.84188859914504));
#48023=CARTESIAN_POINT('Ctrl Pts',(2.09694446312091,-3.41552013962223,-2.83434623395034));
#48024=CARTESIAN_POINT('Ctrl Pts',(2.51504445396781,-3.12078029921391,-2.81898661662597));
#48025=CARTESIAN_POINT('Ctrl Pts',(2.71162733856537,-2.95183390214576,-2.81124171364893));
#48026=CARTESIAN_POINT('Ctrl Pts',(3.06566136120269,-2.58179553922187,-2.79607991691089));
#48027=CARTESIAN_POINT('Ctrl Pts',(3.22284597780397,-2.38243455028453,-2.78855715517691));
#48028=CARTESIAN_POINT('Ctrl Pts',(3.49992739201803,-1.95323289660394,-2.77321859195396));
#48029=CARTESIAN_POINT('Ctrl Pts',(3.61895804909156,-1.72315656774654,-2.76547519260078));
#48030=CARTESIAN_POINT('Ctrl Pts',(3.76217493501356,-1.364537735472,-2.75404121352314));
#48031=CARTESIAN_POINT('Ctrl Pts',(3.80381657658998,-1.24372274051385,-2.75026968632714));
#48032=CARTESIAN_POINT('Ctrl Pts',(3.94531393268906,-0.758491646702463,
-2.7352066494307));
#48033=CARTESIAN_POINT('Ctrl Pts',(3.99971098138022,-0.380629373148319,
-2.72374973626902));
#48034=CARTESIAN_POINT('Ctrl Pts',(4.0000134136939,0.125170532368751,-2.70876711063907));
#48035=CARTESIAN_POINT('Ctrl Pts',(3.99401009623935,0.252250110774488,-2.70501503313205));
#48036=CARTESIAN_POINT('Ctrl Pts',(3.9568297462809,0.641754190918649,-2.69336498465536));
#48037=CARTESIAN_POINT('Ctrl Pts',(3.90565723780332,0.902033904090278,-2.6853970084711));
#48038=CARTESIAN_POINT('Ctrl Pts',(3.75487916969687,1.40258446379034,-2.66974521500997));
#48039=CARTESIAN_POINT('Ctrl Pts',(3.65656300521899,1.64204648993718,-2.66217022491873));
#48040=CARTESIAN_POINT('Ctrl Pts',(3.41187927734039,2.10414329315607,-2.64658894383737));
#48041=CARTESIAN_POINT('Ctrl Pts',(3.2651135487979,2.32528966893541,-2.6386150815753));
#48042=CARTESIAN_POINT('Ctrl Pts',(2.93511444117701,2.72965813373484,-2.62299657363307));
#48043=CARTESIAN_POINT('Ctrl Pts',(2.75356053688138,2.91275559104162,-2.61545546965109));
#48044=CARTESIAN_POINT('Ctrl Pts',(2.25387975142308,3.32738646981954,-2.59609326195907));
#48045=CARTESIAN_POINT('Ctrl Pts',(1.91544238363832,3.53340209283841,-2.5842260236807));
#48046=CARTESIAN_POINT('Ctrl Pts',(1.3179570910716,3.78521221421753,-2.56503529692822));
#48047=CARTESIAN_POINT('Ctrl Pts',(1.07381676479304,3.86140191952328,-2.55744394020935));
#48048=CARTESIAN_POINT('Ctrl Pts',(0.309698104580703,4.02229514523478,-2.53399511988193));
#48049=CARTESIAN_POINT('Ctrl Pts',(-0.219451971089868,4.02834519965438,
-2.5186969990541));
#48050=CARTESIAN_POINT('Ctrl Pts',(-1.25427613962423,3.83433141908602,-2.48707849671069));
#48051=CARTESIAN_POINT('Ctrl Pts',(-1.74569708460653,3.63704011328204,-2.47177159325893));
#48052=CARTESIAN_POINT('Ctrl Pts',(-2.62748994927562,3.06137544257374,-2.44014611995675));
#48053=CARTESIAN_POINT('Ctrl Pts',(-3.00575665316205,2.69084249663867,-2.42483886577149));
#48054=CARTESIAN_POINT('Ctrl Pts',(-3.38241896388994,2.13955135107824,-2.40478833402707));
#48055=CARTESIAN_POINT('Ctrl Pts',(-3.4560224092977,2.01859946390072,-2.4005448130044));
#48056=CARTESIAN_POINT('Ctrl Pts',(-3.62315488767914,1.70795073884791,-2.39002940232023));
#48057=CARTESIAN_POINT('Ctrl Pts',(-3.70821877218224,1.51441198273768,-2.38383620017788));
#48058=CARTESIAN_POINT('Ctrl Pts',(-3.84786718848642,1.11277137122209,-2.37115638012773));
#48059=CARTESIAN_POINT('Ctrl Pts',(-3.90187360705131,0.90513993314234,-2.36471469938033));
#48060=CARTESIAN_POINT('Ctrl Pts',(-3.93905195666665,0.694559625484905,
-2.35830063501608));
#48061=CARTESIAN_POINT('',(-3.4862157938408,0.614712896413036,-2.09242018782987));
#48062=CARTESIAN_POINT('',(-3.486219445663,0.6147145489409,-2.092752209506));
#48063=CARTESIAN_POINT('',(-1.21075130737245,-3.32651187758048,-4.92608554278596));
#48064=CARTESIAN_POINT('Ctrl Pts',(-3.48611163489721,0.614695485491625,
-2.092752209506));
#48065=CARTESIAN_POINT('Ctrl Pts',(-3.45247823923436,0.804904617636082,
-2.099265619468));
#48066=CARTESIAN_POINT('Ctrl Pts',(-3.40329486078118,0.992351978567723,
-2.1057790294295));
#48067=CARTESIAN_POINT('Ctrl Pts',(-3.33926661181778,1.17458628760328,-2.11229243939108));
#48068=CARTESIAN_POINT('Ctrl Pts',(-3.28724381166632,1.32265123070542,-2.11758456950899));
#48069=CARTESIAN_POINT('Ctrl Pts',(-3.22541325987337,1.46728788207019,-2.12287669962695));
#48070=CARTESIAN_POINT('Ctrl Pts',(-3.15416309562667,1.60712636907785,-2.12816882974492));
#48071=CARTESIAN_POINT('Ctrl Pts',(-3.13772049359028,1.63939729245812,-2.12939010958862));
#48072=CARTESIAN_POINT('Ctrl Pts',(-3.12077629297601,1.67141270174591,-2.13061138943231));
#48073=CARTESIAN_POINT('Ctrl Pts',(-3.10334122949876,1.70315880781664,-2.13183266927601));
#48074=CARTESIAN_POINT('Ctrl Pts',(-3.010355402605,1.87246922802227,-2.13834607923767));
#48075=CARTESIAN_POINT('Ctrl Pts',(-2.90342002496954,2.03409949917319,-2.14485948919933));
#48076=CARTESIAN_POINT('Ctrl Pts',(-2.78413804221371,2.18602098504228,-2.15137289916099));
#48077=CARTESIAN_POINT('Ctrl Pts',(-2.66485605945771,2.33794247091159,-2.15788630912266));
#48078=CARTESIAN_POINT('Ctrl Pts',(-2.53321256598554,2.48017394117643,-2.16439971908433));
#48079=CARTESIAN_POINT('Ctrl Pts',(-2.39079396961086,2.61067055624253,-2.170913129046));
#48080=CARTESIAN_POINT('Ctrl Pts',(-2.36676052640752,2.63269213956278,-2.17201228092896));
#48081=CARTESIAN_POINT('Ctrl Pts',(-2.34242073842935,2.65437904749335,-2.17311143281192));
#48082=CARTESIAN_POINT('Ctrl Pts',(-2.3177824805595,2.6757212808535,-2.17421058469488));
#48083=CARTESIAN_POINT('Ctrl Pts',(-2.19641810063612,2.78084993611871,-2.17962484277359));
#48084=CARTESIAN_POINT('Ctrl Pts',(-2.06781106235418,2.87761446755544,-2.18503910085229));
#48085=CARTESIAN_POINT('Ctrl Pts',(-1.93328280840194,2.96525962093555,-2.190453358931));
#48086=CARTESIAN_POINT('Ctrl Pts',(-1.7714438903673,3.07069767113915,-2.19696676889267));
#48087=CARTESIAN_POINT('Ctrl Pts',(-1.6010187810845,3.16295401534946,-2.20348017885433));
#48088=CARTESIAN_POINT('Ctrl Pts',(-1.42421971206299,3.24075297381787,-2.20999358881617));
#48089=CARTESIAN_POINT('Ctrl Pts',(-1.33140030198562,3.28159738249964,-2.21341312531936));
#48090=CARTESIAN_POINT('Ctrl Pts',(-1.23682153800335,3.31845691336659,-2.2168326618226));
#48091=CARTESIAN_POINT('Ctrl Pts',(-1.14082056111593,3.35113838080967,-2.22025219832584));
#48092=CARTESIAN_POINT('Ctrl Pts',(-1.05396233511999,3.38070739538729,-2.22334607178452));
#48093=CARTESIAN_POINT('Ctrl Pts',(-0.965939942205691,3.40685628944164,
-2.2264399452432));
#48094=CARTESIAN_POINT('Ctrl Pts',(-0.877038495435007,3.42954597194126,
-2.22953381870184));
#48095=CARTESIAN_POINT('Ctrl Pts',(-0.689877780312868,3.47731366703263,
-2.23604722866367));
#48096=CARTESIAN_POINT('Ctrl Pts',(-0.498817901017613,3.50975420229228,
-2.24256063862533));
#48097=CARTESIAN_POINT('Ctrl Pts',(-0.306392768733605,3.52652952279029,
-2.24907404858699));
#48098=CARTESIAN_POINT('Ctrl Pts',(-0.136818383836607,3.54131275105748,
-2.25481398221583));
#48099=CARTESIAN_POINT('Ctrl Pts',(0.0338347226870868,3.54392884861796,
-2.26055391584467));
#48100=CARTESIAN_POINT('Ctrl Pts',(0.203776655436933,3.53413003081367,-2.2662938494735));
#48101=CARTESIAN_POINT('Ctrl Pts',(0.226676931195759,3.53280960550016,-2.26706732580633));
#48102=CARTESIAN_POINT('Ctrl Pts',(0.249564290458189,3.53126376392604,-2.26784080213917));
#48103=CARTESIAN_POINT('Ctrl Pts',(0.27243444834103,3.52949358819305,-2.268614278472));
#48104=CARTESIAN_POINT('Ctrl Pts',(0.46502303554917,3.51458701670047,-2.27512768843367));
#48105=CARTESIAN_POINT('Ctrl Pts',(0.656363625397378,3.4837751352979,-2.28164109839533));
#48106=CARTESIAN_POINT('Ctrl Pts',(0.843944386843304,3.43771235132368,-2.288154508357));
#48107=CARTESIAN_POINT('Ctrl Pts',(1.03152514828923,3.39164956734945,-2.29466791831867));
#48108=CARTESIAN_POINT('Ctrl Pts',(1.21536958570617,3.33033103466894,-2.30118132828033));
#48109=CARTESIAN_POINT('Ctrl Pts',(1.39297675817359,3.25438475836223,-2.307694738242));
#48110=CARTESIAN_POINT('Ctrl Pts',(1.43515898045606,3.23634729588709,-2.3092416921347));
#48111=CARTESIAN_POINT('Ctrl Pts',(1.47698836004088,3.2174850491827,-2.3107886460274));
#48112=CARTESIAN_POINT('Ctrl Pts',(1.5184303722474,3.19780693673633,-2.3123355999201));
#48113=CARTESIAN_POINT('Ctrl Pts',(1.65147889683793,3.13463085796226,-2.31730205598907));
#48114=CARTESIAN_POINT('Ctrl Pts',(1.78053424961026,3.06304474292021,-2.32226851205804));
#48115=CARTESIAN_POINT('Ctrl Pts',(1.90464785652295,2.98375084516111,-2.32723496812701));
#48116=CARTESIAN_POINT('Ctrl Pts',(2.06742042360426,2.87975844970031,-2.33374837808867));
#48117=CARTESIAN_POINT('Ctrl Pts',(2.22171376607907,2.76250122118534,-2.34026178805033));
#48118=CARTESIAN_POINT('Ctrl Pts',(2.36547392639545,2.63349262599518,-2.34677519801199));
#48119=CARTESIAN_POINT('Ctrl Pts',(2.45083123681511,2.55689402814848,-2.35064252227459));
#48120=CARTESIAN_POINT('Ctrl Pts',(2.53247769695781,2.47614836598736,-2.35450984653719));
#48121=CARTESIAN_POINT('Ctrl Pts',(2.609961772308,2.3915893349595,-2.3583771707998));
#48122=CARTESIAN_POINT('Ctrl Pts',(2.66297762765571,2.3337326807108,-2.36102325649886));
#48123=CARTESIAN_POINT('Ctrl Pts',(2.71404492982089,2.27409090047738,-2.36366934219792));
#48124=CARTESIAN_POINT('Ctrl Pts',(2.7630696354151,2.21281727982083,-2.36631542789698));
#48125=CARTESIAN_POINT('Ctrl Pts',(2.88374524539246,2.06199064132035,-2.37282883785867));
#48126=CARTESIAN_POINT('Ctrl Pts',(2.99204550459216,1.90128017903614,-2.37934224782037));
#48127=CARTESIAN_POINT('Ctrl Pts',(3.08664143368824,1.73287520944786,-2.38585565778207));
#48128=CARTESIAN_POINT('Ctrl Pts',(3.17650752923906,1.57289055436952,-2.39204339469183));
#48129=CARTESIAN_POINT('Ctrl Pts',(3.2540133932933,1.40594134449907,-2.39823113160158));
#48130=CARTESIAN_POINT('Ctrl Pts',(3.317978242801,1.23394504751905,-2.40441886851134));
#48131=CARTESIAN_POINT('Ctrl Pts',(3.32134484161676,1.22489253611342,-2.40474454156322));
#48132=CARTESIAN_POINT('Ctrl Pts',(3.32467393213607,1.21582604517722,-2.40507021461511));
#48133=CARTESIAN_POINT('Ctrl Pts',(3.32796545991406,1.20674589826919,-2.405395887667));
#48134=CARTESIAN_POINT('Ctrl Pts',(3.39379549925573,1.02514438416957,-2.41190929762864));
#48135=CARTESIAN_POINT('Ctrl Pts',(3.4445898638602,0.838110253654046,-2.41842270759027));
#48136=CARTESIAN_POINT('Ctrl Pts',(3.47993533170847,0.648217911398604,-2.42493611755191));
#48137=CARTESIAN_POINT('Ctrl Pts',(3.51528079955726,0.458325569140407,-2.43144952751364));
#48138=CARTESIAN_POINT('Ctrl Pts',(3.53518366555639,0.265551810365206,-2.43796293747537));
#48139=CARTESIAN_POINT('Ctrl Pts',(3.53921587207989,0.0724312289064312,
-2.44447634743708));
#48140=CARTESIAN_POINT('Ctrl Pts',(3.5404507477039,0.0132874580830817,-2.44647109922969));
#48141=CARTESIAN_POINT('Ctrl Pts',(3.54019686595504,-0.0458877048812477,
-2.44846585102229));
#48142=CARTESIAN_POINT('Ctrl Pts',(3.53844190482233,-0.105018504061302,
-2.4504606028149));
#48143=CARTESIAN_POINT('Ctrl Pts',(3.53446643805599,-0.238965930375457,
-2.4549792609839));
#48144=CARTESIAN_POINT('Ctrl Pts',(3.52278756542149,-0.372685587266579,
-2.45949791915291));
#48145=CARTESIAN_POINT('Ctrl Pts',(3.50360264434659,-0.505307275679988,
-2.46401657732192));
#48146=CARTESIAN_POINT('Ctrl Pts',(3.47594858170895,-0.69647451917164,-2.47052998728364));
#48147=CARTESIAN_POINT('Ctrl Pts',(3.43270056047567,-0.885379751350099,
-2.47704339724537));
#48148=CARTESIAN_POINT('Ctrl Pts',(3.37442090167997,-1.06953540954889,-2.4835568072071));
#48149=CARTESIAN_POINT('Ctrl Pts',(3.33581079605796,-1.19153800120563,-2.48787192249395));
#48150=CARTESIAN_POINT('Ctrl Pts',(3.29059905133193,-1.31146265306598,-2.4921870377808));
#48151=CARTESIAN_POINT('Ctrl Pts',(3.23895722418867,-1.42855034908728,-2.49650215306765));
#48152=CARTESIAN_POINT('Ctrl Pts',(3.21264878372798,-1.48819956852543,-2.49870044774243));
#48153=CARTESIAN_POINT('Ctrl Pts',(3.18467168469657,-1.54711255044106,-2.50089874241722));
#48154=CARTESIAN_POINT('Ctrl Pts',(3.15508456246594,-1.60520476755959,-2.503097037092));
#48155=CARTESIAN_POINT('Ctrl Pts',(3.06741976534675,-1.77732838229316,-2.50961044705364));
#48156=CARTESIAN_POINT('Ctrl Pts',(2.96562690748144,-1.94223957070431,-2.51612385701527));
#48157=CARTESIAN_POINT('Ctrl Pts',(2.85118122343503,-2.0978372735158,-2.52263726697691));
#48158=CARTESIAN_POINT('Ctrl Pts',(2.73673553938697,-2.25343497632954,-2.52915067693864));
#48159=CARTESIAN_POINT('Ctrl Pts',(2.60962088951851,-2.39973705663602,-2.53566408690037));
#48160=CARTESIAN_POINT('Ctrl Pts',(2.47132239430563,-2.53459348728904,-2.54217749686209));
#48161=CARTESIAN_POINT('Ctrl Pts',(2.4687292831959,-2.53712205933177,-2.54229962397351));
#48162=CARTESIAN_POINT('Ctrl Pts',(2.46613224843455,-2.5396465996386,-2.54242175108493));
#48163=CARTESIAN_POINT('Ctrl Pts',(2.463531299937,-2.54216709408167,-2.54254387819635));
#48164=CARTESIAN_POINT('Ctrl Pts',(2.32741576151579,-2.67407222735452,-2.54893516104657));
#48165=CARTESIAN_POINT('Ctrl Pts',(2.18058121321383,-2.79489605595183,-2.55532644389679));
#48166=CARTESIAN_POINT('Ctrl Pts',(2.02510726029512,-2.90329545916035,-2.56171772674717));
#48167=CARTESIAN_POINT('Ctrl Pts',(1.8666624507869,-3.01376620020569,-2.56823113670897));
#48168=CARTESIAN_POINT('Ctrl Pts',(1.69922697758555,-3.11134926906942,-2.57474454667094));
#48169=CARTESIAN_POINT('Ctrl Pts',(1.52494467780377,-3.19463871795646,-2.58125795663274));
#48170=CARTESIAN_POINT('Ctrl Pts',(1.45958838442203,-3.22587246724644,-2.58370050147471));
#48171=CARTESIAN_POINT('Ctrl Pts',(1.39326974838671,-3.25509547106922,-2.58614304631666));
#48172=CARTESIAN_POINT('Ctrl Pts',(1.32610734069228,-3.28223084516667,-2.5885855911586));
#48173=CARTESIAN_POINT('Ctrl Pts',(1.21417117552754,-3.32745599151041,-2.59265645627845));
#48174=CARTESIAN_POINT('Ctrl Pts',(1.09989117051022,-3.3668818964363,-2.59672732139827));
#48175=CARTESIAN_POINT('Ctrl Pts',(0.983909678540035,-3.40038425065325,
-2.60079818651808));
#48176=CARTESIAN_POINT('Ctrl Pts',(0.7983385571865,-3.45398822948136,-2.6073115964797));
#48177=CARTESIAN_POINT('Ctrl Pts',(0.608398132847114,-3.49243632959352,
-2.6138250064413));
#48178=CARTESIAN_POINT('Ctrl Pts',(0.416593020999057,-3.51524584577225,
-2.62033841640292));
#48179=CARTESIAN_POINT('Ctrl Pts',(0.276336123570182,-3.53192523424243,
-2.62510132738114));
#48180=CARTESIAN_POINT('Ctrl Pts',(0.135071043364323,-3.54024113541699,
-2.62986423835936));
#48181=CARTESIAN_POINT('Ctrl Pts',(-0.00617846241521518,-3.539994608273,
-2.63462714933759));
#48182=CARTESIAN_POINT('Ctrl Pts',(-0.0580914873315994,-3.53990400286027,
-2.63637764832109));
#48183=CARTESIAN_POINT('Ctrl Pts',(-0.110002393163228,-3.53865692860149,
-2.63812814730459));
#48184=CARTESIAN_POINT('Ctrl Pts',(-0.161860370969655,-3.53626328586113,
-2.6398786462881));
#48185=CARTESIAN_POINT('Ctrl Pts',(-0.35481807755392,-3.52735681026954,
-2.64639205624973));
#48186=CARTESIAN_POINT('Ctrl Pts',(-0.547027243948119,-3.50257873337156,
-2.65290546621137));
#48187=CARTESIAN_POINT('Ctrl Pts',(-0.735963904152669,-3.46243784695285,
-2.659418876173));
#48188=CARTESIAN_POINT('Ctrl Pts',(-0.92490056435722,-3.42229696053415,
-2.66593228613464));
#48189=CARTESIAN_POINT('Ctrl Pts',(-1.11058788540349,-3.36678693880149,
-2.67244569609627));
#48190=CARTESIAN_POINT('Ctrl Pts',(-1.29047199844307,-3.29639980380972,
-2.67895910605791));
#48191=CARTESIAN_POINT('Ctrl Pts',(-1.30621201758925,-3.29024086718272,
-2.67952903519601));
#48192=CARTESIAN_POINT('Ctrl Pts',(-1.32190738964502,-3.28396810707535,
-2.68009896433411));
#48193=CARTESIAN_POINT('Ctrl Pts',(-1.33755638533705,-3.27758187022733,
-2.68066889347221));
#48194=CARTESIAN_POINT('Ctrl Pts',(-1.5007512451651,-3.21098328155419,-2.68661237429584));
#48195=CARTESIAN_POINT('Ctrl Pts',(-1.65890194128621,-3.13204291772606,
-2.69255585511947));
#48196=CARTESIAN_POINT('Ctrl Pts',(-1.81033770201859,-3.04186253180114,
-2.69849933594308));
#48197=CARTESIAN_POINT('Ctrl Pts',(-1.97629486109295,-2.94303461572669,
-2.7050127459047));
#48198=CARTESIAN_POINT('Ctrl Pts',(-2.13420984660948,-2.83069876261338,
-2.7115261558663));
#48199=CARTESIAN_POINT('Ctrl Pts',(-2.28193901730622,-2.70625136015001,
-2.71803956582792));
#48200=CARTESIAN_POINT('Ctrl Pts',(-2.34749402191622,-2.65102766936699,
-2.72092989966008));
#48201=CARTESIAN_POINT('Ctrl Pts',(-2.41104305301027,-2.593418363129,-2.72382023349223));
#48202=CARTESIAN_POINT('Ctrl Pts',(-2.47239011042567,-2.53355227731117,
-2.72671056732439));
#48203=CARTESIAN_POINT('Ctrl Pts',(-2.54928955258278,-2.45850925491567,
-2.73033364345396));
#48204=CARTESIAN_POINT('Ctrl Pts',(-2.62272889170948,-2.37992008874756,
-2.73395671958353));
#48205=CARTESIAN_POINT('Ctrl Pts',(-2.69244525650513,-2.29816470206638,
-2.7375797957131));
#48206=CARTESIAN_POINT('Ctrl Pts',(-2.81777832948228,-2.15118839492212,
-2.74409320567473));
#48207=CARTESIAN_POINT('Ctrl Pts',(-2.93108910381199,-1.9939736040557,-2.75060661563637));
#48208=CARTESIAN_POINT('Ctrl Pts',(-3.03092976256236,-1.82862245583661,
-2.757120025598));
#48209=CARTESIAN_POINT('Ctrl Pts',(-3.11080203430125,-1.69634196001263,
-2.76233073691455));
#48210=CARTESIAN_POINT('Ctrl Pts',(-3.18205838653695,-1.55884051299148,
-2.7675414482311));
#48211=CARTESIAN_POINT('Ctrl Pts',(-3.2439240626505,-1.41723557525111,-2.77275215954765));
#48212=CARTESIAN_POINT('Ctrl Pts',(-3.25939072882222,-1.38183377512727,
-2.77405485819274));
#48213=CARTESIAN_POINT('Ctrl Pts',(-3.27427051474745,-1.34617553341453,
-2.77535755683782));
#48214=CARTESIAN_POINT('Ctrl Pts',(-3.28855875162332,-1.31028157168752,
-2.77666025548291));
#48215=CARTESIAN_POINT('Ctrl Pts',(-3.35999902275125,-1.13081405726206,
-2.78317366544464));
#48216=CARTESIAN_POINT('Ctrl Pts',(-3.41664396289098,-0.9454748130943,-2.78968707540637));
#48217=CARTESIAN_POINT('Ctrl Pts',(-3.45794355355989,-0.756788175000208,
-2.79620048536809));
#48218=CARTESIAN_POINT('Ctrl Pts',(-3.4992431442282,-0.568101536908848,
-2.80271389532973));
#48219=CARTESIAN_POINT('Ctrl Pts',(-3.52520219045535,-0.376044002607322,
-2.80922730529137));
#48220=CARTESIAN_POINT('Ctrl Pts',(-3.53524656047543,-0.183140996775931,
-2.815740715253));
#48221=CARTESIAN_POINT('Ctrl Pts',(-3.5368160129307,-0.152999524933752,
-2.8167584482951));
#48222=CARTESIAN_POINT('Ctrl Pts',(-3.53799685819296,-0.122838037839213,
-2.8177761813372));
#48223=CARTESIAN_POINT('Ctrl Pts',(-3.53878693041333,-0.0926663970097928,
-2.8187939143793));
#48224=CARTESIAN_POINT('Ctrl Pts',(-3.54305325712833,0.0702580470943514,
-2.82428959129884));
#48225=CARTESIAN_POINT('Ctrl Pts',(-3.5359238682156,0.233478412978711,-2.82978526821837));
#48226=CARTESIAN_POINT('Ctrl Pts',(-3.51766563120604,0.39542686488809,-2.83528094513791));
#48227=CARTESIAN_POINT('Ctrl Pts',(-3.4960261890476,0.587366215653757,-2.84179435509964));
#48228=CARTESIAN_POINT('Ctrl Pts',(-3.4587560775586,0.777542371199,-2.84830776506136));
#48229=CARTESIAN_POINT('Ctrl Pts',(-3.40627360153106,0.963435501424819,
-2.85482117502308));
#48230=CARTESIAN_POINT('Ctrl Pts',(-3.3793763475951,1.05870567743577,-2.85815929576337));
#48231=CARTESIAN_POINT('Ctrl Pts',(-3.34848198131686,1.15285246353696,-2.86149741650365));
#48232=CARTESIAN_POINT('Ctrl Pts',(-3.313650756516,1.24551943535272,-2.86483553724394));
#48233=CARTESIAN_POINT('Ctrl Pts',(-3.28051857787996,1.33366616810228,-2.86801082646526));
#48234=CARTESIAN_POINT('Ctrl Pts',(-3.24382428725794,1.42047390410623,-2.87118611568659));
#48235=CARTESIAN_POINT('Ctrl Pts',(-3.20373088991644,1.50567764427224,-2.87436140490792));
#48236=CARTESIAN_POINT('Ctrl Pts',(-3.12148807187998,1.68045444452225,-2.88087481486964));
#48237=CARTESIAN_POINT('Ctrl Pts',(-3.02494376338762,1.84848829715205,-2.88738822483137));
#48238=CARTESIAN_POINT('Ctrl Pts',(-2.91544434228993,2.0076070020078,-2.89390163479326));
#48239=CARTESIAN_POINT('Ctrl Pts',(-2.82031689157503,2.14584112783464,-2.89956014950434));
#48240=CARTESIAN_POINT('Ctrl Pts',(-2.7153993256723,2.27735955487245,-2.90521866421555));
#48241=CARTESIAN_POINT('Ctrl Pts',(-2.601597666831,2.400685231333,-2.91087717892667));
#48242=CARTESIAN_POINT('Ctrl Pts',(-2.58440437448575,2.41931742378652,-2.91173207417739));
#48243=CARTESIAN_POINT('Ctrl Pts',(-2.5670083197053,2.43776262618973,-2.91258696942811));
#48244=CARTESIAN_POINT('Ctrl Pts',(-2.54941430867889,2.4560172922504,-2.91344186467883));
#48245=CARTESIAN_POINT('Ctrl Pts',(-2.41536629918196,2.59509880389615,-2.91995527464064));
#48246=CARTESIAN_POINT('Ctrl Pts',(-2.26984684389257,2.72310064051428,-2.92646868460227));
#48247=CARTESIAN_POINT('Ctrl Pts',(-2.11495442977927,2.83849845023986,-2.93298209456391));
#48248=CARTESIAN_POINT('Ctrl Pts',(-1.96006201566371,2.95389625996712,-2.93949550452564));
#48249=CARTESIAN_POINT('Ctrl Pts',(-1.79577783391285,3.05670494108783,-2.94600891448736));
#48250=CARTESIAN_POINT('Ctrl Pts',(-1.62417584367481,3.14538952674968,-2.95252232444909));
#48251=CARTESIAN_POINT('Ctrl Pts',(-1.5855649121518,3.16534380851171,-2.95398786005078));
#48252=CARTESIAN_POINT('Ctrl Pts',(-1.54658437024401,3.18458250627967,-2.95545339565246));
#48253=CARTESIAN_POINT('Ctrl Pts',(-1.50725869214041,3.20308776572967,-2.95691893125415));
#48254=CARTESIAN_POINT('Ctrl Pts',(-1.37180576833643,3.26682707345756,-2.9619668056141));
#48255=CARTESIAN_POINT('Ctrl Pts',(-1.23225792299338,3.32186406534164,-2.96701467997405));
#48256=CARTESIAN_POINT('Ctrl Pts',(-1.08981621794126,3.36789750679959,-2.972062554334));
#48257=CARTESIAN_POINT('Ctrl Pts',(-0.90601980097821,3.42729571182215,-2.97857596429564));
#48258=CARTESIAN_POINT('Ctrl Pts',(-0.717386036659192,3.47171455680863,
-2.98508937425727));
#48259=CARTESIAN_POINT('Ctrl Pts',(-0.526388358542247,3.50052703129853,
-2.99160278421891));
#48260=CARTESIAN_POINT('Ctrl Pts',(-0.415371292863036,3.51727423160149,
-2.99538869234426));
#48261=CARTESIAN_POINT('Ctrl Pts',(-0.303551189065533,3.52874803372401,
-2.99917460046961));
#48262=CARTESIAN_POINT('Ctrl Pts',(-0.191438997966164,3.5348198129545,-3.00296050859496));
#48263=CARTESIAN_POINT('Ctrl Pts',(-0.110669418520737,3.53919413701438,
-3.00568801043134));
#48264=CARTESIAN_POINT('Ctrl Pts',(-0.0297482761444177,3.54076478310675,
-3.00841551226771));
#48265=CARTESIAN_POINT('Ctrl Pts',(0.0511292772991568,3.53955874091815,
-3.01114301410408));
#48266=CARTESIAN_POINT('Ctrl Pts',(0.244268895115812,3.53667865222285,-3.0176564240657));
#48267=CARTESIAN_POINT('Ctrl Pts',(0.437158914978994,3.51796689039577,-3.0241698340273));
#48268=CARTESIAN_POINT('Ctrl Pts',(0.627264950562928,3.48378569015157,-3.03068324398892));
#48269=CARTESIAN_POINT('Ctrl Pts',(0.805489255928714,3.45174083344104,-3.03678956229916));
#48270=CARTESIAN_POINT('Ctrl Pts',(0.981286782970914,3.40609307546753,-3.0428958806094));
#48271=CARTESIAN_POINT('Ctrl Pts',(1.15251126677808,3.3471357576215,-3.04900219891965));
#48272=CARTESIAN_POINT('Ctrl Pts',(1.16392633791351,3.34320523342191,-3.04940929057113));
#48273=CARTESIAN_POINT('Ctrl Pts',(1.1753210843407,3.33921555889236,-3.04981638222261));
#48274=CARTESIAN_POINT('Ctrl Pts',(1.18669494970798,3.33516705334005,-3.05022347387409));
#48275=CARTESIAN_POINT('Ctrl Pts',(1.36867521807276,3.27039152601533,-3.05673688383573));
#48276=CARTESIAN_POINT('Ctrl Pts',(1.54528068641558,3.19056603871398,-3.06325029379737));
#48277=CARTESIAN_POINT('Ctrl Pts',(1.7142617758279,3.09700442209031,-3.069763703759));
#48278=CARTESIAN_POINT('Ctrl Pts',(1.88324286524021,3.00344280546664,-3.07627711372064));
#48279=CARTESIAN_POINT('Ctrl Pts',(2.04462139391706,2.89613498241052,-3.08279052368227));
#48280=CARTESIAN_POINT('Ctrl Pts',(2.19616581212668,2.77635948507303,-3.08930393364391));
#48281=CARTESIAN_POINT('Ctrl Pts',(2.24068245442155,2.74117506169632,-3.09121726799701));
#48282=CARTESIAN_POINT('Ctrl Pts',(2.28434948110076,2.70491536505777,-3.09313060235012));
#48283=CARTESIAN_POINT('Ctrl Pts',(2.32710837011083,2.667614408748,-3.09504393670323));
#48284=CARTESIAN_POINT('Ctrl Pts',(2.42991012144495,2.57793472520482,-3.09964401231185));
#48285=CARTESIAN_POINT('Ctrl Pts',(2.52746203568147,2.4822357996935,-3.10424408792047));
#48286=CARTESIAN_POINT('Ctrl Pts',(2.61918727517748,2.38126086742591,-3.10884416352909));
#48287=CARTESIAN_POINT('Ctrl Pts',(2.74906429014366,2.2382868848952,-3.11535757349073));
#48288=CARTESIAN_POINT('Ctrl Pts',(2.8672760376804,2.08472396627836,-3.12187098345237));
#48289=CARTESIAN_POINT('Ctrl Pts',(2.97225682514692,1.92258536488255,-3.128384393414));
#48290=CARTESIAN_POINT('Ctrl Pts',(3.04049404589932,1.81719572356882,-3.13261809182805));
#48291=CARTESIAN_POINT('Ctrl Pts',(3.10314345866287,1.7081759162302,-3.13685179024211));
#48292=CARTESIAN_POINT('Ctrl Pts',(3.15975379732033,1.59610649404043,-3.14108548865616));
#48293=CARTESIAN_POINT('Ctrl Pts',(3.19023665890577,1.53576068503122,-3.14336520020374));
#48294=CARTESIAN_POINT('Ctrl Pts',(3.21896862084255,1.4745307323558,-3.14564491175132));
#48295=CARTESIAN_POINT('Ctrl Pts',(3.24591833613534,1.41252706412558,-3.14792462329891));
#48296=CARTESIAN_POINT('Ctrl Pts',(3.32291691266137,1.23537512981941,-3.15443803326064));
#48297=CARTESIAN_POINT('Ctrl Pts',(3.38536604105095,1.05191544335807,-3.16095144322237));
#48298=CARTESIAN_POINT('Ctrl Pts',(3.43257863439251,0.864620338177983,-3.16746485318408));
#48299=CARTESIAN_POINT('Ctrl Pts',(3.47979122773339,0.677325233000615,-3.1739782631457));
#48300=CARTESIAN_POINT('Ctrl Pts',(3.51177061081401,0.486170850953884,-3.1804916731073));
#48301=CARTESIAN_POINT('Ctrl Pts',(3.52779770972739,0.293671846368205,-3.18700508306892));
#48302=CARTESIAN_POINT('Ctrl Pts',(3.543824808641,0.101172841779728,-3.19351849303064));
#48303=CARTESIAN_POINT('Ctrl Pts',(3.54389063706576,-0.0926387220615211,
-3.20003190299237));
#48304=CARTESIAN_POINT('Ctrl Pts',(3.52829370107048,-0.285162093399606,
-3.20654531295409));
#48305=CARTESIAN_POINT('Ctrl Pts',(3.51269676507543,-0.477685464734901,
-3.21305872291573));
#48306=CARTESIAN_POINT('Ctrl Pts',(3.48143795907197,-0.668944729192226,
-3.21957213287737));
#48307=CARTESIAN_POINT('Ctrl Pts',(3.43479147403392,-0.856389724647796,
-3.226085542839));
#48308=CARTESIAN_POINT('Ctrl Pts',(3.41788200033906,-0.924339029237458,
-3.22844667110665));
#48309=CARTESIAN_POINT('Ctrl Pts',(3.39895032352517,-0.991786185528747,
-3.23080779937431));
#48310=CARTESIAN_POINT('Ctrl Pts',(3.37801076294783,-1.05860440458689,-3.23316892764197));
#48311=CARTESIAN_POINT('Ctrl Pts',(3.34118643821444,-1.17611096770774,-3.23732120933597));
#48312=CARTESIAN_POINT('Ctrl Pts',(3.29815197932222,-1.29167222505157,-3.24147349102998));
#48313=CARTESIAN_POINT('Ctrl Pts',(3.24923804098248,-1.40467798595002,-3.24562577272407));
#48314=CARTESIAN_POINT('Ctrl Pts',(3.17250997753937,-1.58194265704298,-3.25213918268597));
#48315=CARTESIAN_POINT('Ctrl Pts',(3.08131256433664,-1.75293573710959,-3.25865259264803));
#48316=CARTESIAN_POINT('Ctrl Pts',(2.97686209402291,-1.91541538362651,-3.26516600260991));
#48317=CARTESIAN_POINT('Ctrl Pts',(2.90178864237807,-2.03219712572322,-3.26984749582241));
#48318=CARTESIAN_POINT('Ctrl Pts',(2.81986112148131,-2.14458818654423,-3.27452898903482));
#48319=CARTESIAN_POINT('Ctrl Pts',(2.73155102519233,-2.2517168997835,-3.27921048224721));
#48320=CARTESIAN_POINT('Ctrl Pts',(2.6969943704714,-2.29363747409692,-3.28104239899645));
#48321=CARTESIAN_POINT('Ctrl Pts',(2.66146049390567,-2.3347523204531,-3.28287431574568));
#48322=CARTESIAN_POINT('Ctrl Pts',(2.62499516111465,-2.37502361902704,-3.28470623249492));
#48323=CARTESIAN_POINT('Ctrl Pts',(2.4953420740096,-2.51820887971737,-3.29121964245664));
#48324=CARTESIAN_POINT('Ctrl Pts',(2.35392512391005,-2.65072077167277,-3.29773305241837));
#48325=CARTESIAN_POINT('Ctrl Pts',(2.20273828215037,-2.77093269463369,-3.3042464623801));
#48326=CARTESIAN_POINT('Ctrl Pts',(2.05155144039287,-2.89114461759288,-3.31075987234173));
#48327=CARTESIAN_POINT('Ctrl Pts',(1.89057497031891,-2.9990702680108,-3.31727328230337));
#48328=CARTESIAN_POINT('Ctrl Pts',(1.7218118521876,-3.09304726818777,-3.323786692265));
#48329=CARTESIAN_POINT('Ctrl Pts',(1.70915449898499,-3.10009560965795,-3.32427520261816));
#48330=CARTESIAN_POINT('Ctrl Pts',(1.69645349524291,-3.10706540362333,-3.32476371297131));
#48331=CARTESIAN_POINT('Ctrl Pts',(1.68370970010857,-3.11395594794783,-3.32525222332447));
#48332=CARTESIAN_POINT('Ctrl Pts',(1.52653782888907,-3.19893846169562,-3.33127712293295));
#48333=CARTESIAN_POINT('Ctrl Pts',(1.36285678345318,-3.2718654745696,-3.33730202254143));
#48334=CARTESIAN_POINT('Ctrl Pts',(1.19465624061227,-3.33212144593867,-3.34332692214991));
#48335=CARTESIAN_POINT('Ctrl Pts',(1.01281767690137,-3.39726308640959,-3.34984033211164));
#48336=CARTESIAN_POINT('Ctrl Pts',(0.825675827052175,-3.44760704052864,
-3.35635374207337));
#48337=CARTESIAN_POINT('Ctrl Pts',(0.635671099317594,-3.48238259226642,
-3.3628671520351));
#48338=CARTESIAN_POINT('Ctrl Pts',(0.553731273711291,-3.49737960143946,
-3.36567606991167));
#48339=CARTESIAN_POINT('Ctrl Pts',(0.471258885802527,-3.50948064073937,
-3.36848498778823));
#48340=CARTESIAN_POINT('Ctrl Pts',(0.38845946126229,-3.51862178231117,-3.37129390566481));
#48341=CARTESIAN_POINT('Ctrl Pts',(0.279260892156459,-3.53067741657646,
-3.37499839774987));
#48342=CARTESIAN_POINT('Ctrl Pts',(0.169493539234521,-3.53758465049955,
-3.37870288983494));
#48343=CARTESIAN_POINT('Ctrl Pts',(0.059649471939911,-3.53938415619341,
-3.38240738192));
#48344=CARTESIAN_POINT('Ctrl Pts',(-0.133483466588335,-3.54254813064478,
-3.38892079188164));
#48345=CARTESIAN_POINT('Ctrl Pts',(-0.326865118477281,-3.52992630187154,
-3.39543420184327));
#48346=CARTESIAN_POINT('Ctrl Pts',(-0.517952514192366,-3.50173373138306,
-3.40194761180491));
#48347=CARTESIAN_POINT('Ctrl Pts',(-0.668433322988736,-3.47953215815382,
-3.40707690458417));
#48348=CARTESIAN_POINT('Ctrl Pts',(-0.817504437674782,-3.44766956351041,
-3.41220619736343));
#48349=CARTESIAN_POINT('Ctrl Pts',(-0.963872074523706,-3.4062516970935,
-3.41733549014268));
#48350=CARTESIAN_POINT('Ctrl Pts',(-1.00336874001705,-3.39507526731343,
-3.41871960732515));
#48351=CARTESIAN_POINT('Ctrl Pts',(-1.04266855713235,-3.38320312817922,
-3.42010372450761));
#48352=CARTESIAN_POINT('Ctrl Pts',(-1.0817487466423,-3.37064673995017,-3.42148784169008));
#48353=CARTESIAN_POINT('Ctrl Pts',(-1.26565318687387,-3.31155860405448,
-3.4280012516517));
#48354=CARTESIAN_POINT('Ctrl Pts',(-1.4446743658271,-3.23732575217221,-3.4345146616133));
#48355=CARTESIAN_POINT('Ctrl Pts',(-1.61651402611654,-3.14912462305492,
-3.44102807157492));
#48356=CARTESIAN_POINT('Ctrl Pts',(-1.78835368640846,-3.06092349393635,
-3.44754148153664));
#48357=CARTESIAN_POINT('Ctrl Pts',(-1.95303292882817,-2.95874267186129,
-3.45405489149837));
#48358=CARTESIAN_POINT('Ctrl Pts',(-2.10823418017326,-2.84374236629767,
-3.4605683014601));
#48359=CARTESIAN_POINT('Ctrl Pts',(-2.13054463355673,-2.8272108697142,-3.46150461562032));
#48360=CARTESIAN_POINT('Ctrl Pts',(-2.15265877543496,-2.81041477835907,
-3.46244092978054));
#48361=CARTESIAN_POINT('Ctrl Pts',(-2.17456960835048,-2.79335766031483,
-3.46337724394076));
#48362=CARTESIAN_POINT('Ctrl Pts',(-2.30508009238466,-2.69175802050364,
-3.46895433974217));
#48363=CARTESIAN_POINT('Ctrl Pts',(-2.42837651672354,-2.58089661856788,
-3.47453143554359));
#48364=CARTESIAN_POINT('Ctrl Pts',(-2.5433709048767,-2.46202800977271,-3.480108531345));
#48365=CARTESIAN_POINT('Ctrl Pts',(-2.67767119664131,-2.3232030714498,-3.48662194130664));
#48366=CARTESIAN_POINT('Ctrl Pts',(-2.80066707596171,-2.17344287527037,
-3.49313535126827));
#48367=CARTESIAN_POINT('Ctrl Pts',(-2.91067619386607,-2.01467029405205,
-3.49964876122991));
#48368=CARTESIAN_POINT('Ctrl Pts',(-2.96568075281904,-1.93528400344175,
-3.50290546621077));
#48369=CARTESIAN_POINT('Ctrl Pts',(-3.01743874035383,-1.85364279298029,
-3.50616217119164));
#48370=CARTESIAN_POINT('Ctrl Pts',(-3.06572992939683,-1.76999999999985,
-3.5094188761725));
#48371=CARTESIAN_POINT('Ctrl Pts',(-3.11402111843984,-1.6863572070194,-3.51267558115337));
#48372=CARTESIAN_POINT('Ctrl Pts',(-3.15884548692774,-1.60071286973475,
-3.51593228613423));
#48373=CARTESIAN_POINT('Ctrl Pts',(-3.20009375183195,-1.51338437905234,
-3.51918899111509));
#48374=CARTESIAN_POINT('Ctrl Pts',(-3.28259028163917,-1.33872739769007,
-3.52570240107673));
#48375=CARTESIAN_POINT('Ctrl Pts',(-3.350788476346,-1.15732974354807,-3.53221581103837));
#48376=CARTESIAN_POINT('Ctrl Pts',(-3.40386425373005,-0.971609809982892,
-3.538729221));
#48377=CARTESIAN_POINT('Ctrl Pts',(-3.44931029458254,-0.812587444152017,
-3.54430631680142));
#48378=CARTESIAN_POINT('Ctrl Pts',(-3.48367087278858,-0.650378907510944,
-3.54988341260283));
#48379=CARTESIAN_POINT('Ctrl Pts',(-3.50640349986333,-0.486553692971483,
-3.55546050840425));
#48380=CARTESIAN_POINT('Ctrl Pts',(-3.51021998094721,-0.45904979602653,
-3.55639682256447));
#48381=CARTESIAN_POINT('Ctrl Pts',(-3.51370875180592,-0.431500341699595,
-3.55733313672469));
#48382=CARTESIAN_POINT('Ctrl Pts',(-3.51687022111804,-0.4039131740079,-3.55826945088491));
#48383=CARTESIAN_POINT('Ctrl Pts',(-3.53886278150659,-0.21200479486206,
-3.56478286084664));
#48384=CARTESIAN_POINT('Ctrl Pts',(-3.54501434799336,-0.018297976412778,
-3.57129627080837));
#48385=CARTESIAN_POINT('Ctrl Pts',(-3.53547893630661,0.174620099336988,
-3.57780968077025));
#48386=CARTESIAN_POINT('Ctrl Pts',(-3.52594352461999,0.367538175083959,
-3.58432309073203));
#48387=CARTESIAN_POINT('Ctrl Pts',(-3.50072047066892,0.559691489813732,
-3.59083650069397));
#48388=CARTESIAN_POINT('Ctrl Pts',(-3.45994007730116,0.748501474870884,
-3.59734991065576));
#48389=CARTESIAN_POINT('Ctrl Pts',(-3.45127413373233,0.788624105885788,
-3.59873402783826));
#48390=CARTESIAN_POINT('Ctrl Pts',(-3.44190579926218,0.828594815438887,
-3.60011814502075));
#48391=CARTESIAN_POINT('Ctrl Pts',(-3.43183653862866,0.868388146010993,
-3.60150226220324));
#48392=CARTESIAN_POINT('Ctrl Pts',(-3.39452164469186,1.01585517102254,-3.60663155498258));
#48393=CARTESIAN_POINT('Ctrl Pts',(-3.34757990374054,1.16088584063295,-3.61176084776184));
#48394=CARTESIAN_POINT('Ctrl Pts',(-3.2915666257629,1.30230683044729,-3.61689014054109));
#48395=CARTESIAN_POINT('Ctrl Pts',(-3.22043841014641,1.48188965472389,-3.62340355050273));
#48396=CARTESIAN_POINT('Ctrl Pts',(-3.13467840856183,1.65567399227211,-3.62991696046437));
#48397=CARTESIAN_POINT('Ctrl Pts',(-3.03537185704593,1.82135003611944,-3.636430370426));
#48398=CARTESIAN_POINT('Ctrl Pts',(-2.97889140575354,1.91557803600459,-3.64013486251106));
#48399=CARTESIAN_POINT('Ctrl Pts',(-2.91802588924534,2.00718573517956,-3.64383935459613));
#48400=CARTESIAN_POINT('Ctrl Pts',(-2.85298611916,2.09572665294942,-3.64754384668119));
#48401=CARTESIAN_POINT('Ctrl Pts',(-2.80366994606909,2.16286248723415,-3.65035276455776));
#48402=CARTESIAN_POINT('Ctrl Pts',(-2.75195394466873,2.228235150624,-3.65316168243433));
#48403=CARTESIAN_POINT('Ctrl Pts',(-2.6979962409409,2.29169861659425,-3.65597060031091));
#48404=CARTESIAN_POINT('Ctrl Pts',(-2.57287736583807,2.43885976178261,-3.66248401027264));
#48405=CARTESIAN_POINT('Ctrl Pts',(-2.43570729771941,2.57575738080365,-3.66899742023437));
#48406=CARTESIAN_POINT('Ctrl Pts',(-2.2883737003719,2.70066337612947,-3.67551083019609));
#48407=CARTESIAN_POINT('Ctrl Pts',(-2.15209022701611,2.81620133347544,-3.68153572980457));
#48408=CARTESIAN_POINT('Ctrl Pts',(-2.00709305852713,2.92148977050388,-3.68756062941305));
#48409=CARTESIAN_POINT('Ctrl Pts',(-1.85491010713434,3.01511334686633,-3.69358552902153));
#48410=CARTESIAN_POINT('Ctrl Pts',(-1.84257082313618,3.02270452503107,-3.69407403937469));
#48411=CARTESIAN_POINT('Ctrl Pts',(-1.83018430263193,3.03021901994261,-3.69456254972784));
#48412=CARTESIAN_POINT('Ctrl Pts',(-1.81775158326284,3.03765643862568,-3.695051060081));
#48413=CARTESIAN_POINT('Ctrl Pts',(-1.65198355467242,3.13682108606072,-3.70156447004264));
#48414=CARTESIAN_POINT('Ctrl Pts',(-1.47802896465355,3.22226797334726,-3.70807788000427));
#48415=CARTESIAN_POINT('Ctrl Pts',(-1.2983289646543,3.29309365754754,-3.71459128996591));
#48416=CARTESIAN_POINT('Ctrl Pts',(-1.11862896465245,3.36391934174885,-3.72110469992764));
#48417=CARTESIAN_POINT('Ctrl Pts',(-0.933161824865596,3.42013406708304,
-3.72761810988937));
#48418=CARTESIAN_POINT('Ctrl Pts',(-0.744333208107735,3.46082430384987,
-3.73413151985108));
#48419=CARTESIAN_POINT('Ctrl Pts',(-0.691224574103849,3.47226855911735,
-3.73596343660032));
#48420=CARTESIAN_POINT('Ctrl Pts',(-0.637851134403885,3.48248437574009,
-3.73779535334955));
#48421=CARTESIAN_POINT('Ctrl Pts',(-0.58426852474683,3.4914510294415,-3.73962727009879));
#48422=CARTESIAN_POINT('Ctrl Pts',(-0.447337289462379,3.51436545961875,
-3.74430876331116));
#48423=CARTESIAN_POINT('Ctrl Pts',(-0.309040015184776,3.5291212435739,-3.74899025652354));
#48424=CARTESIAN_POINT('Ctrl Pts',(-0.17036733400844,3.53574588879975,-3.75367174973592));
#48425=CARTESIAN_POINT('Ctrl Pts',(0.0225694026298665,3.5449628262702,-3.76018515969764));
#48426=CARTESIAN_POINT('Ctrl Pts',(0.216252460440131,3.5384455628299,-3.76669856965937));
#48427=CARTESIAN_POINT('Ctrl Pts',(0.408132200521637,3.51626167940836,-3.7732119796211));
#48428=CARTESIAN_POINT('Ctrl Pts',(0.530455029403651,3.50211951216048,-3.77736426131508));
#48429=CARTESIAN_POINT('Ctrl Pts',(0.652051243402925,3.48160781812733,-3.78151654300907));
#48430=CARTESIAN_POINT('Ctrl Pts',(0.772227074543825,3.45474533726317,-3.78566882470305));
#48431=CARTESIAN_POINT('Ctrl Pts',(0.840563129972376,3.43947041913817,-3.7880299529707));
#48432=CARTESIAN_POINT('Ctrl Pts',(0.908439919140494,3.4221421540496,-3.79039108123835));
#48433=CARTESIAN_POINT('Ctrl Pts',(0.975740479931958,3.40281153553916,-3.792752209506));
#48434=CARTESIAN_POINT('Ctrl Pts',(1.16139585032783,3.34948607885153,-3.79926561946764));
#48435=CARTESIAN_POINT('Ctrl Pts',(1.34266063505881,3.28092736671375,-3.80577902942927));
#48436=CARTESIAN_POINT('Ctrl Pts',(1.51718923345482,3.19817302383904,-3.81229243939091));
#48437=CARTESIAN_POINT('Ctrl Pts',(1.69171783185335,3.11541868096314,-3.81880584935264));
#48438=CARTESIAN_POINT('Ctrl Pts',(1.85953065547441,3.01845588995455,-3.82531925931437));
#48439=CARTESIAN_POINT('Ctrl Pts',(2.0182261341945,2.90832651285219,-3.83183266927608));
#48440=CARTESIAN_POINT('Ctrl Pts',(2.1769216129123,2.79819713575142,-3.8383460792377));
#48441=CARTESIAN_POINT('Ctrl Pts',(2.32647647226952,2.67492498658273,-3.8448594891993));
#48442=CARTESIAN_POINT('Ctrl Pts',(2.4650724946873,2.54039012878225,-3.85137289916092));
#48443=CARTESIAN_POINT('Ctrl Pts',(2.60366851710708,2.40585527097982,-3.85788630912264));
#48444=CARTESIAN_POINT('Ctrl Pts',(2.73132470195812,2.26004289611969,-3.86439971908436));
#48445=CARTESIAN_POINT('Ctrl Pts',(2.84624348913382,2.10478420563982,-3.87091312904609));
#48446=CARTESIAN_POINT('Ctrl Pts',(2.88646538330249,2.05044323345657,-3.87319284059367));
#48447=CARTESIAN_POINT('Ctrl Pts',(2.92512609682342,1.99494564818121,-3.87547255214125));
#48448=CARTESIAN_POINT('Ctrl Pts',(2.96214566964451,1.93837381116374,-3.87775226368882));
#48449=CARTESIAN_POINT('Ctrl Pts',(3.03089546691971,1.83331310867443,-3.88198596210288));
#48450=CARTESIAN_POINT('Ctrl Pts',(3.09398468320899,1.72454722201944,-3.88621966051694));
#48451=CARTESIAN_POINT('Ctrl Pts',(3.1511361795063,1.61275723470709,-3.890453358931));
#48452=CARTESIAN_POINT('Ctrl Pts',(3.23906193351585,1.4407719051538,-3.89696676889264));
#48453=CARTESIAN_POINT('Ctrl Pts',(3.31294544834883,1.26161606945278,-3.90348017885427));
#48454=CARTESIAN_POINT('Ctrl Pts',(3.37182604181743,1.07765228385916,-3.90999358881607));
#48455=CARTESIAN_POINT('Ctrl Pts',(3.41341027855843,0.947728430153869,-3.91459366442481));
#48456=CARTESIAN_POINT('Ctrl Pts',(3.44751202204771,0.815396531481927,-3.91919374003363));
#48457=CARTESIAN_POINT('Ctrl Pts',(3.47377603053233,0.681527761501758,-3.92379381564241));
#48458=CARTESIAN_POINT('Ctrl Pts',(3.48470016177703,0.625846999226429,-3.92570714999559));
#48459=CARTESIAN_POINT('Ctrl Pts',(3.49426846685995,0.569900396495106,-3.92762048434877));
#48460=CARTESIAN_POINT('Ctrl Pts',(3.50248075017427,0.513755641688056,-3.92953381870193));
#48461=CARTESIAN_POINT('Ctrl Pts',(3.53043716451462,0.322626577048128,-3.93604722866373));
#48462=CARTESIAN_POINT('Ctrl Pts',(3.54267920096763,0.129214760060477,-3.94256063862537));
#48463=CARTESIAN_POINT('Ctrl Pts',(3.53921539307674,-0.063907964441538,
-3.949074048587));
#48464=CARTESIAN_POINT('Ctrl Pts',(3.53575158518584,-0.257030688943553,
-3.95558745854864));
#48465=CARTESIAN_POINT('Ctrl Pts',(3.51657975088695,-0.449888254626207,
-3.96210086851027));
#48466=CARTESIAN_POINT('Ctrl Pts',(3.48168686891133,-0.639875553680029,
-3.96861427847191));
#48467=CARTESIAN_POINT('Ctrl Pts',(3.47950604488335,-0.651749862803495,
-3.96902137012339));
#48468=CARTESIAN_POINT('Ctrl Pts',(3.47726383116518,-0.663612839943919,
-3.96942846177487));
#48469=CARTESIAN_POINT('Ctrl Pts',(3.4749602294045,-0.675463843633017,-3.96983555342635));
#48470=CARTESIAN_POINT('Ctrl Pts',(3.4404065224946,-0.853227255282967,-3.9759418717366));
#48471=CARTESIAN_POINT('Ctrl Pts',(3.39203987700435,-1.02829625861096,-3.98204819004685));
#48472=CARTESIAN_POINT('Ctrl Pts',(3.33067938429338,-1.19866546298495,-3.98815450835708));
#48473=CARTESIAN_POINT('Ctrl Pts',(3.26522815424471,-1.38039271933565,-3.9946679183187));
#48474=CARTESIAN_POINT('Ctrl Pts',(3.18498800540492,-1.55679625758723,-4.0011813282803));
#48475=CARTESIAN_POINT('Ctrl Pts',(3.09091242647188,-1.72550011744132,-4.00769473824192));
#48476=CARTESIAN_POINT('Ctrl Pts',(3.05151811292345,-1.79614515441368,-4.01042224007829));
#48477=CARTESIAN_POINT('Ctrl Pts',(3.00969732231895,-1.86543959636863,-4.01314974191466));
#48478=CARTESIAN_POINT('Ctrl Pts',(2.965524256836,-1.9332009419914,-4.01587724375104));
#48479=CARTESIAN_POINT('Ctrl Pts',(2.90420984622655,-2.02725705794212,-4.01966315187639));
#48480=CARTESIAN_POINT('Ctrl Pts',(2.83836319021171,-2.11835920742328,-4.02344906000174));
#48481=CARTESIAN_POINT('Ctrl Pts',(2.76835115646748,-2.20612920640356,-4.02723496812709));
#48482=CARTESIAN_POINT('Ctrl Pts',(2.64789998255489,-2.35713181047166,-4.03374837808873));
#48483=CARTESIAN_POINT('Ctrl Pts',(2.5151152522304,-2.49828401989007,-4.04026178805037));
#48484=CARTESIAN_POINT('Ctrl Pts',(2.37177668926012,-2.62775728359333,-4.046775198012));
#48485=CARTESIAN_POINT('Ctrl Pts',(2.26068970700779,-2.7280986979979,-4.05182307237195));
#48486=CARTESIAN_POINT('Ctrl Pts',(2.14325235121661,-2.82143218116641,-4.05687094673191));
#48487=CARTESIAN_POINT('Ctrl Pts',(2.02032602960248,-2.90686820033367,-4.06191882109186));
#48488=CARTESIAN_POINT('Ctrl Pts',(1.98463716576339,-2.93167260686741,-4.06338435669354));
#48489=CARTESIAN_POINT('Ctrl Pts',(1.94848569380674,-2.95581139752882,-4.06484989229522));
#48490=CARTESIAN_POINT('Ctrl Pts',(1.91189931312508,-2.97927230421048,-4.06631542789691));
#48491=CARTESIAN_POINT('Ctrl Pts',(1.7492952138987,-3.08354169426571,-4.07282883785864));
#48492=CARTESIAN_POINT('Ctrl Pts',(1.57811819344313,-3.17441162854151,-4.07934224782037));
#48493=CARTESIAN_POINT('Ctrl Pts',(1.40073455162058,-3.25085348915537,-4.0858556577821));
#48494=CARTESIAN_POINT('Ctrl Pts',(1.22335090980063,-3.32729534976811,-4.09236906774373));
#48495=CARTESIAN_POINT('Ctrl Pts',(1.03973833991381,-3.38931797648445,-4.09888247770537));
#48496=CARTESIAN_POINT('Ctrl Pts',(0.852266212883417,-3.43586620221265,
-4.105395887667));
#48497=CARTESIAN_POINT('Ctrl Pts',(0.827660202824008,-3.44197572968566,
-4.1062507829177));
#48498=CARTESIAN_POINT('Ctrl Pts',(0.802988161574587,-3.44781855384957,
-4.1071056781684));
#48499=CARTESIAN_POINT('Ctrl Pts',(0.778255563408939,-3.4533922855685,-4.1079605734191));
#48500=CARTESIAN_POINT('Ctrl Pts',(0.614551565234618,-3.49028457488758,
-4.11361908813004));
#48501=CARTESIAN_POINT('Ctrl Pts',(0.448194483402658,-3.51538663874368,
-4.11927760284097));
#48502=CARTESIAN_POINT('Ctrl Pts',(0.280916493409238,-3.52865236474662,
-4.12493611755191));
#48503=CARTESIAN_POINT('Ctrl Pts',(0.0883659422379453,-3.54392229268905,
-4.13144952751364));
#48504=CARTESIAN_POINT('Ctrl Pts',(-0.105427797081422,-3.54351519011934,
-4.13796293747536));
#48505=CARTESIAN_POINT('Ctrl Pts',(-0.297910355108321,-3.52735115969274,
-4.14447634743708));
#48506=CARTESIAN_POINT('Ctrl Pts',(-0.39174565726025,-3.51947119023151,
-4.14765163665841));
#48507=CARTESIAN_POINT('Ctrl Pts',(-0.485270507195668,-3.50784551008206,
-4.15082692587973));
#48508=CARTESIAN_POINT('Ctrl Pts',(-0.578173906335351,-3.49246545208883,
-4.15400221510106));
#48509=CARTESIAN_POINT('Ctrl Pts',(-0.675841470420018,-3.47629669170343,
-4.15734033584135));
#48510=CARTESIAN_POINT('Ctrl Pts',(-0.772822162007415,-3.45597860468362,
-4.16067845658163));
#48511=CARTESIAN_POINT('Ctrl Pts',(-0.868777181623859,-3.43163722187875,
-4.16401657732192));
#48512=CARTESIAN_POINT('Ctrl Pts',(-1.05600659280207,-3.38414181425924,
-4.17052998728364));
#48513=CARTESIAN_POINT('Ctrl Pts',(-1.23933903044262,-3.32133059983808,
-4.17704339724537));
#48514=CARTESIAN_POINT('Ctrl Pts',(-1.41638310527089,-3.24410123108816,
-4.1835568072071));
#48515=CARTESIAN_POINT('Ctrl Pts',(-1.56576369723281,-3.17893910221207,
-4.18905248412663));
#48516=CARTESIAN_POINT('Ctrl Pts',(-1.71068137496023,-3.10350315118168,
-4.19454816104616));
#48517=CARTESIAN_POINT('Ctrl Pts',(-1.8496449190945,-3.0183461818135,-4.20004383796569));
#48518=CARTESIAN_POINT('Ctrl Pts',(-1.87537929041651,-3.00257613878509,
-4.2010615710078));
#48519=CARTESIAN_POINT('Ctrl Pts',(-1.90090948182522,-2.98647275324273,
-4.2020793040499));
#48520=CARTESIAN_POINT('Ctrl Pts',(-1.9262280359204,-2.97004283162531,-4.203097037092));
#48521=CARTESIAN_POINT('Ctrl Pts',(-2.08826475442685,-2.86489264910712,
-4.20961044705364));
#48522=CARTESIAN_POINT('Ctrl Pts',(-2.24161193500656,-2.74638268846562,
-4.21612385701527));
#48523=CARTESIAN_POINT('Ctrl Pts',(-2.38436956161414,-2.61627287473533,
-4.22263726697691));
#48524=CARTESIAN_POINT('Ctrl Pts',(-2.52712718822379,-2.48616306100314,
-4.22915067693864));
#48525=CARTESIAN_POINT('Ctrl Pts',(-2.65931321192137,-2.34443748176244,
-4.23566408690037));
#48526=CARTESIAN_POINT('Ctrl Pts',(-2.77901650300382,-2.19283463489973,
-4.2421774968621));
#48527=CARTESIAN_POINT('Ctrl Pts',(-2.80295746726397,-2.16251367792641,
-4.24348019550718));
#48528=CARTESIAN_POINT('Ctrl Pts',(-2.8263985174789,-2.13179828445587,-4.24478289415227));
#48529=CARTESIAN_POINT('Ctrl Pts',(-2.84932404264,-2.10070285857735,-4.24608559279736));
#48530=CARTESIAN_POINT('Ctrl Pts',(-2.94102467796757,-1.97632314257066,
-4.25129630411391));
#48531=CARTESIAN_POINT('Ctrl Pts',(-3.02447624802702,-1.84586260784311,
-4.25650701543049));
#48532=CARTESIAN_POINT('Ctrl Pts',(-3.09909838196629,-1.71055094354732,
-4.26171772674717));
#48533=CARTESIAN_POINT('Ctrl Pts',(-3.19237634749372,-1.54141082262935,
-4.26823113670897));
#48534=CARTESIAN_POINT('Ctrl Pts',(-3.27187296306989,-1.36467341810391,
-4.27474454667094));
#48535=CARTESIAN_POINT('Ctrl Pts',(-3.33649164232266,-1.18264363939907,
-4.28125795663274));
#48536=CARTESIAN_POINT('Ctrl Pts',(-3.37243570168691,-1.08138980308597,
-4.2848810327624));
#48537=CARTESIAN_POINT('Ctrl Pts',(-3.40377624648734,-0.978494886681129,
-4.288504108892));
#48538=CARTESIAN_POINT('Ctrl Pts',(-3.43031568918,-0.874376505038574,-4.29212718502158));
#48539=CARTESIAN_POINT('Ctrl Pts',(-3.45148771161571,-0.791315351960366,
-4.29501751885376));
#48540=CARTESIAN_POINT('Ctrl Pts',(-3.4696043187652,-0.707475623527939,
-4.29790785268592));
#48541=CARTESIAN_POINT('Ctrl Pts',(-3.48465193556905,-0.623091478798857,
-4.30079818651808));
#48542=CARTESIAN_POINT('Ctrl Pts',(-3.51856196218893,-0.432930562863846,
-4.3073115964797));
#48543=CARTESIAN_POINT('Ctrl Pts',(-3.5368901719826,-0.240004247211696,
-4.3138250064413));
#48544=CARTESIAN_POINT('Ctrl Pts',(-3.539499078369,-0.0468671734762678,
-4.32033841640292));
#48545=CARTESIAN_POINT('Ctrl Pts',(-3.5418797031369,0.129370235321772,-4.32628189722653));
#48546=CARTESIAN_POINT('Ctrl Pts',(-3.53116871553553,0.305802937702781,
-4.33222537805016));
#48547=CARTESIAN_POINT('Ctrl Pts',(-3.50724735526867,0.480433126417416,
-4.33816885887379));
#48548=CARTESIAN_POINT('Ctrl Pts',(-3.50495350076762,0.497178672654429,
-4.33873878801189));
#48549=CARTESIAN_POINT('Ctrl Pts',(-3.50253818434456,0.513907643630247,
-4.33930871714999));
#48550=CARTESIAN_POINT('Ctrl Pts',(-3.50000197035076,0.530618368380382,
-4.33987864628809));
#48551=CARTESIAN_POINT('Ctrl Pts',(-3.47101696083347,0.72159614750572,-4.34639205624973));
#48552=CARTESIAN_POINT('Ctrl Pts',(-3.42624638929545,0.910161095558849,
-4.35290546621137));
#48553=CARTESIAN_POINT('Ctrl Pts',(-3.36654108656219,1.09385548621155,-4.359418876173));
#48554=CARTESIAN_POINT('Ctrl Pts',(-3.30683578382893,1.27754987686425,-4.36593228613464));
#48555=CARTESIAN_POINT('Ctrl Pts',(-3.23218964468241,1.45639693625083,-4.37244569609627));
#48556=CARTESIAN_POINT('Ctrl Pts',(-3.14342402551079,1.62795644980454,-4.37895910605791));
#48557=CARTESIAN_POINT('Ctrl Pts',(-3.11956799202827,1.67406359734405,-4.38070960504141));
#48558=CARTESIAN_POINT('Ctrl Pts',(-3.09469253710093,1.71964329765716,-4.38246010402492));
#48559=CARTESIAN_POINT('Ctrl Pts',(-3.06881449123183,1.76464659872848,-4.38421060300842));
#48560=CARTESIAN_POINT('Ctrl Pts',(-2.99840323711153,1.88709552257745,-4.38897351398665));
#48561=CARTESIAN_POINT('Ctrl Pts',(-2.92056891533613,2.00527672011598,-4.39373642496487));
#48562=CARTESIAN_POINT('Ctrl Pts',(-2.83599569248695,2.11840306211022,-4.39849933594308));
#48563=CARTESIAN_POINT('Ctrl Pts',(-2.72033951610409,2.27310640345701,-4.4050127459047));
#48564=CARTESIAN_POINT('Ctrl Pts',(-2.59207227250994,2.4183755860845,-4.4115261558663));
#48565=CARTESIAN_POINT('Ctrl Pts',(-2.45286430442405,2.55228290197142,-4.41803956582792));
#48566=CARTESIAN_POINT('Ctrl Pts',(-2.36585966860048,2.63597464327796,-4.42211043094773));
#48567=CARTESIAN_POINT('Ctrl Pts',(-2.27457583085879,2.71523107830464,-4.42618129606755));
#48568=CARTESIAN_POINT('Ctrl Pts',(-2.17944162265286,2.78955806776767,-4.43025216118736));
#48569=CARTESIAN_POINT('Ctrl Pts',(-2.12236049549604,2.83415473196168,-4.43269470602927));
#48570=CARTESIAN_POINT('Ctrl Pts',(-2.06389331379296,2.87697685360123,-4.43513725087118));
#48571=CARTESIAN_POINT('Ctrl Pts',(-2.00416594676152,2.91796018932203,-4.43757979571309));
#48572=CARTESIAN_POINT('Ctrl Pts',(-1.84489401826728,3.02724836391952,-4.44409320567473));
#48573=CARTESIAN_POINT('Ctrl Pts',(-1.67666686505147,3.12346020277471,-4.45060661563637));
#48574=CARTESIAN_POINT('Ctrl Pts',(-1.50177399217723,3.20544206238398,-4.457120025598));
#48575=CARTESIAN_POINT('Ctrl Pts',(-1.33016037878431,3.28588675363412,-4.46351130844821));
#48576=CARTESIAN_POINT('Ctrl Pts',(-1.15210659968557,3.35263728831822,-4.46990259129843));
#48577=CARTESIAN_POINT('Ctrl Pts',(-0.969815634171214,3.40456423580433,
-4.47629387414864));
#48578=CARTESIAN_POINT('Ctrl Pts',(-0.966332347704576,3.40555647605564,
-4.47641600126006));
#48579=CARTESIAN_POINT('Ctrl Pts',(-0.962847514285249,3.40654330398007,
-4.47653812837148));
#48580=CARTESIAN_POINT('Ctrl Pts',(-0.959361151106016,3.4075247180546,-4.47666025548291));
#48581=CARTESIAN_POINT('Ctrl Pts',(-0.773422808690397,3.45986651288758,
-4.48317366544464));
#48582=CARTESIAN_POINT('Ctrl Pts',(-0.583164165584344,3.49679998871353,
-4.48968707540637));
#48583=CARTESIAN_POINT('Ctrl Pts',(-0.391189760153187,3.51811400704572,
-4.4962004853681));
#48584=CARTESIAN_POINT('Ctrl Pts',(-0.199215354724813,3.53942802537761,
-4.50271389532973));
#48585=CARTESIAN_POINT('Ctrl Pts',(-0.00550164725985493,3.54512763200719,
-4.50922730529137));
#48586=CARTESIAN_POINT('Ctrl Pts',(0.187394174250291,3.53498576596323,-4.515740715253));
#48587=CARTESIAN_POINT('Ctrl Pts',(0.25249707115236,3.53156285688057,-4.51793900992778));
#48588=CARTESIAN_POINT('Ctrl Pts',(0.317505759619646,3.52633524440815,-4.52013730460256));
#48589=CARTESIAN_POINT('Ctrl Pts',(0.382317719199291,3.519294412462,-4.52233559927734));
#48590=CARTESIAN_POINT('Ctrl Pts',(0.509539551996122,3.50547369865527,-4.5266507145642));
#48591=CARTESIAN_POINT('Ctrl Pts',(0.636003219410405,3.48466589220727,-4.53096582985105));
#48592=CARTESIAN_POINT('Ctrl Pts',(0.760965615923843,3.45710192869036,-4.53528094513791));
#48593=CARTESIAN_POINT('Ctrl Pts',(0.949588923572606,3.41549576463196,-4.54179435509963));
#48594=CARTESIAN_POINT('Ctrl Pts',(1.13480966416368,3.35849703359421,-4.54830776506137));
#48595=CARTESIAN_POINT('Ctrl Pts',(1.31419238471769,3.28686253261049,-4.55482117502308));
#48596=CARTESIAN_POINT('Ctrl Pts',(1.43863859651384,3.23716631742433,-4.55933983319209));
#48597=CARTESIAN_POINT('Ctrl Pts',(1.56028265268397,3.18042068936791,-4.56385849136109));
#48598=CARTESIAN_POINT('Ctrl Pts',(1.67827226002658,3.1168898314225,-4.5683771495301));
#48599=CARTESIAN_POINT('Ctrl Pts',(1.73035851482898,3.08884427275604,-4.5703719013227));
#48600=CARTESIAN_POINT('Ctrl Pts',(1.78173265010367,3.05947655931791,-4.57236665311531));
#48601=CARTESIAN_POINT('Ctrl Pts',(1.83233522030034,3.02883524024529,-4.57436140490792));
#48602=CARTESIAN_POINT('Ctrl Pts',(1.99756644657541,2.92878295623329,-4.58087481486964));
#48603=CARTESIAN_POINT('Ctrl Pts',(2.15456198585818,2.81515968928226,-4.58738822483137));
#48604=CARTESIAN_POINT('Ctrl Pts',(2.30134084431348,2.68960344508741,-4.59390163479326));
#48605=CARTESIAN_POINT('Ctrl Pts',(2.44811970276666,2.56404720089438,-4.60041504475506));
#48606=CARTESIAN_POINT('Ctrl Pts',(2.58469882886557,2.42654092551998,-4.60692845471703));
#48607=CARTESIAN_POINT('Ctrl Pts',(2.70905533377063,2.2787296820682,-4.61344186467883));
#48608=CARTESIAN_POINT('Ctrl Pts',(2.71527320777415,2.2713390619411,-4.61376753773073));
#48609=CARTESIAN_POINT('Ctrl Pts',(2.72146047398848,2.26392273951171,-4.61409321078263));
#48610=CARTESIAN_POINT('Ctrl Pts',(2.72761687942599,2.25648092371001,-4.61441888383453));
#48611=CARTESIAN_POINT('Ctrl Pts',(2.84458761721353,2.1150875905972,-4.62060662074442));
#48612=CARTESIAN_POINT('Ctrl Pts',(2.95041694207574,1.96449093844901,-4.62679435765416));
#48613=CARTESIAN_POINT('Ctrl Pts',(3.04403466981377,1.80667228922409,-4.63298209456391));
#48614=CARTESIAN_POINT('Ctrl Pts',(3.14257968705312,1.64054732673751,-4.63949550452564));
#48615=CARTESIAN_POINT('Ctrl Pts',(3.2276089004457,1.4664013198912,-4.64600891448737));
#48616=CARTESIAN_POINT('Ctrl Pts',(3.29789079596611,1.2864798567823,-4.65252232444909));
#48617=CARTESIAN_POINT('Ctrl Pts',(3.32644295523914,1.21338640599696,-4.65516841014813));
#48618=CARTESIAN_POINT('Ctrl Pts',(3.35256060096538,1.13933993490305,-4.65781449584717));
#48619=CARTESIAN_POINT('Ctrl Pts',(3.37615800564866,1.06449853024478,-4.66046058154621));
#48620=CARTESIAN_POINT('Ctrl Pts',(3.410646236963,0.955115837089003,-4.66432790580881));
#48621=CARTESIAN_POINT('Ctrl Pts',(3.43975080156849,0.844035097395934,-4.6681952300714));
#48622=CARTESIAN_POINT('Ctrl Pts',(3.46340847798809,0.731814199250707,-4.672062554334));
#48623=CARTESIAN_POINT('Ctrl Pts',(3.50325311857094,0.542809950770156,-4.67857596429564));
#48624=CARTESIAN_POINT('Ctrl Pts',(3.52765418600473,0.350559382295599,-4.68508937425727));
#48625=CARTESIAN_POINT('Ctrl Pts',(3.53632795873358,0.157598006434378,-4.69160278421891));
#48626=CARTESIAN_POINT('Ctrl Pts',(3.54294168510181,0.0104655210122198,
-4.69656924028791));
#48627=CARTESIAN_POINT('Ctrl Pts',(3.54040940290031,-0.137092750504991,
-4.70153569635691));
#48628=CARTESIAN_POINT('Ctrl Pts',(3.52859722973483,-0.283904192124258,
-4.7065021524259));
#48629=CARTESIAN_POINT('Ctrl Pts',(3.52491796890859,-0.329633083703001,
-4.70804910631863));
#48630=CARTESIAN_POINT('Ctrl Pts',(3.52033846393456,-0.375289512400935,
-4.70959606021136));
#48631=CARTESIAN_POINT('Ctrl Pts',(3.5148682535165,-0.420839119723915,-4.71114301410408));
#48632=CARTESIAN_POINT('Ctrl Pts',(3.49183607188734,-0.612624581126916,
-4.7176564240657));
#48633=CARTESIAN_POINT('Ctrl Pts',(3.4530172602035,-0.80249780061272,-4.7241698340273));
#48634=CARTESIAN_POINT('Ctrl Pts',(3.3991184205719,-0.987978897271879,-4.73068324398892));
#48635=CARTESIAN_POINT('Ctrl Pts',(3.34521958093952,-1.17345999393373,-4.73719665395063));
#48636=CARTESIAN_POINT('Ctrl Pts',(3.2762331580479,-1.35457174622048,-4.74371006391237));
#48637=CARTESIAN_POINT('Ctrl Pts',(3.19284833403879,-1.52881164096968,-4.75022347387409));
#48638=CARTESIAN_POINT('Ctrl Pts',(3.18294627225166,-1.5495028665505,-4.7509969502069));
#48639=CARTESIAN_POINT('Ctrl Pts',(3.17284133069424,-1.57009682188359,-4.7517704265397));
#48640=CARTESIAN_POINT('Ctrl Pts',(3.1625347146805,-1.5905892551004,-4.7525439028725));
#48641=CARTESIAN_POINT('Ctrl Pts',(3.08604977345116,-1.74266269493216,-4.75828383650133));
#48642=CARTESIAN_POINT('Ctrl Pts',(2.99845761324308,-1.88914457163618,-4.76402377013017));
#48643=CARTESIAN_POINT('Ctrl Pts',(2.90086776956525,-2.02860868265436,-4.769763703759));
#48644=CARTESIAN_POINT('Ctrl Pts',(2.79012734971569,-2.18686607528926,-4.77627711372064));
#48645=CARTESIAN_POINT('Ctrl Pts',(2.6665030824214,-2.33610851677235,-4.78279052368227));
#48646=CARTESIAN_POINT('Ctrl Pts',(2.53155468743157,-2.47431060311237,-4.78930393364391));
#48647=CARTESIAN_POINT('Ctrl Pts',(2.46745412259722,-2.53995667319974,-4.7923978071025));
#48648=CARTESIAN_POINT('Ctrl Pts',(2.40079731960751,-2.60311185453884,-4.79549168056109));
#48649=CARTESIAN_POINT('Ctrl Pts',(2.33176068881981,-2.66354877749069,-4.79858555401968));
#48650=CARTESIAN_POINT('Ctrl Pts',(2.25545721933669,-2.7303473285424,-4.80200509052282));
#48651=CARTESIAN_POINT('Ctrl Pts',(2.17624654724241,-2.79382517537667,-4.80542462702596));
#48652=CARTESIAN_POINT('Ctrl Pts',(2.09446454668198,-2.85378693812754,-4.80884416352909));
#48653=CARTESIAN_POINT('Ctrl Pts',(1.93868913775044,-2.96799994403061,-4.81535757349073));
#48654=CARTESIAN_POINT('Ctrl Pts',(1.77358024536384,-3.06946424600634,-4.82187098345237));
#48655=CARTESIAN_POINT('Ctrl Pts',(1.60134875634575,-3.15690183524312,-4.828384393414));
#48656=CARTESIAN_POINT('Ctrl Pts',(1.45818170002382,-3.22958414400259,-4.83379865149271));
#48657=CARTESIAN_POINT('Ctrl Pts',(1.31007763847309,-3.29257884054208,-4.83921290957143));
#48658=CARTESIAN_POINT('Ctrl Pts',(1.15835136238572,-3.34511914903784,-4.84462716765014));
#48659=CARTESIAN_POINT('Ctrl Pts',(1.12754931718851,-3.35578538957768,-4.84572631953306));
#48660=CARTESIAN_POINT('Ctrl Pts',(1.09659801000313,-3.36602081032388,-4.84682547141599));
#48661=CARTESIAN_POINT('Ctrl Pts',(1.06551003781568,-3.37582359101795,-4.84792462329891));
#48662=CARTESIAN_POINT('Ctrl Pts',(0.8812873558714,-3.43391340591755,-4.85443803326064));
#48663=CARTESIAN_POINT('Ctrl Pts',(0.692289542666389,-3.47680428037546,
-4.86095144322237));
#48664=CARTESIAN_POINT('Ctrl Pts',(0.501080685143525,-3.50414476472143,
-4.86746485318408));
#48665=CARTESIAN_POINT('Ctrl Pts',(0.309871827623432,-3.53148524906699,
-4.8739782631457));
#48666=CARTESIAN_POINT('Ctrl Pts',(0.116428217970221,-3.54327886708705,
-4.8804916731073));
#48667=CARTESIAN_POINT('Ctrl Pts',(-0.0766918204989502,-3.53915174526628,
-4.88700508306892));
#48668=CARTESIAN_POINT('Ctrl Pts',(-0.112902286566704,-3.53837790011881,
-4.88822636291264));
#48669=CARTESIAN_POINT('Ctrl Pts',(-0.149100544630311,-3.53704430365368,
-4.88944764275636));
#48670=CARTESIAN_POINT('Ctrl Pts',(-0.185269285100072,-3.53514855303133,
-4.89066892260008));
#48671=CARTESIAN_POINT('Ctrl Pts',(-0.341998049399606,-3.52693376178892,
-4.89596105271809));
#48672=CARTESIAN_POINT('Ctrl Pts',(-0.49817233969735,-3.50816226468903,
-4.90125318283612));
#48673=CARTESIAN_POINT('Ctrl Pts',(-0.652411741910373,-3.47918285964478,
-4.90654531295425));
#48674=CARTESIAN_POINT('Ctrl Pts',(-0.842245398493005,-3.44351579697333,
-4.91305872260848));
#48675=CARTESIAN_POINT('Ctrl Pts',(-1.02917125546825,-3.3923861748366,-4.91957213226287));
#48676=CARTESIAN_POINT('Ctrl Pts',(-1.21071388570407,-3.32640898834169,
-4.92608554191631));
#48677=CARTESIAN_POINT('',(-1.210751307373,-3.326511877582,-4.926085542839));
#48678=CARTESIAN_POINT('Ctrl Pts',(-3.841349734859,-1.189096377216,-1.539436278284));
#48679=CARTESIAN_POINT('Ctrl Pts',(-3.994234933732,-0.6952040995074,-1.554783500506));
#48680=CARTESIAN_POINT('Ctrl Pts',(-4.10706259235,0.3520715397013,-1.58547794495));
#48681=CARTESIAN_POINT('Ctrl Pts',(-3.672853039324,1.871418570915,-1.631519611617));
#48682=CARTESIAN_POINT('Ctrl Pts',(-2.698930474802,3.115729236588,-1.677561278284));
#48683=CARTESIAN_POINT('Ctrl Pts',(-1.328423408128,3.902218173295,-1.72360294495));
#48684=CARTESIAN_POINT('Ctrl Pts',(0.2372868317335,4.115301255755,-1.769644611617));
#48685=CARTESIAN_POINT('Ctrl Pts',(1.76812922683,3.723671568578,-1.815686278284));
#48686=CARTESIAN_POINT('Ctrl Pts',(3.039157943544,2.784875152802,-1.86172794495));
#48687=CARTESIAN_POINT('Ctrl Pts',(3.863604450802,1.43686161852,-1.907769611617));
#48688=CARTESIAN_POINT('Ctrl Pts',(4.120322345675,-0.1222883131347,-1.953811278284));
#48689=CARTESIAN_POINT('Ctrl Pts',(3.771588791194,-1.663468860739,-1.99985294495));
#48690=CARTESIAN_POINT('Ctrl Pts',(2.868647652528,-2.960214740138,-2.045894611617));
#48691=CARTESIAN_POINT('Ctrl Pts',(1.544179572608,-3.821978559474,-2.091936278284));
#48692=CARTESIAN_POINT('Ctrl Pts',(-0.007194482043365,-4.122130383809,-2.13797794495));
#48693=CARTESIAN_POINT('Ctrl Pts',(-1.557511359811,-3.816565082075,-2.184019611617));
#48694=CARTESIAN_POINT('Ctrl Pts',(-2.8789632535,-2.950183256454,-2.230061278284));
#48695=CARTESIAN_POINT('Ctrl Pts',(-3.777372403381,-1.65029342477,-2.27610294495));
#48696=CARTESIAN_POINT('Ctrl Pts',(-4.120724108895,-0.1079049583238,-2.322144611617));
#48697=CARTESIAN_POINT('Ctrl Pts',(-3.85856533025,1.45033935817,-2.368186278284));
#48698=CARTESIAN_POINT('Ctrl Pts',(-3.029418396237,2.795466837973,-2.41422794495));
#48699=CARTESIAN_POINT('Ctrl Pts',(-1.755120427756,3.7298207659,-2.460269611617));
#48700=CARTESIAN_POINT('Ctrl Pts',(-0.2229202576515,4.11610461728,-2.506311278284));
#48701=CARTESIAN_POINT('Ctrl Pts',(1.342036425525,3.897556785247,-2.55235294495));
#48702=CARTESIAN_POINT('Ctrl Pts',(2.709790601495,3.106291286681,-2.598394611617));
#48703=CARTESIAN_POINT('Ctrl Pts',(3.679360726381,1.858578840628,-2.644436278284));
#48704=CARTESIAN_POINT('Ctrl Pts',(4.108275511099,0.337761730468,-2.69047794495));
#48705=CARTESIAN_POINT('Ctrl Pts',(3.933509042705,-1.232687013245,-2.736519611617));
#48706=CARTESIAN_POINT('Ctrl Pts',(3.180741984619,-2.622001351819,-2.782561278284));
#48707=CARTESIAN_POINT('Ctrl Pts',(1.960587989627,-3.626031632045,-2.82860294495));
#48708=CARTESIAN_POINT('Ctrl Pts',(0.4523398268471,-4.097242895254,-2.874644611617));
#48709=CARTESIAN_POINT('Ctrl Pts',(-1.122376388713,-3.966394068133,-2.920686278284));
#48710=CARTESIAN_POINT('Ctrl Pts',(-2.532167544361,-3.252712435637,-2.96672794495));
#48711=CARTESIAN_POINT('Ctrl Pts',(-3.569875067316,-2.061068331088,-3.012769611617));
#48712=CARTESIAN_POINT('Ctrl Pts',(-4.083015372648,-0.566565202236,-3.058811278284));
#48713=CARTESIAN_POINT('Ctrl Pts',(-3.99618621878,1.011190568834,-3.10485294495));
#48714=CARTESIAN_POINT('Ctrl Pts',(-3.322146519342,2.44035922882,-3.150894611617));
#48715=CARTESIAN_POINT('Ctrl Pts',(-2.159941513463,3.510934821395,-3.196936278284));
#48716=CARTESIAN_POINT('Ctrl Pts',(-0.6803487871228,4.065604037474,-3.24297794495));
#48717=CARTESIAN_POINT('Ctrl Pts',(0.8992162529668,4.022862263621,-3.289019611617));
#48718=CARTESIAN_POINT('Ctrl Pts',(2.346647994561,3.388990093123,-3.335061278284));
#48719=CARTESIAN_POINT('Ctrl Pts',(3.44925685411,2.257130438418,-3.38110294495));
#48720=CARTESIAN_POINT('Ctrl Pts',(4.045022466568,0.7936018564908,-3.427144611617));
#48721=CARTESIAN_POINT('Ctrl Pts',(4.046401401479,-0.7865407553148,-3.473186278284));
#48722=CARTESIAN_POINT('Ctrl Pts',(3.453191034373,-2.251106914784,-3.51922794495));
#48723=CARTESIAN_POINT('Ctrl Pts',(2.352559320954,-3.384889260088,-3.565269611617));
#48724=CARTESIAN_POINT('Ctrl Pts',(0.9062360990033,-4.021286708819,-3.611311278284));
#48725=CARTESIAN_POINT('Ctrl Pts',(-0.6732519368415,-4.066785277243,-3.65735294495));
#48726=CARTESIAN_POINT('Ctrl Pts',(-2.15381048955,-3.514699281129,-3.703394611617));
#48727=CARTESIAN_POINT('Ctrl Pts',(-3.31788223124,-2.446153748497,-3.749436278284));
#48728=CARTESIAN_POINT('Ctrl Pts',(-3.994415272659,-1.018163685866,-3.79547794495));
#48729=CARTESIAN_POINT('Ctrl Pts',(-4.083997996179,0.559438136759,-3.841519611617));
#48730=CARTESIAN_POINT('Ctrl Pts',(-3.573466871112,2.054834587688,-3.887561278284));
#48731=CARTESIAN_POINT('Ctrl Pts',(-2.537840738919,3.248288017621,-3.93360294495));
#48732=CARTESIAN_POINT('Ctrl Pts',(-1.129297339352,3.964429111665,-3.979644611617));
#48733=CARTESIAN_POINT('Ctrl Pts',(0.4451881037925,4.098026136172,-4.025686278284));
#48734=CARTESIAN_POINT('Ctrl Pts',(1.954256387077,3.629447979702,-4.07172794495));
#48735=CARTESIAN_POINT('Ctrl Pts',(3.176160888763,2.627548795309,-4.117769611617));
#48736=CARTESIAN_POINT('Ctrl Pts',(3.931351600467,1.239550408822,-4.163811278284));
#48737=CARTESIAN_POINT('Ctrl Pts',(4.108858787154,-0.3305909566808,-4.20985294495));
#48738=CARTESIAN_POINT('Ctrl Pts',(3.682598847576,-1.852154203613,-4.255894611617));
#48739=CARTESIAN_POINT('Ctrl Pts',(2.715208365118,-3.101557505068,-4.301936278284));
#48740=CARTESIAN_POINT('Ctrl Pts',(1.348835432798,-3.89520697252,-4.34797794495));
#48741=CARTESIAN_POINT('Ctrl Pts',(-0.2157304961352,-4.116493321879,-4.394019611617));
#48742=CARTESIAN_POINT('Ctrl Pts',(-1.748628398844,-3.732856309759,-4.440061278284));
#48743=CARTESIAN_POINT('Ctrl Pts',(-2.599181877855,-3.111506871542,-4.470755722728));
#48744=CARTESIAN_POINT('Ctrl Pts',(-2.950462537646,-2.7321582666,-4.48610294495));
#48745=CARTESIAN_POINT('Ctrl Pts',(-3.681382861754,-1.139578358183,-1.636116911815));
#48746=CARTESIAN_POINT('Ctrl Pts',(-3.827901400756,-0.6662534353805,-1.651464134037));
#48747=CARTESIAN_POINT('Ctrl Pts',(-3.936030531775,0.337410082869,-1.682158578481));
#48748=CARTESIAN_POINT('Ctrl Pts',(-3.519902941929,1.793486334144,-1.728200245148));
#48749=CARTESIAN_POINT('Ctrl Pts',(-2.586537826753,2.985979669945,-1.774241911815));
#48750=CARTESIAN_POINT('Ctrl Pts',(-1.27310333747,3.739716531309,-1.820283578481));
#48751=CARTESIAN_POINT('Ctrl Pts',(0.2274054006946,3.943926109203,-1.866325245148));
#48752=CARTESIAN_POINT('Ctrl Pts',(1.694498309787,3.568605214716,-1.912366911815));
#48753=CARTESIAN_POINT('Ctrl Pts',(2.912597066077,2.668903475936,-1.958408578481));
#48754=CARTESIAN_POINT('Ctrl Pts',(3.702710815604,1.377025811821,-2.004450245148));
#48755=CARTESIAN_POINT('Ctrl Pts',(3.948738103854,-0.1171958116913,-2.050491911815));
#48756=CARTESIAN_POINT('Ctrl Pts',(3.614527001144,-1.594196357445,-2.096533578481));
#48757=CARTESIAN_POINT('Ctrl Pts',(2.749187403738,-2.836941326264,-2.142575245148));
#48758=CARTESIAN_POINT('Ctrl Pts',(1.479874681153,-3.662818368022,-2.188616911815));
#48759=CARTESIAN_POINT('Ctrl Pts',(-0.006894879331943,-3.950470849129,-2.234658578481));
#48760=CARTESIAN_POINT('Ctrl Pts',(-1.492651287375,-3.657630326242,-2.280700245148));
#48761=CARTESIAN_POINT('Ctrl Pts',(-2.759073427987,-2.827327587693,-2.326741911815));
#48762=CARTESIAN_POINT('Ctrl Pts',(-3.620069764041,-1.581569591459,-2.372783578481));
#48763=CARTESIAN_POINT('Ctrl Pts',(-3.949123136288,-0.1034114287139,-2.418825245148));
#48764=CARTESIAN_POINT('Ctrl Pts',(-3.697881541177,1.389942292534,-2.464866911815));
#48765=CARTESIAN_POINT('Ctrl Pts',(-2.903263106658,2.679054087298,-2.510908578481));
#48766=CARTESIAN_POINT('Ctrl Pts',(-1.682031241369,3.574498338538,-2.556950245148));
#48767=CARTESIAN_POINT('Ctrl Pts',(-0.2136370996395,3.944696016021,-2.602991911815));
#48768=CARTESIAN_POINT('Ctrl Pts',(1.286149462504,3.73524925932,-2.649033578481));
#48769=CARTESIAN_POINT('Ctrl Pts',(2.59694570082,2.976934748386,-2.695075245148));
#48770=CARTESIAN_POINT('Ctrl Pts',(3.526139626754,1.781181293913,-2.741116911815));
#48771=CARTESIAN_POINT('Ctrl Pts',(3.93719294046,0.3236961827811,-2.787158578481));
#48772=CARTESIAN_POINT('Ctrl Pts',(3.76970434245,-1.181353731811,-2.833200245148));
#48773=CARTESIAN_POINT('Ctrl Pts',(3.048285065944,-2.512812294202,-2.879241911815));
#48774=CARTESIAN_POINT('Ctrl Pts',(1.878942434863,-3.475031337359,-2.925283578481));
#48775=CARTESIAN_POINT('Ctrl Pts',(0.4335028573765,-3.926619760277,-2.971325245148));
#48776=CARTESIAN_POINT('Ctrl Pts',(-1.075636817015,-3.801219923529,-3.017366911815));
#48777=CARTESIAN_POINT('Ctrl Pts',(-2.426719472144,-3.117258422503,-3.063408578481));
#48778=CARTESIAN_POINT('Ctrl Pts',(-3.421213323057,-1.975238433022,-3.109450245148));
#48779=CARTESIAN_POINT('Ctrl Pts',(-3.912984720121,-0.5429714994837,-3.155491911815));
#48780=CARTESIAN_POINT('Ctrl Pts',(-3.829771427655,0.969081152984,-3.201533578481));
#48781=CARTESIAN_POINT('Ctrl Pts',(-3.183801034714,2.33873436724,-3.247575245148));
#48782=CARTESIAN_POINT('Ctrl Pts',(-2.069994199668,3.364727549519,-3.293616911815));
#48783=CARTESIAN_POINT('Ctrl Pts',(-0.6520167487486,3.896298452185,-3.339658578481));
#48784=CARTESIAN_POINT('Ctrl Pts',(0.861769828621,3.855336591224,-3.385700245148));
#48785=CARTESIAN_POINT('Ctrl Pts',(2.248925587626,3.247861014648,-3.431741911815));
#48786=CARTESIAN_POINT('Ctrl Pts',(3.305618062651,2.163135847104,-3.477783578481));
#48787=CARTESIAN_POINT('Ctrl Pts',(3.87657396792,0.760553574966,-3.523825245148));
#48788=CARTESIAN_POINT('Ctrl Pts',(3.87789547929,-0.7537865220682,-3.569866911815));
#48789=CARTESIAN_POINT('Ctrl Pts',(3.309388410261,-2.157363163489,-3.615908578481));
#48790=CARTESIAN_POINT('Ctrl Pts',(2.254590746275,-3.243930954253,-3.661950245148));
#48791=CARTESIAN_POINT('Ctrl Pts',(0.8684973443836,-3.853826647885,-3.707991911815));
#48792=CARTESIAN_POINT('Ctrl Pts',(-0.64521543546,-3.897430501112,-3.754033578481));
#48793=CARTESIAN_POINT('Ctrl Pts',(-2.064118492452,-3.368335244341,-3.800075245148));
#48794=CARTESIAN_POINT('Ctrl Pts',(-3.179714326077,-2.344287583402,-3.846116911815));
#48795=CARTESIAN_POINT('Ctrl Pts',(-3.828074229756,-0.9757638856968,-3.892158578481));
#48796=CARTESIAN_POINT('Ctrl Pts',(-3.913926423865,0.5361412292629,-3.938200245148));
#48797=CARTESIAN_POINT('Ctrl Pts',(-3.424655551922,1.969264283907,-3.984241911815));
#48798=CARTESIAN_POINT('Ctrl Pts',(-2.432156415579,3.113018252307,-4.030283578481));
#48799=CARTESIAN_POINT('Ctrl Pts',(-1.082269555721,3.799336794534,-4.076325245148));
#48800=CARTESIAN_POINT('Ctrl Pts',(0.4266489564036,3.927370384378,-4.122366911815));
#48801=CARTESIAN_POINT('Ctrl Pts',(1.872874501785,3.478305416675,-4.168408578481));
#48802=CARTESIAN_POINT('Ctrl Pts',(3.043894742506,2.51812872327,-4.214450245148));
#48803=CARTESIAN_POINT('Ctrl Pts',(3.767636743447,1.187931312243,-4.260491911815));
#48804=CARTESIAN_POINT('Ctrl Pts',(3.937751926915,-0.3168240244129,-4.306533578481));
#48805=CARTESIAN_POINT('Ctrl Pts',(3.529242901566,-1.775024200642,-4.352575245148));
#48806=CARTESIAN_POINT('Ctrl Pts',(2.602137850332,-2.972398097546,-4.398616911815));
#48807=CARTESIAN_POINT('Ctrl Pts',(1.29266533598,-3.73299730079,-4.444658578481));
#48808=CARTESIAN_POINT('Ctrl Pts',(-0.2067467442558,-3.945068533638,-4.490700245148));
#48809=CARTESIAN_POINT('Ctrl Pts',(-1.67580956263,-3.577407472023,-4.536741911815));
#48810=CARTESIAN_POINT('Ctrl Pts',(-2.490943100776,-2.981933138547,-4.567436356259));
#48811=CARTESIAN_POINT('Ctrl Pts',(-2.827595238666,-2.618381900244,-4.582783578481));
#48812=CARTESIAN_POINT('Ctrl Pts',(-3.521415988649,-1.090060339149,-1.732797545346));
#48813=CARTESIAN_POINT('Ctrl Pts',(-3.66156786778,-0.6373027712535,-1.748144767568));
#48814=CARTESIAN_POINT('Ctrl Pts',(-3.764998471199,0.3227486260367,-1.778839212012));
#48815=CARTESIAN_POINT('Ctrl Pts',(-3.366952844534,1.715554097372,-1.824880878679));
#48816=CARTESIAN_POINT('Ctrl Pts',(-2.474145178704,2.856230103303,-1.870922545346));
#48817=CARTESIAN_POINT('Ctrl Pts',(-1.217783266811,3.577214889324,-1.916964212012));
#48818=CARTESIAN_POINT('Ctrl Pts',(0.2175239696557,3.772550962651,-1.963005878679));
#48819=CARTESIAN_POINT('Ctrl Pts',(1.620867392743,3.413538860853,-2.009047545346));
#48820=CARTESIAN_POINT('Ctrl Pts',(2.78603618861,2.552931799069,-2.055089212012));
#48821=CARTESIAN_POINT('Ctrl Pts',(3.541817180406,1.317190005122,-2.101130878679));
#48822=CARTESIAN_POINT('Ctrl Pts',(3.777153862034,-0.1121033102479,-2.147172545346));
#48823=CARTESIAN_POINT('Ctrl Pts',(3.457465211094,-1.524923854152,-2.193214212012));
#48824=CARTESIAN_POINT('Ctrl Pts',(2.629727154949,-2.71366791239,-2.239255878679));
#48825=CARTESIAN_POINT('Ctrl Pts',(1.415569789697,-3.50365817657,-2.285297545346));
#48826=CARTESIAN_POINT('Ctrl Pts',(-0.006595276620518,-3.778811314449,-2.331339212012));
#48827=CARTESIAN_POINT('Ctrl Pts',(-1.427791214939,-3.498695570408,-2.377380878679));
#48828=CARTESIAN_POINT('Ctrl Pts',(-2.639183602474,-2.704471918932,-2.423422545346));
#48829=CARTESIAN_POINT('Ctrl Pts',(-3.462767124701,-1.512845758149,-2.469464212012));
#48830=CARTESIAN_POINT('Ctrl Pts',(-3.77752216368,-0.09891789910402,-2.515505878679));
#48831=CARTESIAN_POINT('Ctrl Pts',(-3.537197752104,1.329545226898,-2.561547545346));
#48832=CARTESIAN_POINT('Ctrl Pts',(-2.77710781708,2.562641336623,-2.607589212012));
#48833=CARTESIAN_POINT('Ctrl Pts',(-1.608942054981,3.419175911177,-2.653630878679));
#48834=CARTESIAN_POINT('Ctrl Pts',(-0.2043539416274,3.773287414762,-2.699672545346));
#48835=CARTESIAN_POINT('Ctrl Pts',(1.230262499482,3.572941733393,-2.745714212012));
#48836=CARTESIAN_POINT('Ctrl Pts',(2.484100800144,2.84757821009,-2.791755878679));
#48837=CARTESIAN_POINT('Ctrl Pts',(3.372918527128,1.703783747197,-2.837797545346));
#48838=CARTESIAN_POINT('Ctrl Pts',(3.76611036982,0.3096306350943,-2.883839212012));
#48839=CARTESIAN_POINT('Ctrl Pts',(3.605899642196,-1.130020450377,-2.929880878679));
#48840=CARTESIAN_POINT('Ctrl Pts',(2.915828147269,-2.403623236585,-2.975922545346));
#48841=CARTESIAN_POINT('Ctrl Pts',(1.797296880098,-3.324031042672,-3.021964212012));
#48842=CARTESIAN_POINT('Ctrl Pts',(0.4146658879059,-3.7559966253,-3.068005878679));
#48843=CARTESIAN_POINT('Ctrl Pts',(-1.028897245317,-3.636045778925,-3.114047545346));
#48844=CARTESIAN_POINT('Ctrl Pts',(-2.321271399928,-2.981804409369,-3.160089212012));
#48845=CARTESIAN_POINT('Ctrl Pts',(-3.272551578798,-1.889408534956,-3.206130878679));
#48846=CARTESIAN_POINT('Ctrl Pts',(-3.742954067594,-0.5193777967315,-3.252172545346));
#48847=CARTESIAN_POINT('Ctrl Pts',(-3.66335663653,0.9269717371343,-3.298214212012));
#48848=CARTESIAN_POINT('Ctrl Pts',(-3.045455550085,2.237109505659,-3.344255878679));
#48849=CARTESIAN_POINT('Ctrl Pts',(-1.980046885873,3.218520277643,-3.390297545346));
#48850=CARTESIAN_POINT('Ctrl Pts',(-0.6236847103744,3.726992866897,-3.436339212012));
#48851=CARTESIAN_POINT('Ctrl Pts',(0.8243234042752,3.687810918827,-3.482380878679));
#48852=CARTESIAN_POINT('Ctrl Pts',(2.151203180692,3.106731936173,-3.528422545346));
#48853=CARTESIAN_POINT('Ctrl Pts',(3.161979271192,2.06914125579,-3.574464212012));
#48854=CARTESIAN_POINT('Ctrl Pts',(3.708125469273,0.7275052934411,-3.620505878679));
#48855=CARTESIAN_POINT('Ctrl Pts',(3.709389557102,-0.7210322888216,-3.666547545346));
#48856=CARTESIAN_POINT('Ctrl Pts',(3.16558578615,-2.063619412194,-3.712589212012));
#48857=CARTESIAN_POINT('Ctrl Pts',(2.156622171596,-3.102972648419,-3.758630878679));
#48858=CARTESIAN_POINT('Ctrl Pts',(0.8307585897638,-3.686366586951,-3.804672545346));
#48859=CARTESIAN_POINT('Ctrl Pts',(-0.6171789340784,-3.72807572498,-3.850714212012));
#48860=CARTESIAN_POINT('Ctrl Pts',(-1.974426495353,-3.221971207554,-3.896755878679));
#48861=CARTESIAN_POINT('Ctrl Pts',(-3.041546420915,-2.242421418306,-3.942797545346));
#48862=CARTESIAN_POINT('Ctrl Pts',(-3.661733186854,-0.9333640855279,-3.988839212012));
#48863=CARTESIAN_POINT('Ctrl Pts',(-3.743854851551,0.5128443217669,-4.034880878679));
#48864=CARTESIAN_POINT('Ctrl Pts',(-3.275844232732,1.883693980126,-4.080922545346));
#48865=CARTESIAN_POINT('Ctrl Pts',(-2.326472092238,2.977748486993,-4.126964212012));
#48866=CARTESIAN_POINT('Ctrl Pts',(-1.03524177209,3.634244477402,-4.173005878679));
#48867=CARTESIAN_POINT('Ctrl Pts',(0.4081098090146,3.756714632584,-4.219047545346));
#48868=CARTESIAN_POINT('Ctrl Pts',(1.791492616494,3.327162853648,-4.265089212012));
#48869=CARTESIAN_POINT('Ctrl Pts',(2.911628596249,2.40870865123,-4.311130878679));
#48870=CARTESIAN_POINT('Ctrl Pts',(3.603921886428,1.136312215665,-4.357172545346));
#48871=CARTESIAN_POINT('Ctrl Pts',(3.766645066676,-0.303057092145,-4.403214212012));
#48872=CARTESIAN_POINT('Ctrl Pts',(3.375886955555,-1.697894197672,-4.449255878679));
#48873=CARTESIAN_POINT('Ctrl Pts',(2.489067335545,-2.843238690024,-4.495297545346));
#48874=CARTESIAN_POINT('Ctrl Pts',(1.236495239162,-3.570787629061,-4.541339212012));
#48875=CARTESIAN_POINT('Ctrl Pts',(-0.1977629923763,-3.773643745397,-4.587380878679));
#48876=CARTESIAN_POINT('Ctrl Pts',(-1.602990726415,-3.421958634286,-4.633422545346));
#48877=CARTESIAN_POINT('Ctrl Pts',(-2.382704323698,-2.852359405552,-4.66411698979));
#48878=CARTESIAN_POINT('Ctrl Pts',(-2.704727939686,-2.504605533888,-4.679464212012));
#48879=CARTESIAN_POINT('Ctrl Pts',(-3.361449115544,-1.040542320116,-1.829478178877));
#48880=CARTESIAN_POINT('Ctrl Pts',(-3.495234334804,-0.6083521071266,-1.844825401099));
#48881=CARTESIAN_POINT('Ctrl Pts',(-3.593966410624,0.3080871692045,-1.875519845544));
#48882=CARTESIAN_POINT('Ctrl Pts',(-3.214002747139,1.6376218606,-1.92156151221));
#48883=CARTESIAN_POINT('Ctrl Pts',(-2.361752530656,2.726480536661,-1.967603178877));
#48884=CARTESIAN_POINT('Ctrl Pts',(-1.162463196152,3.414713247338,-2.013644845544));
#48885=CARTESIAN_POINT('Ctrl Pts',(0.2076425386167,3.6011758161,-2.05968651221));
#48886=CARTESIAN_POINT('Ctrl Pts',(1.5472364757,3.258472506991,-2.105728178877));
#48887=CARTESIAN_POINT('Ctrl Pts',(2.659475311144,2.436960122203,-2.151769845544));
#48888=CARTESIAN_POINT('Ctrl Pts',(3.380923545207,1.257354198423,-2.19781151221));
#48889=CARTESIAN_POINT('Ctrl Pts',(3.605569620214,-0.1070108088044,-2.243853178877));
#48890=CARTESIAN_POINT('Ctrl Pts',(3.300403421044,-1.455651350858,-2.289894845544));
#48891=CARTESIAN_POINT('Ctrl Pts',(2.510266906159,-2.590394498517,-2.33593651221));
#48892=CARTESIAN_POINT('Ctrl Pts',(1.351264898242,-3.344497985119,-2.381978178877));
#48893=CARTESIAN_POINT('Ctrl Pts',(-0.006295673909096,-3.607151779769,-2.428019845544));
#48894=CARTESIAN_POINT('Ctrl Pts',(-1.362931142503,-3.339760814575,-2.47406151221));
#48895=CARTESIAN_POINT('Ctrl Pts',(-2.519293776961,-2.581616250171,-2.520103178877));
#48896=CARTESIAN_POINT('Ctrl Pts',(-3.305464485361,-1.444121924838,-2.566144845544));
#48897=CARTESIAN_POINT('Ctrl Pts',(-3.605921191072,-0.09442436949412,-2.61218651221));
#48898=CARTESIAN_POINT('Ctrl Pts',(-3.376513963031,1.269148161262,-2.658228178877));
#48899=CARTESIAN_POINT('Ctrl Pts',(-2.650952527502,2.446228585948,-2.704269845544));
#48900=CARTESIAN_POINT('Ctrl Pts',(-1.535852868594,3.263853483815,-2.75031151221));
#48901=CARTESIAN_POINT('Ctrl Pts',(-0.1950707836154,3.601878813503,-2.796353178877));
#48902=CARTESIAN_POINT('Ctrl Pts',(1.174375536461,3.410634207467,-2.842394845544));
#48903=CARTESIAN_POINT('Ctrl Pts',(2.371255899469,2.718221671795,-2.88843651221));
#48904=CARTESIAN_POINT('Ctrl Pts',(3.219697427502,1.626386200482,-2.934478178877));
#48905=CARTESIAN_POINT('Ctrl Pts',(3.595027799181,0.2955650874075,-2.980519845544));
#48906=CARTESIAN_POINT('Ctrl Pts',(3.442094941941,-1.078687168943,-3.02656151221));
#48907=CARTESIAN_POINT('Ctrl Pts',(2.783371228594,-2.294434178968,-3.072603178877));
#48908=CARTESIAN_POINT('Ctrl Pts',(1.715651325333,-3.173030747985,-3.118644845544));
#48909=CARTESIAN_POINT('Ctrl Pts',(0.3958289184352,-3.585373490323,-3.16468651221));
#48910=CARTESIAN_POINT('Ctrl Pts',(-0.9821576736188,-3.470871634321,-3.210728178877));
#48911=CARTESIAN_POINT('Ctrl Pts',(-2.215823327712,-2.846350396235,-3.256769845544));
#48912=CARTESIAN_POINT('Ctrl Pts',(-3.123889834539,-1.80357863689,-3.30281151221));
#48913=CARTESIAN_POINT('Ctrl Pts',(-3.572923415067,-0.4957840939792,-3.348853178877));
#48914=CARTESIAN_POINT('Ctrl Pts',(-3.496941845406,0.8848623212845,-3.394894845544));
#48915=CARTESIAN_POINT('Ctrl Pts',(-2.907110065457,2.135484644079,-3.44093651221));
#48916=CARTESIAN_POINT('Ctrl Pts',(-1.890099572078,3.072313005768,-3.486978178877));
#48917=CARTESIAN_POINT('Ctrl Pts',(-0.5953526720002,3.557687281609,-3.533019845544));
#48918=CARTESIAN_POINT('Ctrl Pts',(0.7868769799293,3.520285246431,-3.57906151221));
#48919=CARTESIAN_POINT('Ctrl Pts',(2.053480773757,2.965602857698,-3.625103178877));
#48920=CARTESIAN_POINT('Ctrl Pts',(3.018340479732,1.975146664475,-3.671144845544));
#48921=CARTESIAN_POINT('Ctrl Pts',(3.539676970626,0.6944570119162,-3.71718651221));
#48922=CARTESIAN_POINT('Ctrl Pts',(3.540883634913,-0.688278055575,-3.763228178877));
#48923=CARTESIAN_POINT('Ctrl Pts',(3.021783162038,-1.969875660898,-3.809269845544));
#48924=CARTESIAN_POINT('Ctrl Pts',(2.058653596917,-2.962014342585,-3.85531151221));
#48925=CARTESIAN_POINT('Ctrl Pts',(0.7930198351441,-3.518906526017,-3.901353178877));
#48926=CARTESIAN_POINT('Ctrl Pts',(-0.5891424326969,-3.558720948849,-3.947394845544));
#48927=CARTESIAN_POINT('Ctrl Pts',(-1.884734498254,-3.075607170766,-3.99343651221));
#48928=CARTESIAN_POINT('Ctrl Pts',(-2.903378515752,-2.140555253211,-4.039478178877));
#48929=CARTESIAN_POINT('Ctrl Pts',(-3.495392143951,-0.890964285359,-4.085519845544));
#48930=CARTESIAN_POINT('Ctrl Pts',(-3.573783279237,0.4895474142708,-4.13156151221));
#48931=CARTESIAN_POINT('Ctrl Pts',(-3.127032913541,1.798123676345,-4.177603178877));
#48932=CARTESIAN_POINT('Ctrl Pts',(-2.220787768898,2.842478721679,-4.223644845544));
#48933=CARTESIAN_POINT('Ctrl Pts',(-0.9882139884594,3.469152160271,-4.26968651221));
#48934=CARTESIAN_POINT('Ctrl Pts',(0.3895706616256,3.58605888079,-4.315728178877));
#48935=CARTESIAN_POINT('Ctrl Pts',(1.710110731203,3.176020290621,-4.361769845544));
#48936=CARTESIAN_POINT('Ctrl Pts',(2.779362449993,2.299288579191,-4.40781151221));
#48937=CARTESIAN_POINT('Ctrl Pts',(3.440207029409,1.084693119086,-4.453853178877));
#48938=CARTESIAN_POINT('Ctrl Pts',(3.595538206437,-0.2892901598772,-4.499894845544));
#48939=CARTESIAN_POINT('Ctrl Pts',(3.222531009545,-1.620764194701,-4.54593651221));
#48940=CARTESIAN_POINT('Ctrl Pts',(2.375996820758,-2.714079282501,-4.591978178877));
#48941=CARTESIAN_POINT('Ctrl Pts',(1.180325142345,-3.408577957331,-4.638019845544));
#48942=CARTESIAN_POINT('Ctrl Pts',(-0.1887792404969,-3.602218957155,-4.68406151221));
#48943=CARTESIAN_POINT('Ctrl Pts',(-1.530171890201,-3.26650979655,-4.730103178877));
#48944=CARTESIAN_POINT('Ctrl Pts',(-2.27446554662,-2.722785672557,-4.760797623321));
#48945=CARTESIAN_POINT('Ctrl Pts',(-2.581860640706,-2.390829167532,-4.776144845544));
#48946=CARTESIAN_POINT('',(-3.93911337870815,0.694572063117019,-1.60839731732686));
#48947=CARTESIAN_POINT('Ctrl Pts',(-3.9391476461815,0.694580681980914,-1.60831164028612));
#48948=CARTESIAN_POINT('Ctrl Pts',(-3.87575636899027,1.05329971993104,-1.61916055136511));
#48949=CARTESIAN_POINT('Ctrl Pts',(-3.76331552410144,1.40367728055008,-1.63004175976234));
#48950=CARTESIAN_POINT('Ctrl Pts',(-3.44908409131853,2.05768393665711,-1.65177420498472));
#48951=CARTESIAN_POINT('Ctrl Pts',(-3.24867678133451,2.36091786560673,-1.66242155380477));
#48952=CARTESIAN_POINT('Ctrl Pts',(-2.85427330231202,2.81251457419833,-1.68033258195991));
#48953=CARTESIAN_POINT('Ctrl Pts',(-2.68089218807246,2.97828559101128,-1.68755165834065));
#48954=CARTESIAN_POINT('Ctrl Pts',(-2.29199649028268,3.28815721323979,-1.70234773215377));
#48955=CARTESIAN_POINT('Ctrl Pts',(-2.07541513183239,3.42900620445079,-1.70993152711484));
#48956=CARTESIAN_POINT('Ctrl Pts',(-1.73246767296789,3.60753719420245,-1.72151186108472));
#48957=CARTESIAN_POINT('Ctrl Pts',(-1.6152980874153,3.66151208582675,-1.72539240561347));
#48958=CARTESIAN_POINT('Ctrl Pts',(-1.26155783509673,3.80419579142845,-1.73684399654552));
#48959=CARTESIAN_POINT('Ctrl Pts',(-1.01959031116382,3.87599732536495,-1.74426624699113));
#48960=CARTESIAN_POINT('Ctrl Pts',(-0.520819148694711,3.97409498843021,
-1.75936524951164));
#48961=CARTESIAN_POINT('Ctrl Pts',(-0.264781011431223,3.9992682257859,-1.76708259008009));
#48962=CARTESIAN_POINT('Ctrl Pts',(0.24893970914982,4.00053834585732,-1.78247105983387));
#48963=CARTESIAN_POINT('Ctrl Pts',(0.505470134302276,3.97626597241578,-1.79004184896571));
#48964=CARTESIAN_POINT('Ctrl Pts',(1.01240067258279,3.87819256282968,-1.8054348808173));
#48965=CARTESIAN_POINT('Ctrl Pts',(1.26150083420194,3.80449777615572,-1.81319367488307));
#48966=CARTESIAN_POINT('Ctrl Pts',(1.74342457165987,3.60956884353135,-1.82873460850295));
#48967=CARTESIAN_POINT('Ctrl Pts',(1.97457153864621,3.48830483716102,-1.83645395373821));
#48968=CARTESIAN_POINT('Ctrl Pts',(2.62992623847885,3.05858975308443,-1.85980733424332));
#48969=CARTESIAN_POINT('Ctrl Pts',(3.00637774151654,2.6901616353728,-1.87531400123001));
#48970=CARTESIAN_POINT('Ctrl Pts',(3.44781193210487,2.04384145685652,-1.89857824856414));
#48971=CARTESIAN_POINT('Ctrl Pts',(3.57243967653421,1.81757792873232,-1.90625597378683));
#48972=CARTESIAN_POINT('Ctrl Pts',(3.77617991548416,1.34412722685851,-1.92173915500655));
#48973=CARTESIAN_POINT('Ctrl Pts',(3.85474827892487,1.09817128411223,-1.92935993309336));
#48974=CARTESIAN_POINT('Ctrl Pts',(3.96319739898563,0.597574292783151,-1.94456013998803));
#48975=CARTESIAN_POINT('Ctrl Pts',(3.99320564673335,0.344047886583298,-1.95220040824628));
#48976=CARTESIAN_POINT('Ctrl Pts',(4.00458381732679,-0.162576490571243,
-1.96740990150124));
#48977=CARTESIAN_POINT('Ctrl Pts',(3.98641123253988,-0.413670763323244,
-1.97480775895236));
#48978=CARTESIAN_POINT('Ctrl Pts',(3.92319550876267,-0.790361327529153,
-1.98615799566182));
#48979=CARTESIAN_POINT('Ctrl Pts',(3.89526587387948,-0.9180352503498,-1.99006416710248));
#48980=CARTESIAN_POINT('Ctrl Pts',(3.79391229657841,-1.29288061633546,-2.00170958005469));
#48981=CARTESIAN_POINT('Ctrl Pts',(3.70261571485556,-1.53537175287446,-2.00945323725056));
#48982=CARTESIAN_POINT('Ctrl Pts',(3.47453219068466,-1.99840856444878,-2.02476565236659));
#48983=CARTESIAN_POINT('Ctrl Pts',(3.33842647584621,-2.21798524879933,-2.03243546445543));
#48984=CARTESIAN_POINT('Ctrl Pts',(2.86447884276471,-2.84079120359918,-2.05585926705293));
#48985=CARTESIAN_POINT('Ctrl Pts',(2.46970933926694,-3.18935455492974,-2.07121509202959));
#48986=CARTESIAN_POINT('Ctrl Pts',(1.79334333320813,-3.58483604994515,-2.09461011537361));
#48987=CARTESIAN_POINT('Ctrl Pts',(1.55647028382883,-3.69401257860335,-2.10241022000926));
#48988=CARTESIAN_POINT('Ctrl Pts',(1.06633238570733,-3.86369280979337,-2.11786329345988));
#48989=CARTESIAN_POINT('Ctrl Pts',(0.814729067481227,-3.92443178881597,
-2.12549294687453));
#48990=CARTESIAN_POINT('Ctrl Pts',(0.305940997637993,-3.99645945661362,
-2.14084188698538));
#48991=CARTESIAN_POINT('Ctrl Pts',(0.0497744729073863,-4.00787011059076,
-2.14855605117495));
#48992=CARTESIAN_POINT('Ctrl Pts',(-0.460511180924768,-3.98141866816329,
-2.16374520187095));
#48993=CARTESIAN_POINT('Ctrl Pts',(-0.713171682148684,-3.94404452875386,
-2.17125045661919));
#48994=CARTESIAN_POINT('Ctrl Pts',(-1.20616270496559,-3.82207313292113,
-2.1864759203107));
#48995=CARTESIAN_POINT('Ctrl Pts',(-1.44578608562418,-3.73812438180054,
-2.19409957806823));
#48996=CARTESIAN_POINT('Ctrl Pts',(-1.79243706317895,-3.57813833673693,
-2.20542588038207));
#48997=CARTESIAN_POINT('Ctrl Pts',(-1.90642404006754,-3.51871380126743,
-2.20922126752684));
#48998=CARTESIAN_POINT('Ctrl Pts',(-2.2318305682894,-3.32860139091786,-2.22042824021237));
#48999=CARTESIAN_POINT('Ctrl Pts',(-2.43459498834245,-3.18326446341512,
-2.22791388798638));
#49000=CARTESIAN_POINT('Ctrl Pts',(-2.81827082920698,-2.85037426083714,
-2.24312531473129));
#49001=CARTESIAN_POINT('Ctrl Pts',(-2.99678000710199,-2.66202820658115,
-2.25075054803303));
#49002=CARTESIAN_POINT('Ctrl Pts',(-3.31540162582115,-2.25250451580803,
-2.26622360816346));
#49003=CARTESIAN_POINT('Ctrl Pts',(-3.45476507159533,-2.03239459659418,
-2.27400186365226));
#49004=CARTESIAN_POINT('Ctrl Pts',(-3.80523178798918,-1.33796544403393,
-2.29725172660996));
#49005=CARTESIAN_POINT('Ctrl Pts',(-3.90874827153045,-0.910232814772706,
-2.31012052099671));
#49006=CARTESIAN_POINT('Ctrl Pts',(-3.98832494428433,-0.372437174862723,
-2.32636476587382));
#49007=CARTESIAN_POINT('Ctrl Pts',(-4.00260791525811,-0.158802003029431,
-2.33277805970415));
#49008=CARTESIAN_POINT('Ctrl Pts',(-3.99651941653082,0.269734882242017,
-2.34555535366208));
#49009=CARTESIAN_POINT('Ctrl Pts',(-3.97624197357851,0.483643897924661,
-2.35190371057797));
#49010=CARTESIAN_POINT('Ctrl Pts',(-3.93908532777216,0.694566072447258,
-2.35828102994364));
#49011=CARTESIAN_POINT('',(-3.48621875314954,0.61471493280625,-1.87404472598981));
#49012=CARTESIAN_POINT('Ctrl Pts',(-3.48611163489721,0.614695485491625,
-1.873914457161));
#49013=CARTESIAN_POINT('Ctrl Pts',(-3.45247823923436,0.804904617636081,
-1.880427867122));
#49014=CARTESIAN_POINT('Ctrl Pts',(-3.40329486078119,0.992351978567723,
-1.886941277084));
#49015=CARTESIAN_POINT('Ctrl Pts',(-3.33926661181778,1.17458628760328,-1.89345468704583));
#49016=CARTESIAN_POINT('Ctrl Pts',(-3.28724381166632,1.32265123070542,-1.89874681716394));
#49017=CARTESIAN_POINT('Ctrl Pts',(-3.22541325987337,1.46728788207019,-1.90403894728194));
#49018=CARTESIAN_POINT('Ctrl Pts',(-3.15416309562667,1.60712636907785,-1.90933107739992));
#49019=CARTESIAN_POINT('Ctrl Pts',(-3.13772049359028,1.63939729245812,-1.91055235724362));
#49020=CARTESIAN_POINT('Ctrl Pts',(-3.12077629297601,1.67141270174591,-1.91177363708731));
#49021=CARTESIAN_POINT('Ctrl Pts',(-3.10334122949876,1.70315880781664,-1.91299491693101));
#49022=CARTESIAN_POINT('Ctrl Pts',(-3.010355402605,1.87246922802227,-1.91950832689267));
#49023=CARTESIAN_POINT('Ctrl Pts',(-2.90342002496954,2.03409949917319,-1.92602173685433));
#49024=CARTESIAN_POINT('Ctrl Pts',(-2.78413804221371,2.18602098504228,-1.93253514681599));
#49025=CARTESIAN_POINT('Ctrl Pts',(-2.66485605945771,2.33794247091159,-1.93904855677766));
#49026=CARTESIAN_POINT('Ctrl Pts',(-2.53321256598554,2.48017394117643,-1.94556196673933));
#49027=CARTESIAN_POINT('Ctrl Pts',(-2.39079396961086,2.61067055624253,-1.952075376701));
#49028=CARTESIAN_POINT('Ctrl Pts',(-2.36676052640752,2.63269213956278,-1.95317452858396));
#49029=CARTESIAN_POINT('Ctrl Pts',(-2.34242073842935,2.65437904749335,-1.95427368046692));
#49030=CARTESIAN_POINT('Ctrl Pts',(-2.3177824805595,2.6757212808535,-1.95537283234988));
#49031=CARTESIAN_POINT('Ctrl Pts',(-2.19641810063612,2.78084993611871,-1.96078709042859));
#49032=CARTESIAN_POINT('Ctrl Pts',(-2.06781106235418,2.87761446755544,-1.96620134850729));
#49033=CARTESIAN_POINT('Ctrl Pts',(-1.93328280840194,2.96525962093555,-1.971615606586));
#49034=CARTESIAN_POINT('Ctrl Pts',(-1.7714438903673,3.07069767113915,-1.97812901654767));
#49035=CARTESIAN_POINT('Ctrl Pts',(-1.6010187810845,3.16295401534946,-1.98464242650933));
#49036=CARTESIAN_POINT('Ctrl Pts',(-1.42421971206299,3.24075297381787,-1.991155836471));
#49037=CARTESIAN_POINT('Ctrl Pts',(-1.33140030198562,3.28159738249964,-1.99457537297411));
#49038=CARTESIAN_POINT('Ctrl Pts',(-1.23682153800335,3.31845691336659,-1.99799490947721));
#49039=CARTESIAN_POINT('Ctrl Pts',(-1.14082056111593,3.35113838080967,-2.00141444598032));
#49040=CARTESIAN_POINT('Ctrl Pts',(-1.05396233511999,3.38070739538729,-2.00450831943888));
#49041=CARTESIAN_POINT('Ctrl Pts',(-0.965939942205691,3.40685628944164,
-2.00760219289745));
#49042=CARTESIAN_POINT('Ctrl Pts',(-0.877038495435007,3.42954597194126,
-2.01069606635601));
#49043=CARTESIAN_POINT('Ctrl Pts',(-0.689877780312868,3.47731366703263,
-2.01720947631767));
#49044=CARTESIAN_POINT('Ctrl Pts',(-0.498817901017613,3.50975420229228,
-2.02372288627933));
#49045=CARTESIAN_POINT('Ctrl Pts',(-0.306392768733605,3.52652952279029,
-2.03023629624099));
#49046=CARTESIAN_POINT('Ctrl Pts',(-0.136818383836607,3.54131275105748,
-2.03597622986983));
#49047=CARTESIAN_POINT('Ctrl Pts',(0.0338347226870868,3.54392884861796,
-2.04171616349867));
#49048=CARTESIAN_POINT('Ctrl Pts',(0.203776655436933,3.53413003081367,-2.0474560971275));
#49049=CARTESIAN_POINT('Ctrl Pts',(0.226676931195759,3.53280960550016,-2.04822957346034));
#49050=CARTESIAN_POINT('Ctrl Pts',(0.249564290458189,3.53126376392604,-2.04900304979317));
#49051=CARTESIAN_POINT('Ctrl Pts',(0.27243444834103,3.52949358819305,-2.049776526126));
#49052=CARTESIAN_POINT('Ctrl Pts',(0.46502303554917,3.51458701670047,-2.05628993608767));
#49053=CARTESIAN_POINT('Ctrl Pts',(0.656363625397378,3.4837751352979,-2.06280334604933));
#49054=CARTESIAN_POINT('Ctrl Pts',(0.843944386843304,3.43771235132368,-2.069316756011));
#49055=CARTESIAN_POINT('Ctrl Pts',(1.03152514828923,3.39164956734945,-2.07583016597267));
#49056=CARTESIAN_POINT('Ctrl Pts',(1.21536958570617,3.33033103466894,-2.08234357593433));
#49057=CARTESIAN_POINT('Ctrl Pts',(1.39297675817359,3.25438475836223,-2.088856985896));
#49058=CARTESIAN_POINT('Ctrl Pts',(1.43515898045606,3.23634729588709,-2.0904039397887));
#49059=CARTESIAN_POINT('Ctrl Pts',(1.47698836004088,3.2174850491827,-2.0919508936814));
#49060=CARTESIAN_POINT('Ctrl Pts',(1.5184303722474,3.19780693673633,-2.0934978475741));
#49061=CARTESIAN_POINT('Ctrl Pts',(1.65147889683793,3.13463085796226,-2.09846430364307));
#49062=CARTESIAN_POINT('Ctrl Pts',(1.78053424961026,3.06304474292021,-2.10343075971204));
#49063=CARTESIAN_POINT('Ctrl Pts',(1.90464785652295,2.98375084516111,-2.10839721578101));
#49064=CARTESIAN_POINT('Ctrl Pts',(2.06742042360426,2.87975844970031,-2.11491062574267));
#49065=CARTESIAN_POINT('Ctrl Pts',(2.22171376607907,2.76250122118534,-2.12142403570433));
#49066=CARTESIAN_POINT('Ctrl Pts',(2.36547392639545,2.63349262599518,-2.12793744566599));
#49067=CARTESIAN_POINT('Ctrl Pts',(2.45083123681511,2.55689402814848,-2.13180476992859));
#49068=CARTESIAN_POINT('Ctrl Pts',(2.53247769695781,2.47614836598736,-2.13567209419119));
#49069=CARTESIAN_POINT('Ctrl Pts',(2.609961772308,2.3915893349595,-2.1395394184538));
#49070=CARTESIAN_POINT('Ctrl Pts',(2.66297762765571,2.3337326807108,-2.14218550415286));
#49071=CARTESIAN_POINT('Ctrl Pts',(2.71404492982089,2.27409090047738,-2.14483158985192));
#49072=CARTESIAN_POINT('Ctrl Pts',(2.7630696354151,2.21281727982083,-2.14747767555098));
#49073=CARTESIAN_POINT('Ctrl Pts',(2.88374524539246,2.06199064132035,-2.15399108551267));
#49074=CARTESIAN_POINT('Ctrl Pts',(2.99204550459216,1.90128017903614,-2.16050449547437));
#49075=CARTESIAN_POINT('Ctrl Pts',(3.08664143368824,1.73287520944786,-2.16701790543607));
#49076=CARTESIAN_POINT('Ctrl Pts',(3.17650752923906,1.57289055436952,-2.17320564234583));
#49077=CARTESIAN_POINT('Ctrl Pts',(3.2540133932933,1.40594134449907,-2.17939337925558));
#49078=CARTESIAN_POINT('Ctrl Pts',(3.317978242801,1.23394504751905,-2.18558111616548));
#49079=CARTESIAN_POINT('Ctrl Pts',(3.32134484161676,1.22489253611342,-2.18590678921737));
#49080=CARTESIAN_POINT('Ctrl Pts',(3.32467393213607,1.21582604517722,-2.18623246226927));
#49081=CARTESIAN_POINT('Ctrl Pts',(3.32796545991406,1.20674589826919,-2.18655813532116));
#49082=CARTESIAN_POINT('Ctrl Pts',(3.39379549925573,1.02514438416957,-2.19307154528297));
#49083=CARTESIAN_POINT('Ctrl Pts',(3.4445898638602,0.838110253654046,-2.19958495524494));
#49084=CARTESIAN_POINT('Ctrl Pts',(3.47993533170847,0.648217911398604,-2.20609836520674));
#49085=CARTESIAN_POINT('Ctrl Pts',(3.51528079955726,0.458325569140407,-2.21261177516864));
#49086=CARTESIAN_POINT('Ctrl Pts',(3.53518366555639,0.265551810365206,-2.21912518513037));
#49087=CARTESIAN_POINT('Ctrl Pts',(3.53921587207989,0.0724312289064312,
-2.22563859509208));
#49088=CARTESIAN_POINT('Ctrl Pts',(3.5404507477039,0.0132874580830817,-2.22763334688469));
#49089=CARTESIAN_POINT('Ctrl Pts',(3.54019686595504,-0.0458877048812477,
-2.22962809867729));
#49090=CARTESIAN_POINT('Ctrl Pts',(3.53844190482233,-0.105018504061302,
-2.2316228504699));
#49091=CARTESIAN_POINT('Ctrl Pts',(3.53446643805599,-0.238965930375457,
-2.2361415086389));
#49092=CARTESIAN_POINT('Ctrl Pts',(3.52278756542149,-0.372685587266579,
-2.24066016680791));
#49093=CARTESIAN_POINT('Ctrl Pts',(3.50360264434659,-0.505307275679988,
-2.24517882497692));
#49094=CARTESIAN_POINT('Ctrl Pts',(3.47594858170895,-0.69647451917164,-2.25169223493864));
#49095=CARTESIAN_POINT('Ctrl Pts',(3.43270056047567,-0.885379751350099,
-2.25820564490037));
#49096=CARTESIAN_POINT('Ctrl Pts',(3.37442090167997,-1.06953540954889,-2.26471905486209));
#49097=CARTESIAN_POINT('Ctrl Pts',(3.33581079605796,-1.19153800120563,-2.26903417014895));
#49098=CARTESIAN_POINT('Ctrl Pts',(3.29059905133193,-1.31146265306598,-2.2733492854358));
#49099=CARTESIAN_POINT('Ctrl Pts',(3.23895722418867,-1.42855034908728,-2.27766440072265));
#49100=CARTESIAN_POINT('Ctrl Pts',(3.21264878372798,-1.48819956852543,-2.27986269539743));
#49101=CARTESIAN_POINT('Ctrl Pts',(3.18467168469657,-1.54711255044106,-2.28206099007222));
#49102=CARTESIAN_POINT('Ctrl Pts',(3.15508456246594,-1.60520476755959,-2.284259284747));
#49103=CARTESIAN_POINT('Ctrl Pts',(3.06741976534675,-1.77732838229316,-2.29077269470864));
#49104=CARTESIAN_POINT('Ctrl Pts',(2.96562690748143,-1.94223957070431,-2.29728610467027));
#49105=CARTESIAN_POINT('Ctrl Pts',(2.85118122343503,-2.0978372735158,-2.30379951463191));
#49106=CARTESIAN_POINT('Ctrl Pts',(2.73673553938697,-2.25343497632954,-2.31031292459364));
#49107=CARTESIAN_POINT('Ctrl Pts',(2.60962088951851,-2.39973705663602,-2.31682633455537));
#49108=CARTESIAN_POINT('Ctrl Pts',(2.47132239430563,-2.53459348728904,-2.32333974451709));
#49109=CARTESIAN_POINT('Ctrl Pts',(2.4687292831959,-2.53712205933177,-2.32346187162851));
#49110=CARTESIAN_POINT('Ctrl Pts',(2.46613224843455,-2.5396465996386,-2.32358399873993));
#49111=CARTESIAN_POINT('Ctrl Pts',(2.463531299937,-2.54216709408167,-2.32370612585135));
#49112=CARTESIAN_POINT('Ctrl Pts',(2.32741576151579,-2.67407222735452,-2.33009740870157));
#49113=CARTESIAN_POINT('Ctrl Pts',(2.18058121321383,-2.79489605595183,-2.33648869155178));
#49114=CARTESIAN_POINT('Ctrl Pts',(2.02510726029512,-2.90329545916035,-2.342879974402));
#49115=CARTESIAN_POINT('Ctrl Pts',(1.8666624507869,-3.01376620020569,-2.34939338436364));
#49116=CARTESIAN_POINT('Ctrl Pts',(1.69922697758555,-3.11134926906942,-2.35590679432527));
#49117=CARTESIAN_POINT('Ctrl Pts',(1.52494467780377,-3.19463871795646,-2.36242020428691));
#49118=CARTESIAN_POINT('Ctrl Pts',(1.45958838442203,-3.22587246724644,-2.36486274912882));
#49119=CARTESIAN_POINT('Ctrl Pts',(1.39326974838671,-3.25509547106922,-2.36730529397073));
#49120=CARTESIAN_POINT('Ctrl Pts',(1.32610734069228,-3.28223084516667,-2.36974783881264));
#49121=CARTESIAN_POINT('Ctrl Pts',(1.21417117552754,-3.32745599151041,-2.37381870393245));
#49122=CARTESIAN_POINT('Ctrl Pts',(1.09989117051022,-3.3668818964363,-2.37788956905227));
#49123=CARTESIAN_POINT('Ctrl Pts',(0.983909678540035,-3.40038425065325,
-2.38196043417208));
#49124=CARTESIAN_POINT('Ctrl Pts',(0.7983385571865,-3.45398822948136,-2.3884738441337));
#49125=CARTESIAN_POINT('Ctrl Pts',(0.608398132847113,-3.49243632959352,
-2.3949872540953));
#49126=CARTESIAN_POINT('Ctrl Pts',(0.416593020999056,-3.51524584577225,
-2.40150066405692));
#49127=CARTESIAN_POINT('Ctrl Pts',(0.276336123570181,-3.53192523424243,
-2.40626357503514));
#49128=CARTESIAN_POINT('Ctrl Pts',(0.135071043364323,-3.54024113541699,
-2.41102648601336));
#49129=CARTESIAN_POINT('Ctrl Pts',(-0.00617846241521584,-3.539994608273,
-2.41578939699159));
#49130=CARTESIAN_POINT('Ctrl Pts',(-0.0580914873316,-3.53990400286027,-2.41753989597509));
#49131=CARTESIAN_POINT('Ctrl Pts',(-0.110002393163228,-3.53865692860149,
-2.41929039495859));
#49132=CARTESIAN_POINT('Ctrl Pts',(-0.161860370969656,-3.53626328586113,
-2.4210408939421));
#49133=CARTESIAN_POINT('Ctrl Pts',(-0.354818077553921,-3.52735681026954,
-2.42755430390373));
#49134=CARTESIAN_POINT('Ctrl Pts',(-0.547027243948119,-3.50257873337156,
-2.43406771386537));
#49135=CARTESIAN_POINT('Ctrl Pts',(-0.73596390415267,-3.46243784695285,
-2.440581123827));
#49136=CARTESIAN_POINT('Ctrl Pts',(-0.924900564357221,-3.42229696053415,
-2.44709453378864));
#49137=CARTESIAN_POINT('Ctrl Pts',(-1.11058788540349,-3.36678693880149,
-2.45360794375027));
#49138=CARTESIAN_POINT('Ctrl Pts',(-1.29047199844307,-3.29639980380972,
-2.46012135371191));
#49139=CARTESIAN_POINT('Ctrl Pts',(-1.30621201758925,-3.29024086718272,
-2.46069128285001));
#49140=CARTESIAN_POINT('Ctrl Pts',(-1.32190738964502,-3.28396810707535,
-2.46126121198811));
#49141=CARTESIAN_POINT('Ctrl Pts',(-1.33755638533705,-3.27758187022733,
-2.46183114112621));
#49142=CARTESIAN_POINT('Ctrl Pts',(-1.5007512451651,-3.21098328155419,-2.46777462194984));
#49143=CARTESIAN_POINT('Ctrl Pts',(-1.65890194128621,-3.13204291772606,
-2.47371810277347));
#49144=CARTESIAN_POINT('Ctrl Pts',(-1.81033770201859,-3.04186253180114,
-2.47966158359708));
#49145=CARTESIAN_POINT('Ctrl Pts',(-1.97629486109295,-2.94303461572669,
-2.4861749935587));
#49146=CARTESIAN_POINT('Ctrl Pts',(-2.13420984660948,-2.83069876261338,
-2.4926884035203));
#49147=CARTESIAN_POINT('Ctrl Pts',(-2.28193901730622,-2.70625136015001,
-2.49920181348192));
#49148=CARTESIAN_POINT('Ctrl Pts',(-2.34749402191622,-2.65102766936699,
-2.50209214731408));
#49149=CARTESIAN_POINT('Ctrl Pts',(-2.41104305301027,-2.593418363129,-2.50498248114623));
#49150=CARTESIAN_POINT('Ctrl Pts',(-2.47239011042567,-2.53355227731117,
-2.50787281497841));
#49151=CARTESIAN_POINT('Ctrl Pts',(-2.54928955258278,-2.45850925491567,
-2.51149589110799));
#49152=CARTESIAN_POINT('Ctrl Pts',(-2.62272889170948,-2.37992008874756,
-2.5151189672376));
#49153=CARTESIAN_POINT('Ctrl Pts',(-2.69244525650513,-2.29816470206638,
-2.51874204336726));
#49154=CARTESIAN_POINT('Ctrl Pts',(-2.81777832948228,-2.15118839492212,
-2.52525545332906));
#49155=CARTESIAN_POINT('Ctrl Pts',(-2.93108910381199,-1.9939736040557,-2.53176886329103));
#49156=CARTESIAN_POINT('Ctrl Pts',(-3.03092976256236,-1.82862245583661,
-2.53828227325283));
#49157=CARTESIAN_POINT('Ctrl Pts',(-3.11080203430125,-1.69634196001263,
-2.54349298456952));
#49158=CARTESIAN_POINT('Ctrl Pts',(-3.18205838653695,-1.55884051299148,
-2.5487036958861));
#49159=CARTESIAN_POINT('Ctrl Pts',(-3.2439240626505,-1.41723557525112,-2.55391440720265));
#49160=CARTESIAN_POINT('Ctrl Pts',(-3.25939072882222,-1.38183377512727,
-2.55521710584774));
#49161=CARTESIAN_POINT('Ctrl Pts',(-3.27427051474745,-1.34617553341453,
-2.55651980449282));
#49162=CARTESIAN_POINT('Ctrl Pts',(-3.28855875162332,-1.31028157168752,
-2.55782250313791));
#49163=CARTESIAN_POINT('Ctrl Pts',(-3.35999902275125,-1.13081405726206,
-2.56433591309964));
#49164=CARTESIAN_POINT('Ctrl Pts',(-3.41664396289098,-0.9454748130943,-2.57084932306137));
#49165=CARTESIAN_POINT('Ctrl Pts',(-3.45794355355989,-0.756788175000208,
-2.57736273302309));
#49166=CARTESIAN_POINT('Ctrl Pts',(-3.49924314422819,-0.568101536908852,
-2.58387614298473));
#49167=CARTESIAN_POINT('Ctrl Pts',(-3.52520219045534,-0.376044002607325,
-2.59038955294637));
#49168=CARTESIAN_POINT('Ctrl Pts',(-3.53524656047543,-0.183140996775934,
-2.596902962908));
#49169=CARTESIAN_POINT('Ctrl Pts',(-3.5368160129307,-0.152999524933752,
-2.5979206959501));
#49170=CARTESIAN_POINT('Ctrl Pts',(-3.53799685819296,-0.122838037839204,
-2.5989384289922));
#49171=CARTESIAN_POINT('Ctrl Pts',(-3.53878693041333,-0.0926663970097817,
-2.5999561620343));
#49172=CARTESIAN_POINT('Ctrl Pts',(-3.54305325712833,0.070258047094353,
-2.60545183895384));
#49173=CARTESIAN_POINT('Ctrl Pts',(-3.5359238682156,0.233478412978716,-2.61094751587337));
#49174=CARTESIAN_POINT('Ctrl Pts',(-3.51766563120604,0.395426864888091,
-2.61644319279291));
#49175=CARTESIAN_POINT('Ctrl Pts',(-3.4960261890476,0.587366215653757,-2.62295660275464));
#49176=CARTESIAN_POINT('Ctrl Pts',(-3.4587560775586,0.777542371198995,-2.62947001271637));
#49177=CARTESIAN_POINT('Ctrl Pts',(-3.40627360153106,0.963435501424812,
-2.63598342267808));
#49178=CARTESIAN_POINT('Ctrl Pts',(-3.3793763475951,1.05870567743576,-2.63932154341837));
#49179=CARTESIAN_POINT('Ctrl Pts',(-3.34848198131686,1.15285246353695,-2.64265966415865));
#49180=CARTESIAN_POINT('Ctrl Pts',(-3.313650756516,1.24551943535272,-2.64599778489894));
#49181=CARTESIAN_POINT('Ctrl Pts',(-3.28051857787996,1.33366616810227,-2.64917307412027));
#49182=CARTESIAN_POINT('Ctrl Pts',(-3.24382428725794,1.42047390410623,-2.65234836334159));
#49183=CARTESIAN_POINT('Ctrl Pts',(-3.20373088991644,1.50567764427224,-2.65552365256292));
#49184=CARTESIAN_POINT('Ctrl Pts',(-3.12148807187998,1.68045444452225,-2.66203706252464));
#49185=CARTESIAN_POINT('Ctrl Pts',(-3.02494376338762,1.84848829715205,-2.66855047248637));
#49186=CARTESIAN_POINT('Ctrl Pts',(-2.91544434228993,2.0076070020078,-2.67506388244809));
#49187=CARTESIAN_POINT('Ctrl Pts',(-2.82031689157503,2.14584112783464,-2.68072239715903));
#49188=CARTESIAN_POINT('Ctrl Pts',(-2.7153993256723,2.27735955487245,-2.68638091186997));
#49189=CARTESIAN_POINT('Ctrl Pts',(-2.601597666831,2.400685231333,-2.69203942658091));
#49190=CARTESIAN_POINT('Ctrl Pts',(-2.58440437448575,2.41931742378652,-2.6928943218316));
#49191=CARTESIAN_POINT('Ctrl Pts',(-2.5670083197053,2.43776262618973,-2.6937492170823));
#49192=CARTESIAN_POINT('Ctrl Pts',(-2.54941430867889,2.4560172922504,-2.694604112333));
#49193=CARTESIAN_POINT('Ctrl Pts',(-2.41536629918196,2.59509880389615,-2.70111752229464));
#49194=CARTESIAN_POINT('Ctrl Pts',(-2.26984684389257,2.72310064051428,-2.70763093225627));
#49195=CARTESIAN_POINT('Ctrl Pts',(-2.11495442977927,2.83849845023986,-2.71414434221791));
#49196=CARTESIAN_POINT('Ctrl Pts',(-1.96006201566371,2.95389625996712,-2.72065775217964));
#49197=CARTESIAN_POINT('Ctrl Pts',(-1.79577783391285,3.05670494108783,-2.72717116214137));
#49198=CARTESIAN_POINT('Ctrl Pts',(-1.62417584367481,3.14538952674968,-2.73368457210309));
#49199=CARTESIAN_POINT('Ctrl Pts',(-1.5855649121518,3.16534380851171,-2.73515010770478));
#49200=CARTESIAN_POINT('Ctrl Pts',(-1.54658437024401,3.18458250627967,-2.73661564330646));
#49201=CARTESIAN_POINT('Ctrl Pts',(-1.50725869214041,3.20308776572967,-2.73808117890815));
#49202=CARTESIAN_POINT('Ctrl Pts',(-1.37180576833643,3.26682707345756,-2.7431290532681));
#49203=CARTESIAN_POINT('Ctrl Pts',(-1.23225792299338,3.32186406534164,-2.74817692762805));
#49204=CARTESIAN_POINT('Ctrl Pts',(-1.08981621794126,3.36789750679959,-2.753224801988));
#49205=CARTESIAN_POINT('Ctrl Pts',(-0.90601980097821,3.42729571182215,-2.75973821194964));
#49206=CARTESIAN_POINT('Ctrl Pts',(-0.717386036659192,3.47171455680863,
-2.76625162191127));
#49207=CARTESIAN_POINT('Ctrl Pts',(-0.526388358542247,3.50052703129853,
-2.77276503187291));
#49208=CARTESIAN_POINT('Ctrl Pts',(-0.415371292863036,3.51727423160149,
-2.77655093999826));
#49209=CARTESIAN_POINT('Ctrl Pts',(-0.303551189065533,3.52874803372401,
-2.78033684812361));
#49210=CARTESIAN_POINT('Ctrl Pts',(-0.191438997966164,3.5348198129545,-2.78412275624896));
#49211=CARTESIAN_POINT('Ctrl Pts',(-0.110669418520737,3.53919413701438,
-2.78685025808534));
#49212=CARTESIAN_POINT('Ctrl Pts',(-0.0297482761444177,3.54076478310675,
-2.78957775992171));
#49213=CARTESIAN_POINT('Ctrl Pts',(0.0511292772991568,3.53955874091815,
-2.79230526175808));
#49214=CARTESIAN_POINT('Ctrl Pts',(0.244268895115812,3.53667865222285,-2.7988186717197));
#49215=CARTESIAN_POINT('Ctrl Pts',(0.437158914978994,3.51796689039577,-2.8053320816813));
#49216=CARTESIAN_POINT('Ctrl Pts',(0.627264950562928,3.48378569015157,-2.81184549164292));
#49217=CARTESIAN_POINT('Ctrl Pts',(0.805489255928714,3.45174083344104,-2.81795180995316));
#49218=CARTESIAN_POINT('Ctrl Pts',(0.981286782970914,3.40609307546753,-2.8240581282634));
#49219=CARTESIAN_POINT('Ctrl Pts',(1.15251126677808,3.3471357576215,-2.83016444657365));
#49220=CARTESIAN_POINT('Ctrl Pts',(1.16392633791351,3.34320523342191,-2.83057153822513));
#49221=CARTESIAN_POINT('Ctrl Pts',(1.1753210843407,3.33921555889236,-2.83097862987661));
#49222=CARTESIAN_POINT('Ctrl Pts',(1.18669494970798,3.33516705334005,-2.83138572152809));
#49223=CARTESIAN_POINT('Ctrl Pts',(1.36867521807276,3.27039152601533,-2.83789913148973));
#49224=CARTESIAN_POINT('Ctrl Pts',(1.54528068641558,3.19056603871398,-2.84441254145137));
#49225=CARTESIAN_POINT('Ctrl Pts',(1.7142617758279,3.09700442209031,-2.850925951413));
#49226=CARTESIAN_POINT('Ctrl Pts',(1.88324286524021,3.00344280546664,-2.85743936137464));
#49227=CARTESIAN_POINT('Ctrl Pts',(2.04462139391706,2.89613498241052,-2.86395277133627));
#49228=CARTESIAN_POINT('Ctrl Pts',(2.19616581212668,2.77635948507303,-2.87046618129807));
#49229=CARTESIAN_POINT('Ctrl Pts',(2.24068245442155,2.74117506169632,-2.87237951565123));
#49230=CARTESIAN_POINT('Ctrl Pts',(2.28434948110076,2.70491536505777,-2.8742928500044));
#49231=CARTESIAN_POINT('Ctrl Pts',(2.32710837011083,2.667614408748,-2.87620618435757));
#49232=CARTESIAN_POINT('Ctrl Pts',(2.42991012144495,2.57793472520482,-2.88080625996636));
#49233=CARTESIAN_POINT('Ctrl Pts',(2.52746203568147,2.4822357996935,-2.88540633557519));
#49234=CARTESIAN_POINT('Ctrl Pts',(2.61918727517748,2.38126086742591,-2.89000641118393));
#49235=CARTESIAN_POINT('Ctrl Pts',(2.74906429014366,2.2382868848952,-2.89651982114573));
#49236=CARTESIAN_POINT('Ctrl Pts',(2.8672760376804,2.08472396627836,-2.90303323110736));
#49237=CARTESIAN_POINT('Ctrl Pts',(2.97225682514692,1.92258536488254,-2.909546641069));
#49238=CARTESIAN_POINT('Ctrl Pts',(3.04049404589932,1.8171957235688,-2.91378033948305));
#49239=CARTESIAN_POINT('Ctrl Pts',(3.10314345866287,1.70817591623019,-2.9180140378971));
#49240=CARTESIAN_POINT('Ctrl Pts',(3.15975379732033,1.59610649404042,-2.92224773631116));
#49241=CARTESIAN_POINT('Ctrl Pts',(3.19023665890577,1.53576068503121,-2.92452744785874));
#49242=CARTESIAN_POINT('Ctrl Pts',(3.21896862084254,1.47453073235579,-2.92680715940632));
#49243=CARTESIAN_POINT('Ctrl Pts',(3.24591833613534,1.41252706412557,-2.92908687095391));
#49244=CARTESIAN_POINT('Ctrl Pts',(3.32291691266136,1.23537512981941,-2.93560028091564));
#49245=CARTESIAN_POINT('Ctrl Pts',(3.38536604105094,1.05191544335807,-2.94211369087737));
#49246=CARTESIAN_POINT('Ctrl Pts',(3.43257863439251,0.864620338177981,-2.94862710083908));
#49247=CARTESIAN_POINT('Ctrl Pts',(3.47979122773339,0.677325233000614,-2.9551405108007));
#49248=CARTESIAN_POINT('Ctrl Pts',(3.51177061081401,0.486170850953884,-2.9616539207623));
#49249=CARTESIAN_POINT('Ctrl Pts',(3.52779770972739,0.293671846368202,-2.96816733072392));
#49250=CARTESIAN_POINT('Ctrl Pts',(3.54382480864101,0.101172841779726,-2.97468074068564));
#49251=CARTESIAN_POINT('Ctrl Pts',(3.54389063706576,-0.0926387220615205,
-2.98119415064737));
#49252=CARTESIAN_POINT('Ctrl Pts',(3.52829370107045,-0.285162093399601,
-2.98770756060909));
#49253=CARTESIAN_POINT('Ctrl Pts',(3.51269676507538,-0.477685464734896,
-2.99422097057073));
#49254=CARTESIAN_POINT('Ctrl Pts',(3.48143795907187,-0.668944729192209,
-3.00073438053237));
#49255=CARTESIAN_POINT('Ctrl Pts',(3.43479147403378,-0.856389724647762,
-3.007247790494));
#49256=CARTESIAN_POINT('Ctrl Pts',(3.41788200033896,-0.92433902923723,-3.00960891876165));
#49257=CARTESIAN_POINT('Ctrl Pts',(3.39895032352512,-0.991786185528306,
-3.0119700470293));
#49258=CARTESIAN_POINT('Ctrl Pts',(3.37801076294783,-1.05860440458627,-3.01433117529694));
#49259=CARTESIAN_POINT('Ctrl Pts',(3.34118643821438,-1.17611096770731,-3.01848345699093));
#49260=CARTESIAN_POINT('Ctrl Pts',(3.29815197932209,-1.29167222505131,-3.02263573868492));
#49261=CARTESIAN_POINT('Ctrl Pts',(3.24923804098228,-1.40467798594993,-3.02678802037891));
#49262=CARTESIAN_POINT('Ctrl Pts',(3.17250997753916,-1.58194265704288,-3.03330143034064));
#49263=CARTESIAN_POINT('Ctrl Pts',(3.08131256433646,-1.75293573710948,-3.03981484030237));
#49264=CARTESIAN_POINT('Ctrl Pts',(2.97686209402276,-1.91541538362641,-3.04632825026408));
#49265=CARTESIAN_POINT('Ctrl Pts',(2.90178864237797,-2.0321971257231,-3.05100974347646));
#49266=CARTESIAN_POINT('Ctrl Pts',(2.81986112148126,-2.14458818654409,-3.05569123668883));
#49267=CARTESIAN_POINT('Ctrl Pts',(2.73155102519233,-2.25171689978334,-3.06037272990121));
#49268=CARTESIAN_POINT('Ctrl Pts',(2.69699437047138,-2.2936374740968,-3.06220464665044));
#49269=CARTESIAN_POINT('Ctrl Pts',(2.66146049390564,-2.33475232045301,-3.06403656339968));
#49270=CARTESIAN_POINT('Ctrl Pts',(2.6249951611146,-2.37502361902699,-3.06586848014892));
#49271=CARTESIAN_POINT('Ctrl Pts',(2.49534207400957,-2.51820887971733,-3.07238189011064));
#49272=CARTESIAN_POINT('Ctrl Pts',(2.35392512391004,-2.65072077167275,-3.07889530007237));
#49273=CARTESIAN_POINT('Ctrl Pts',(2.20273828215036,-2.77093269463368,-3.08540871003409));
#49274=CARTESIAN_POINT('Ctrl Pts',(2.05155144039287,-2.89114461759288,-3.09192211999573));
#49275=CARTESIAN_POINT('Ctrl Pts',(1.89057497031891,-2.9990702680108,-3.09843552995737));
#49276=CARTESIAN_POINT('Ctrl Pts',(1.7218118521876,-3.09304726818777,-3.104948939919));
#49277=CARTESIAN_POINT('Ctrl Pts',(1.70915449898499,-3.10009560965795,-3.10543745027216));
#49278=CARTESIAN_POINT('Ctrl Pts',(1.69645349524291,-3.10706540362333,-3.10592596062531));
#49279=CARTESIAN_POINT('Ctrl Pts',(1.68370970010857,-3.11395594794783,-3.10641447097847));
#49280=CARTESIAN_POINT('Ctrl Pts',(1.52653782888907,-3.19893846169562,-3.11243937058695));
#49281=CARTESIAN_POINT('Ctrl Pts',(1.36285678345318,-3.2718654745696,-3.11846427019543));
#49282=CARTESIAN_POINT('Ctrl Pts',(1.19465624061227,-3.33212144593867,-3.12448916980391));
#49283=CARTESIAN_POINT('Ctrl Pts',(1.01281767690137,-3.39726308640959,-3.13100257976564));
#49284=CARTESIAN_POINT('Ctrl Pts',(0.825675827052175,-3.44760704052864,
-3.13751598972737));
#49285=CARTESIAN_POINT('Ctrl Pts',(0.635671099317594,-3.48238259226642,
-3.1440293996891));
#49286=CARTESIAN_POINT('Ctrl Pts',(0.553731273711291,-3.49737960143946,
-3.14683831756567));
#49287=CARTESIAN_POINT('Ctrl Pts',(0.471258885802527,-3.50948064073937,
-3.14964723544223));
#49288=CARTESIAN_POINT('Ctrl Pts',(0.38845946126229,-3.51862178231117,-3.15245615331881));
#49289=CARTESIAN_POINT('Ctrl Pts',(0.279260892156459,-3.53067741657646,
-3.15616064540387));
#49290=CARTESIAN_POINT('Ctrl Pts',(0.169493539234521,-3.53758465049955,
-3.15986513748894));
#49291=CARTESIAN_POINT('Ctrl Pts',(0.059649471939911,-3.53938415619341,
-3.163569629574));
#49292=CARTESIAN_POINT('Ctrl Pts',(-0.133483466588335,-3.54254813064478,
-3.17008303953564));
#49293=CARTESIAN_POINT('Ctrl Pts',(-0.326865118477281,-3.52992630187154,
-3.17659644949727));
#49294=CARTESIAN_POINT('Ctrl Pts',(-0.517952514192366,-3.50173373138306,
-3.18310985945891));
#49295=CARTESIAN_POINT('Ctrl Pts',(-0.668433322988736,-3.47953215815382,
-3.18823915223817));
#49296=CARTESIAN_POINT('Ctrl Pts',(-0.817504437674782,-3.44766956351041,
-3.19336844501743));
#49297=CARTESIAN_POINT('Ctrl Pts',(-0.963872074523706,-3.4062516970935,
-3.19849773779676));
#49298=CARTESIAN_POINT('Ctrl Pts',(-1.00336874001705,-3.39507526731343,
-3.19988185497925));
#49299=CARTESIAN_POINT('Ctrl Pts',(-1.04266855713235,-3.38320312817922,
-3.20126597216175));
#49300=CARTESIAN_POINT('Ctrl Pts',(-1.0817487466423,-3.37064673995017,-3.20265008934425));
#49301=CARTESIAN_POINT('Ctrl Pts',(-1.26565318687387,-3.31155860405448,
-3.20916349930603));
#49302=CARTESIAN_POINT('Ctrl Pts',(-1.4446743658271,-3.23732575217221,-3.21567690926797));
#49303=CARTESIAN_POINT('Ctrl Pts',(-1.61651402611654,-3.14912462305492,
-3.22219031922975));
#49304=CARTESIAN_POINT('Ctrl Pts',(-1.78835368640846,-3.06092349393635,
-3.22870372919164));
#49305=CARTESIAN_POINT('Ctrl Pts',(-1.95303292882817,-2.95874267186129,
-3.23521713915337));
#49306=CARTESIAN_POINT('Ctrl Pts',(-2.10823418017326,-2.84374236629767,
-3.2417305491151));
#49307=CARTESIAN_POINT('Ctrl Pts',(-2.13054463355673,-2.8272108697142,-3.24266686327532));
#49308=CARTESIAN_POINT('Ctrl Pts',(-2.15265877543496,-2.81041477835907,
-3.24360317743554));
#49309=CARTESIAN_POINT('Ctrl Pts',(-2.17456960835048,-2.79335766031483,
-3.24453949159576));
#49310=CARTESIAN_POINT('Ctrl Pts',(-2.30508009238466,-2.69175802050364,
-3.25011658739717));
#49311=CARTESIAN_POINT('Ctrl Pts',(-2.42837651672354,-2.58089661856788,
-3.25569368319859));
#49312=CARTESIAN_POINT('Ctrl Pts',(-2.5433709048767,-2.46202800977271,-3.261270779));
#49313=CARTESIAN_POINT('Ctrl Pts',(-2.67767119664131,-2.3232030714498,-3.26778418896164));
#49314=CARTESIAN_POINT('Ctrl Pts',(-2.80066707596171,-2.17344287527037,
-3.27429759892327));
#49315=CARTESIAN_POINT('Ctrl Pts',(-2.91067619386607,-2.01467029405205,
-3.28081100888491));
#49316=CARTESIAN_POINT('Ctrl Pts',(-2.96568075281904,-1.93528400344175,
-3.28406771386577));
#49317=CARTESIAN_POINT('Ctrl Pts',(-3.01743874035383,-1.85364279298029,
-3.28732441884663));
#49318=CARTESIAN_POINT('Ctrl Pts',(-3.06572992939683,-1.76999999999985,
-3.2905811238275));
#49319=CARTESIAN_POINT('Ctrl Pts',(-3.11402111843984,-1.6863572070194,-3.29383782880836));
#49320=CARTESIAN_POINT('Ctrl Pts',(-3.15884548692774,-1.60071286973475,
-3.29709453378923));
#49321=CARTESIAN_POINT('Ctrl Pts',(-3.20009375183195,-1.51338437905234,
-3.30035123877009));
#49322=CARTESIAN_POINT('Ctrl Pts',(-3.28259028163917,-1.33872739769007,
-3.30686464873173));
#49323=CARTESIAN_POINT('Ctrl Pts',(-3.350788476346,-1.15732974354807,-3.31337805869336));
#49324=CARTESIAN_POINT('Ctrl Pts',(-3.40386425373005,-0.971609809982892,
-3.319891468655));
#49325=CARTESIAN_POINT('Ctrl Pts',(-3.44931029458254,-0.812587444152017,
-3.32546856445642));
#49326=CARTESIAN_POINT('Ctrl Pts',(-3.48367087278858,-0.650378907510944,
-3.33104566025783));
#49327=CARTESIAN_POINT('Ctrl Pts',(-3.50640349986333,-0.486553692971483,
-3.33662275605925));
#49328=CARTESIAN_POINT('Ctrl Pts',(-3.51021998094721,-0.45904979602653,
-3.33755907021947));
#49329=CARTESIAN_POINT('Ctrl Pts',(-3.51370875180592,-0.431500341699595,
-3.33849538437969));
#49330=CARTESIAN_POINT('Ctrl Pts',(-3.51687022111804,-0.4039131740079,-3.33943169853991));
#49331=CARTESIAN_POINT('Ctrl Pts',(-3.53886278150659,-0.21200479486206,
-3.34594510850164));
#49332=CARTESIAN_POINT('Ctrl Pts',(-3.54501434799336,-0.018297976412778,
-3.35245851846337));
#49333=CARTESIAN_POINT('Ctrl Pts',(-3.53547893630661,0.174620099336988,
-3.35897192842508));
#49334=CARTESIAN_POINT('Ctrl Pts',(-3.52594352461999,0.367538175083959,
-3.3654853383867));
#49335=CARTESIAN_POINT('Ctrl Pts',(-3.50072047066892,0.559691489813732,
-3.3719987483483));
#49336=CARTESIAN_POINT('Ctrl Pts',(-3.45994007730116,0.748501474870884,
-3.37851215830992));
#49337=CARTESIAN_POINT('Ctrl Pts',(-3.45127413373233,0.788624105885788,
-3.37989627549239));
#49338=CARTESIAN_POINT('Ctrl Pts',(-3.44190579926218,0.828594815438887,
-3.38128039267486));
#49339=CARTESIAN_POINT('Ctrl Pts',(-3.43183653862866,0.868388146010993,
-3.38266450985732));
#49340=CARTESIAN_POINT('Ctrl Pts',(-3.39452164469186,1.01585517102254,-3.38779380263658));
#49341=CARTESIAN_POINT('Ctrl Pts',(-3.34757990374054,1.16088584063295,-3.39292309541584));
#49342=CARTESIAN_POINT('Ctrl Pts',(-3.2915666257629,1.30230683044729,-3.3980523881951));
#49343=CARTESIAN_POINT('Ctrl Pts',(-3.22043841014641,1.48188965472389,-3.40456579815673));
#49344=CARTESIAN_POINT('Ctrl Pts',(-3.13467840856183,1.65567399227211,-3.41107920811837));
#49345=CARTESIAN_POINT('Ctrl Pts',(-3.03537185704593,1.82135003611944,-3.41759261808));
#49346=CARTESIAN_POINT('Ctrl Pts',(-2.97889140575354,1.91557803600459,-3.42129711016506));
#49347=CARTESIAN_POINT('Ctrl Pts',(-2.91802588924534,2.00718573517956,-3.42500160225013));
#49348=CARTESIAN_POINT('Ctrl Pts',(-2.85298611916,2.09572665294942,-3.42870609433519));
#49349=CARTESIAN_POINT('Ctrl Pts',(-2.80366994606909,2.16286248723414,-3.43151501221176));
#49350=CARTESIAN_POINT('Ctrl Pts',(-2.75195394466874,2.228235150624,-3.43432393008833));
#49351=CARTESIAN_POINT('Ctrl Pts',(-2.6979962409409,2.29169861659424,-3.43713284796491));
#49352=CARTESIAN_POINT('Ctrl Pts',(-2.57287736583807,2.43885976178261,-3.44364625792664));
#49353=CARTESIAN_POINT('Ctrl Pts',(-2.43570729771941,2.57575738080365,-3.45015966788836));
#49354=CARTESIAN_POINT('Ctrl Pts',(-2.2883737003719,2.70066337612947,-3.45667307785009));
#49355=CARTESIAN_POINT('Ctrl Pts',(-2.15209022701611,2.81620133347544,-3.46269797745857));
#49356=CARTESIAN_POINT('Ctrl Pts',(-2.00709305852713,2.92148977050388,-3.46872287706705));
#49357=CARTESIAN_POINT('Ctrl Pts',(-1.85491010713434,3.01511334686633,-3.47474777667553));
#49358=CARTESIAN_POINT('Ctrl Pts',(-1.84257082313618,3.02270452503107,-3.47523628702869));
#49359=CARTESIAN_POINT('Ctrl Pts',(-1.83018430263193,3.03021901994261,-3.47572479738184));
#49360=CARTESIAN_POINT('Ctrl Pts',(-1.81775158326284,3.03765643862568,-3.476213307735));
#49361=CARTESIAN_POINT('Ctrl Pts',(-1.65198355467242,3.13682108606072,-3.48272671769664));
#49362=CARTESIAN_POINT('Ctrl Pts',(-1.47802896465355,3.22226797334726,-3.48924012765827));
#49363=CARTESIAN_POINT('Ctrl Pts',(-1.2983289646543,3.29309365754754,-3.49575353761991));
#49364=CARTESIAN_POINT('Ctrl Pts',(-1.11862896465245,3.36391934174885,-3.50226694758164));
#49365=CARTESIAN_POINT('Ctrl Pts',(-0.933161824865596,3.42013406708304,
-3.50878035754337));
#49366=CARTESIAN_POINT('Ctrl Pts',(-0.744333208107735,3.46082430384987,
-3.51529376750508));
#49367=CARTESIAN_POINT('Ctrl Pts',(-0.691224574103849,3.47226855911735,
-3.51712568425432));
#49368=CARTESIAN_POINT('Ctrl Pts',(-0.637851134403885,3.48248437574009,
-3.51895760100355));
#49369=CARTESIAN_POINT('Ctrl Pts',(-0.58426852474683,3.4914510294415,-3.52078951775279));
#49370=CARTESIAN_POINT('Ctrl Pts',(-0.447337289462379,3.51436545961875,
-3.52547101096518));
#49371=CARTESIAN_POINT('Ctrl Pts',(-0.309040015184776,3.5291212435739,-3.53015250417759));
#49372=CARTESIAN_POINT('Ctrl Pts',(-0.17036733400844,3.53574588879975,-3.53483399739009));
#49373=CARTESIAN_POINT('Ctrl Pts',(0.0225694026298665,3.5449628262702,-3.54134740735197));
#49374=CARTESIAN_POINT('Ctrl Pts',(0.216252460440131,3.5384455628299,-3.54786081731403));
#49375=CARTESIAN_POINT('Ctrl Pts',(0.408132200521637,3.51626167940836,-3.55437422727593));
#49376=CARTESIAN_POINT('Ctrl Pts',(0.530455029403651,3.50211951216048,-3.55852650897002));
#49377=CARTESIAN_POINT('Ctrl Pts',(0.652051243402925,3.48160781812733,-3.56267879066404));
#49378=CARTESIAN_POINT('Ctrl Pts',(0.772227074543825,3.45474533726317,-3.56683107235804));
#49379=CARTESIAN_POINT('Ctrl Pts',(0.840563129972376,3.43947041913817,-3.5691922006257));
#49380=CARTESIAN_POINT('Ctrl Pts',(0.908439919140494,3.4221421540496,-3.57155332889335));
#49381=CARTESIAN_POINT('Ctrl Pts',(0.975740479931958,3.40281153553916,-3.573914457161));
#49382=CARTESIAN_POINT('Ctrl Pts',(1.16139585032783,3.34948607885153,-3.58042786712264));
#49383=CARTESIAN_POINT('Ctrl Pts',(1.34266063505881,3.28092736671375,-3.58694127708427));
#49384=CARTESIAN_POINT('Ctrl Pts',(1.51718923345482,3.19817302383904,-3.59345468704591));
#49385=CARTESIAN_POINT('Ctrl Pts',(1.69171783185335,3.11541868096314,-3.59996809700764));
#49386=CARTESIAN_POINT('Ctrl Pts',(1.85953065547441,3.01845588995455,-3.60648150696937));
#49387=CARTESIAN_POINT('Ctrl Pts',(2.0182261341945,2.90832651285219,-3.61299491693108));
#49388=CARTESIAN_POINT('Ctrl Pts',(2.1769216129123,2.79819713575142,-3.6195083268927));
#49389=CARTESIAN_POINT('Ctrl Pts',(2.32647647226952,2.67492498658273,-3.6260217368543));
#49390=CARTESIAN_POINT('Ctrl Pts',(2.4650724946873,2.54039012878225,-3.63253514681592));
#49391=CARTESIAN_POINT('Ctrl Pts',(2.60366851710708,2.40585527097982,-3.63904855677764));
#49392=CARTESIAN_POINT('Ctrl Pts',(2.73132470195812,2.26004289611969,-3.64556196673937));
#49393=CARTESIAN_POINT('Ctrl Pts',(2.84624348913382,2.10478420563982,-3.6520753767011));
#49394=CARTESIAN_POINT('Ctrl Pts',(2.88646538330249,2.05044323345657,-3.65435508824867));
#49395=CARTESIAN_POINT('Ctrl Pts',(2.92512609682342,1.99494564818121,-3.65663479979625));
#49396=CARTESIAN_POINT('Ctrl Pts',(2.96214566964451,1.93837381116374,-3.65891451134382));
#49397=CARTESIAN_POINT('Ctrl Pts',(3.03089546691971,1.83331310867443,-3.66314820975788));
#49398=CARTESIAN_POINT('Ctrl Pts',(3.09398468320899,1.72454722201944,-3.66738190817194));
#49399=CARTESIAN_POINT('Ctrl Pts',(3.1511361795063,1.61275723470709,-3.671615606586));
#49400=CARTESIAN_POINT('Ctrl Pts',(3.23906193351585,1.4407719051538,-3.67812901654764));
#49401=CARTESIAN_POINT('Ctrl Pts',(3.31294544834883,1.26161606945278,-3.68464242650927));
#49402=CARTESIAN_POINT('Ctrl Pts',(3.37182604181743,1.07765228385916,-3.69115583647091));
#49403=CARTESIAN_POINT('Ctrl Pts',(3.41341027855843,0.947728430153869,-3.69575591207952));
#49404=CARTESIAN_POINT('Ctrl Pts',(3.44751202204771,0.815396531481927,-3.70035598768814));
#49405=CARTESIAN_POINT('Ctrl Pts',(3.47377603053233,0.681527761501758,-3.70495606329676));
#49406=CARTESIAN_POINT('Ctrl Pts',(3.48470016177703,0.625846999226429,-3.70686939764987));
#49407=CARTESIAN_POINT('Ctrl Pts',(3.49426846685995,0.569900396495106,-3.70878273200298));
#49408=CARTESIAN_POINT('Ctrl Pts',(3.50248075017427,0.513755641688056,-3.7106960663561));
#49409=CARTESIAN_POINT('Ctrl Pts',(3.53043716451462,0.322626577048128,-3.71720947631773));
#49410=CARTESIAN_POINT('Ctrl Pts',(3.54267920096763,0.129214760060477,-3.72372288627937));
#49411=CARTESIAN_POINT('Ctrl Pts',(3.53921539307674,-0.063907964441538,
-3.730236296241));
#49412=CARTESIAN_POINT('Ctrl Pts',(3.53575158518584,-0.257030688943553,
-3.73674970620264));
#49413=CARTESIAN_POINT('Ctrl Pts',(3.51657975088695,-0.449888254626207,
-3.74326311616427));
#49414=CARTESIAN_POINT('Ctrl Pts',(3.48168686891133,-0.639875553680029,
-3.74977652612591));
#49415=CARTESIAN_POINT('Ctrl Pts',(3.47950604488335,-0.651749862803495,
-3.75018361777739));
#49416=CARTESIAN_POINT('Ctrl Pts',(3.47726383116518,-0.663612839943919,
-3.75059070942887));
#49417=CARTESIAN_POINT('Ctrl Pts',(3.4749602294045,-0.675463843633017,-3.75099780108035));
#49418=CARTESIAN_POINT('Ctrl Pts',(3.4404065224946,-0.853227255282967,-3.7571041193906));
#49419=CARTESIAN_POINT('Ctrl Pts',(3.39203987700435,-1.02829625861096,-3.76321043770085));
#49420=CARTESIAN_POINT('Ctrl Pts',(3.33067938429338,-1.19866546298495,-3.76931675601108));
#49421=CARTESIAN_POINT('Ctrl Pts',(3.26522815424471,-1.38039271933565,-3.7758301659727));
#49422=CARTESIAN_POINT('Ctrl Pts',(3.18498800540492,-1.55679625758723,-3.7823435759343));
#49423=CARTESIAN_POINT('Ctrl Pts',(3.09091242647188,-1.72550011744132,-3.78885698589592));
#49424=CARTESIAN_POINT('Ctrl Pts',(3.05151811292345,-1.79614515441368,-3.79158448773229));
#49425=CARTESIAN_POINT('Ctrl Pts',(3.00969732231895,-1.86543959636863,-3.79431198956866));
#49426=CARTESIAN_POINT('Ctrl Pts',(2.965524256836,-1.9332009419914,-3.79703949140504));
#49427=CARTESIAN_POINT('Ctrl Pts',(2.90420984622655,-2.02725705794212,-3.80082539953039));
#49428=CARTESIAN_POINT('Ctrl Pts',(2.83836319021171,-2.11835920742328,-3.80461130765574));
#49429=CARTESIAN_POINT('Ctrl Pts',(2.76835115646748,-2.20612920640356,-3.80839721578109));
#49430=CARTESIAN_POINT('Ctrl Pts',(2.64789998255489,-2.35713181047166,-3.81491062574273));
#49431=CARTESIAN_POINT('Ctrl Pts',(2.5151152522304,-2.49828401989007,-3.82142403570437));
#49432=CARTESIAN_POINT('Ctrl Pts',(2.37177668926012,-2.62775728359333,-3.827937445666));
#49433=CARTESIAN_POINT('Ctrl Pts',(2.26068970700779,-2.7280986979979,-3.83298532002595));
#49434=CARTESIAN_POINT('Ctrl Pts',(2.14325235121661,-2.82143218116641,-3.83803319438591));
#49435=CARTESIAN_POINT('Ctrl Pts',(2.02032602960248,-2.90686820033367,-3.84308106874586));
#49436=CARTESIAN_POINT('Ctrl Pts',(1.98463716576339,-2.93167260686741,-3.84454660434754));
#49437=CARTESIAN_POINT('Ctrl Pts',(1.94848569380674,-2.95581139752882,-3.84601213994922));
#49438=CARTESIAN_POINT('Ctrl Pts',(1.91189931312508,-2.97927230421048,-3.84747767555091));
#49439=CARTESIAN_POINT('Ctrl Pts',(1.7492952138987,-3.08354169426571,-3.85399108551264));
#49440=CARTESIAN_POINT('Ctrl Pts',(1.57811819344313,-3.17441162854151,-3.86050449547437));
#49441=CARTESIAN_POINT('Ctrl Pts',(1.40073455162058,-3.25085348915537,-3.8670179054361));
#49442=CARTESIAN_POINT('Ctrl Pts',(1.22335090980063,-3.32729534976811,-3.87353131539773));
#49443=CARTESIAN_POINT('Ctrl Pts',(1.03973833991381,-3.38931797648445,-3.88004472535937));
#49444=CARTESIAN_POINT('Ctrl Pts',(0.852266212883417,-3.43586620221265,
-3.88655813532117));
#49445=CARTESIAN_POINT('Ctrl Pts',(0.827660202824008,-3.44197572968566,
-3.88741303057189));
#49446=CARTESIAN_POINT('Ctrl Pts',(0.802988161574587,-3.44781855384957,
-3.88826792582262));
#49447=CARTESIAN_POINT('Ctrl Pts',(0.778255563408939,-3.4533922855685,-3.88912282107334));
#49448=CARTESIAN_POINT('Ctrl Pts',(0.614551565234618,-3.49028457488758,
-3.89478133578446));
#49449=CARTESIAN_POINT('Ctrl Pts',(0.448194483402658,-3.51538663874368,
-3.90043985049566));
#49450=CARTESIAN_POINT('Ctrl Pts',(0.280916493409238,-3.52865236474662,
-3.90609836520674));
#49451=CARTESIAN_POINT('Ctrl Pts',(0.0883659422379453,-3.54392229268905,
-3.91261177516864));
#49452=CARTESIAN_POINT('Ctrl Pts',(-0.105427797081422,-3.54351519011934,
-3.91912518513037));
#49453=CARTESIAN_POINT('Ctrl Pts',(-0.297910355108321,-3.52735115969274,
-3.92563859509208));
#49454=CARTESIAN_POINT('Ctrl Pts',(-0.39174565726025,-3.51947119023151,
-3.92881388431341));
#49455=CARTESIAN_POINT('Ctrl Pts',(-0.485270507195668,-3.50784551008206,
-3.93198917353473));
#49456=CARTESIAN_POINT('Ctrl Pts',(-0.578173906335351,-3.49246545208883,
-3.93516446275606));
#49457=CARTESIAN_POINT('Ctrl Pts',(-0.675841470420018,-3.47629669170343,
-3.93850258349635));
#49458=CARTESIAN_POINT('Ctrl Pts',(-0.772822162007415,-3.45597860468362,
-3.94184070423663));
#49459=CARTESIAN_POINT('Ctrl Pts',(-0.868777181623859,-3.43163722187875,
-3.94517882497692));
#49460=CARTESIAN_POINT('Ctrl Pts',(-1.05600659280207,-3.38414181425924,
-3.95169223493864));
#49461=CARTESIAN_POINT('Ctrl Pts',(-1.23933903044262,-3.32133059983808,
-3.95820564490036));
#49462=CARTESIAN_POINT('Ctrl Pts',(-1.41638310527089,-3.24410123108816,
-3.96471905486209));
#49463=CARTESIAN_POINT('Ctrl Pts',(-1.56576369723281,-3.17893910221207,
-3.97021473178163));
#49464=CARTESIAN_POINT('Ctrl Pts',(-1.71068137496023,-3.10350315118168,
-3.97571040870116));
#49465=CARTESIAN_POINT('Ctrl Pts',(-1.8496449190945,-3.0183461818135,-3.98120608562069));
#49466=CARTESIAN_POINT('Ctrl Pts',(-1.87537929041651,-3.00257613878509,
-3.9822238186628));
#49467=CARTESIAN_POINT('Ctrl Pts',(-1.90090948182522,-2.98647275324273,
-3.9832415517049));
#49468=CARTESIAN_POINT('Ctrl Pts',(-1.9262280359204,-2.97004283162531,-3.984259284747));
#49469=CARTESIAN_POINT('Ctrl Pts',(-2.08826475442685,-2.86489264910712,
-3.99077269470864));
#49470=CARTESIAN_POINT('Ctrl Pts',(-2.24161193500656,-2.74638268846562,
-3.99728610467027));
#49471=CARTESIAN_POINT('Ctrl Pts',(-2.38436956161414,-2.61627287473533,
-4.00379951463191));
#49472=CARTESIAN_POINT('Ctrl Pts',(-2.52712718822379,-2.48616306100314,
-4.01031292459364));
#49473=CARTESIAN_POINT('Ctrl Pts',(-2.65931321192137,-2.34443748176244,
-4.01682633455537));
#49474=CARTESIAN_POINT('Ctrl Pts',(-2.77901650300382,-2.19283463489973,
-4.0233397445171));
#49475=CARTESIAN_POINT('Ctrl Pts',(-2.80295746726397,-2.16251367792641,
-4.02464244316218));
#49476=CARTESIAN_POINT('Ctrl Pts',(-2.8263985174789,-2.13179828445587,-4.02594514180727));
#49477=CARTESIAN_POINT('Ctrl Pts',(-2.84932404264,-2.10070285857735,-4.02724784045235));
#49478=CARTESIAN_POINT('Ctrl Pts',(-2.94102467796757,-1.97632314257066,
-4.0324585517689));
#49479=CARTESIAN_POINT('Ctrl Pts',(-3.02447624802702,-1.84586260784311,
-4.03766926308545));
#49480=CARTESIAN_POINT('Ctrl Pts',(-3.09909838196629,-1.71055094354732,
-4.042879974402));
#49481=CARTESIAN_POINT('Ctrl Pts',(-3.19237634749372,-1.54141082262935,
-4.04939338436364));
#49482=CARTESIAN_POINT('Ctrl Pts',(-3.27187296306989,-1.36467341810391,
-4.05590679432527));
#49483=CARTESIAN_POINT('Ctrl Pts',(-3.33649164232266,-1.18264363939907,
-4.06242020428691));
#49484=CARTESIAN_POINT('Ctrl Pts',(-3.37243570168691,-1.08138980308597,
-4.06604328041647));
#49485=CARTESIAN_POINT('Ctrl Pts',(-3.40377624648734,-0.978494886681129,
-4.06966635654604));
#49486=CARTESIAN_POINT('Ctrl Pts',(-3.43031568918,-0.874376505038574,-4.0732894326756));
#49487=CARTESIAN_POINT('Ctrl Pts',(-3.45148771161571,-0.791315351960366,
-4.07617976650776));
#49488=CARTESIAN_POINT('Ctrl Pts',(-3.4696043187652,-0.707475623527939,
-4.07907010033992));
#49489=CARTESIAN_POINT('Ctrl Pts',(-3.48465193556905,-0.623091478798857,
-4.08196043417208));
#49490=CARTESIAN_POINT('Ctrl Pts',(-3.51856196218893,-0.432930562863846,
-4.0884738441337));
#49491=CARTESIAN_POINT('Ctrl Pts',(-3.5368901719826,-0.240004247211696,
-4.0949872540953));
#49492=CARTESIAN_POINT('Ctrl Pts',(-3.539499078369,-0.0468671734762678,
-4.10150066405692));
#49493=CARTESIAN_POINT('Ctrl Pts',(-3.5418797031369,0.129370235321772,-4.10744414488054));
#49494=CARTESIAN_POINT('Ctrl Pts',(-3.53116871553553,0.305802937702781,
-4.11338762570416));
#49495=CARTESIAN_POINT('Ctrl Pts',(-3.50724735526867,0.480433126417416,
-4.11933110652779));
#49496=CARTESIAN_POINT('Ctrl Pts',(-3.50495350076762,0.497178672654429,
-4.11990103566589));
#49497=CARTESIAN_POINT('Ctrl Pts',(-3.50253818434456,0.513907643630247,
-4.12047096480399));
#49498=CARTESIAN_POINT('Ctrl Pts',(-3.50000197035076,0.530618368380382,
-4.12104089394209));
#49499=CARTESIAN_POINT('Ctrl Pts',(-3.47101696083347,0.72159614750572,-4.12755430390373));
#49500=CARTESIAN_POINT('Ctrl Pts',(-3.42624638929545,0.910161095558849,
-4.13406771386537));
#49501=CARTESIAN_POINT('Ctrl Pts',(-3.36654108656219,1.09385548621155,-4.140581123827));
#49502=CARTESIAN_POINT('Ctrl Pts',(-3.30683578382893,1.27754987686425,-4.14709453378864));
#49503=CARTESIAN_POINT('Ctrl Pts',(-3.23218964468241,1.45639693625083,-4.15360794375027));
#49504=CARTESIAN_POINT('Ctrl Pts',(-3.14342402551079,1.62795644980454,-4.16012135371191));
#49505=CARTESIAN_POINT('Ctrl Pts',(-3.11956799202827,1.67406359734405,-4.16187185269541));
#49506=CARTESIAN_POINT('Ctrl Pts',(-3.09469253710093,1.71964329765716,-4.16362235167892));
#49507=CARTESIAN_POINT('Ctrl Pts',(-3.06881449123183,1.76464659872848,-4.16537285066242));
#49508=CARTESIAN_POINT('Ctrl Pts',(-2.99840323711153,1.88709552257745,-4.17013576164065));
#49509=CARTESIAN_POINT('Ctrl Pts',(-2.92056891533613,2.00527672011598,-4.17489867261887));
#49510=CARTESIAN_POINT('Ctrl Pts',(-2.83599569248695,2.11840306211022,-4.17966158359708));
#49511=CARTESIAN_POINT('Ctrl Pts',(-2.72033951610409,2.27310640345701,-4.1861749935587));
#49512=CARTESIAN_POINT('Ctrl Pts',(-2.59207227250994,2.4183755860845,-4.1926884035203));
#49513=CARTESIAN_POINT('Ctrl Pts',(-2.45286430442405,2.55228290197142,-4.19920181348192));
#49514=CARTESIAN_POINT('Ctrl Pts',(-2.36585966860048,2.63597464327796,-4.20327267860173));
#49515=CARTESIAN_POINT('Ctrl Pts',(-2.27457583085879,2.71523107830464,-4.20734354372155));
#49516=CARTESIAN_POINT('Ctrl Pts',(-2.17944162265286,2.78955806776767,-4.2114144088414));
#49517=CARTESIAN_POINT('Ctrl Pts',(-2.12236049549604,2.83415473196168,-4.21385695368334));
#49518=CARTESIAN_POINT('Ctrl Pts',(-2.06389331379296,2.87697685360123,-4.21629949852529));
#49519=CARTESIAN_POINT('Ctrl Pts',(-2.00416594676152,2.91796018932203,-4.21874204336726));
#49520=CARTESIAN_POINT('Ctrl Pts',(-1.84489401826728,3.02724836391952,-4.22525545332906));
#49521=CARTESIAN_POINT('Ctrl Pts',(-1.67666686505147,3.12346020277471,-4.23176886329103));
#49522=CARTESIAN_POINT('Ctrl Pts',(-1.50177399217723,3.20544206238398,-4.23828227325283));
#49523=CARTESIAN_POINT('Ctrl Pts',(-1.33016037878431,3.28588675363412,-4.24467355610321));
#49524=CARTESIAN_POINT('Ctrl Pts',(-1.15210659968557,3.35263728831822,-4.25106483895343));
#49525=CARTESIAN_POINT('Ctrl Pts',(-0.969815634171214,3.40456423580433,
-4.25745612180364));
#49526=CARTESIAN_POINT('Ctrl Pts',(-0.966332347704576,3.40555647605564,
-4.25757824891506));
#49527=CARTESIAN_POINT('Ctrl Pts',(-0.962847514285249,3.40654330398007,
-4.25770037602648));
#49528=CARTESIAN_POINT('Ctrl Pts',(-0.959361151106016,3.4075247180546,-4.25782250313791));
#49529=CARTESIAN_POINT('Ctrl Pts',(-0.773422808690397,3.45986651288758,
-4.26433591309964));
#49530=CARTESIAN_POINT('Ctrl Pts',(-0.583164165584344,3.49679998871353,
-4.27084932306137));
#49531=CARTESIAN_POINT('Ctrl Pts',(-0.391189760153187,3.51811400704572,
-4.27736273302309));
#49532=CARTESIAN_POINT('Ctrl Pts',(-0.199215354724813,3.53942802537761,
-4.28387614298473));
#49533=CARTESIAN_POINT('Ctrl Pts',(-0.00550164725985493,3.54512763200719,
-4.29038955294637));
#49534=CARTESIAN_POINT('Ctrl Pts',(0.187394174250291,3.53498576596323,-4.296902962908));
#49535=CARTESIAN_POINT('Ctrl Pts',(0.25249707115236,3.53156285688057,-4.29910125758278));
#49536=CARTESIAN_POINT('Ctrl Pts',(0.317505759619646,3.52633524440815,-4.30129955225756));
#49537=CARTESIAN_POINT('Ctrl Pts',(0.382317719199291,3.519294412462,-4.30349784693234));
#49538=CARTESIAN_POINT('Ctrl Pts',(0.509539551996122,3.50547369865527,-4.3078129622192));
#49539=CARTESIAN_POINT('Ctrl Pts',(0.636003219410405,3.48466589220727,-4.31212807750605));
#49540=CARTESIAN_POINT('Ctrl Pts',(0.760965615923843,3.45710192869036,-4.31644319279291));
#49541=CARTESIAN_POINT('Ctrl Pts',(0.949588923572606,3.41549576463196,-4.32295660275463));
#49542=CARTESIAN_POINT('Ctrl Pts',(1.13480966416368,3.35849703359421,-4.32947001271637));
#49543=CARTESIAN_POINT('Ctrl Pts',(1.31419238471769,3.28686253261049,-4.33598342267808));
#49544=CARTESIAN_POINT('Ctrl Pts',(1.43863859651384,3.23716631742433,-4.34050208084709));
#49545=CARTESIAN_POINT('Ctrl Pts',(1.56028265268397,3.18042068936791,-4.34502073901609));
#49546=CARTESIAN_POINT('Ctrl Pts',(1.67827226002658,3.1168898314225,-4.3495393971851));
#49547=CARTESIAN_POINT('Ctrl Pts',(1.73035851482898,3.08884427275604,-4.3515341489777));
#49548=CARTESIAN_POINT('Ctrl Pts',(1.78173265010367,3.05947655931791,-4.35352890077031));
#49549=CARTESIAN_POINT('Ctrl Pts',(1.83233522030034,3.02883524024529,-4.35552365256292));
#49550=CARTESIAN_POINT('Ctrl Pts',(1.99756644657541,2.92878295623329,-4.36203706252464));
#49551=CARTESIAN_POINT('Ctrl Pts',(2.15456198585818,2.81515968928226,-4.36855047248637));
#49552=CARTESIAN_POINT('Ctrl Pts',(2.30134084431348,2.68960344508741,-4.37506388244809));
#49553=CARTESIAN_POINT('Ctrl Pts',(2.44811970276666,2.56404720089438,-4.38157729240973));
#49554=CARTESIAN_POINT('Ctrl Pts',(2.58469882886557,2.42654092551998,-4.38809070237137));
#49555=CARTESIAN_POINT('Ctrl Pts',(2.70905533377063,2.2787296820682,-4.394604112333));
#49556=CARTESIAN_POINT('Ctrl Pts',(2.71527320777415,2.2713390619411,-4.39492978538489));
#49557=CARTESIAN_POINT('Ctrl Pts',(2.72146047398848,2.26392273951171,-4.39525545843678));
#49558=CARTESIAN_POINT('Ctrl Pts',(2.72761687942599,2.25648092371001,-4.39558113148867));
#49559=CARTESIAN_POINT('Ctrl Pts',(2.84458761721353,2.1150875905972,-4.40176886839842));
#49560=CARTESIAN_POINT('Ctrl Pts',(2.95041694207574,1.96449093844901,-4.40795660530816));
#49561=CARTESIAN_POINT('Ctrl Pts',(3.04403466981377,1.80667228922409,-4.4141443422179));
#49562=CARTESIAN_POINT('Ctrl Pts',(3.14257968705312,1.64054732673751,-4.42065775217963));
#49563=CARTESIAN_POINT('Ctrl Pts',(3.2276089004457,1.4664013198912,-4.42717116214137));
#49564=CARTESIAN_POINT('Ctrl Pts',(3.29789079596611,1.2864798567823,-4.4336845721031));
#49565=CARTESIAN_POINT('Ctrl Pts',(3.32644295523914,1.21338640599696,-4.43633065780213));
#49566=CARTESIAN_POINT('Ctrl Pts',(3.35256060096538,1.13933993490305,-4.43897674350117));
#49567=CARTESIAN_POINT('Ctrl Pts',(3.37615800564866,1.06449853024478,-4.44162282920021));
#49568=CARTESIAN_POINT('Ctrl Pts',(3.410646236963,0.955115837089003,-4.44549015346281));
#49569=CARTESIAN_POINT('Ctrl Pts',(3.43975080156849,0.844035097395934,-4.4493574777254));
#49570=CARTESIAN_POINT('Ctrl Pts',(3.46340847798809,0.731814199250707,-4.453224801988));
#49571=CARTESIAN_POINT('Ctrl Pts',(3.50325311857094,0.542809950770156,-4.45973821194964));
#49572=CARTESIAN_POINT('Ctrl Pts',(3.52765418600473,0.350559382295599,-4.46625162191127));
#49573=CARTESIAN_POINT('Ctrl Pts',(3.53632795873358,0.157598006434378,-4.47276503187291));
#49574=CARTESIAN_POINT('Ctrl Pts',(3.54294168510181,0.0104655210122198,
-4.47773148794191));
#49575=CARTESIAN_POINT('Ctrl Pts',(3.54040940290031,-0.137092750504991,
-4.48269794401091));
#49576=CARTESIAN_POINT('Ctrl Pts',(3.52859722973483,-0.283904192124258,
-4.4876644000799));
#49577=CARTESIAN_POINT('Ctrl Pts',(3.52491796890859,-0.329633083703001,
-4.48921135397263));
#49578=CARTESIAN_POINT('Ctrl Pts',(3.52033846393456,-0.375289512400935,
-4.49075830786536));
#49579=CARTESIAN_POINT('Ctrl Pts',(3.5148682535165,-0.420839119723915,-4.49230526175808));
#49580=CARTESIAN_POINT('Ctrl Pts',(3.49183607188734,-0.612624581126916,
-4.4988186717197));
#49581=CARTESIAN_POINT('Ctrl Pts',(3.4530172602035,-0.80249780061272,-4.5053320816813));
#49582=CARTESIAN_POINT('Ctrl Pts',(3.3991184205719,-0.987978897271879,-4.51184549164292));
#49583=CARTESIAN_POINT('Ctrl Pts',(3.34521958093952,-1.17345999393373,-4.51835890160464));
#49584=CARTESIAN_POINT('Ctrl Pts',(3.2762331580479,-1.35457174622048,-4.52487231156637));
#49585=CARTESIAN_POINT('Ctrl Pts',(3.19284833403879,-1.52881164096968,-4.5313857215281));
#49586=CARTESIAN_POINT('Ctrl Pts',(3.18294627225166,-1.5495028665505,-4.5321591978609));
#49587=CARTESIAN_POINT('Ctrl Pts',(3.17284133069424,-1.57009682188359,-4.5329326741937));
#49588=CARTESIAN_POINT('Ctrl Pts',(3.1625347146805,-1.5905892551004,-4.5337061505265));
#49589=CARTESIAN_POINT('Ctrl Pts',(3.08604977345116,-1.74266269493216,-4.53944608415534));
#49590=CARTESIAN_POINT('Ctrl Pts',(2.99845761324308,-1.88914457163618,-4.54518601778417));
#49591=CARTESIAN_POINT('Ctrl Pts',(2.90086776956525,-2.02860868265436,-4.550925951413));
#49592=CARTESIAN_POINT('Ctrl Pts',(2.79012734971569,-2.18686607528926,-4.55743936137464));
#49593=CARTESIAN_POINT('Ctrl Pts',(2.6665030824214,-2.33610851677235,-4.56395277133627));
#49594=CARTESIAN_POINT('Ctrl Pts',(2.53155468743157,-2.47431060311237,-4.57046618129807));
#49595=CARTESIAN_POINT('Ctrl Pts',(2.46745412259722,-2.53995667319974,-4.57356005475674));
#49596=CARTESIAN_POINT('Ctrl Pts',(2.40079731960751,-2.60311185453884,-4.57665392821545));
#49597=CARTESIAN_POINT('Ctrl Pts',(2.33176068881981,-2.66354877749069,-4.57974780167416));
#49598=CARTESIAN_POINT('Ctrl Pts',(2.25545721933669,-2.7303473285424,-4.58316733817743));
#49599=CARTESIAN_POINT('Ctrl Pts',(2.17624654724241,-2.79382517537667,-4.5865868746807));
#49600=CARTESIAN_POINT('Ctrl Pts',(2.09446454668198,-2.85378693812754,-4.59000641118393));
#49601=CARTESIAN_POINT('Ctrl Pts',(1.93868913775044,-2.96799994403061,-4.59651982114573));
#49602=CARTESIAN_POINT('Ctrl Pts',(1.77358024536384,-3.06946424600634,-4.60303323110737));
#49603=CARTESIAN_POINT('Ctrl Pts',(1.60134875634575,-3.15690183524312,-4.609546641069));
#49604=CARTESIAN_POINT('Ctrl Pts',(1.45818170002382,-3.22958414400259,-4.61496089914771));
#49605=CARTESIAN_POINT('Ctrl Pts',(1.31007763847309,-3.29257884054208,-4.62037515722643));
#49606=CARTESIAN_POINT('Ctrl Pts',(1.15835136238572,-3.34511914903784,-4.62578941530514));
#49607=CARTESIAN_POINT('Ctrl Pts',(1.12754931718851,-3.35578538957768,-4.62688856718806));
#49608=CARTESIAN_POINT('Ctrl Pts',(1.09659801000313,-3.36602081032388,-4.62798771907099));
#49609=CARTESIAN_POINT('Ctrl Pts',(1.06551003781568,-3.37582359101795,-4.62908687095391));
#49610=CARTESIAN_POINT('Ctrl Pts',(0.8812873558714,-3.43391340591755,-4.63560028091563));
#49611=CARTESIAN_POINT('Ctrl Pts',(0.692289542666389,-3.47680428037546,
-4.64211369087736));
#49612=CARTESIAN_POINT('Ctrl Pts',(0.501080685143525,-3.50414476472143,
-4.64862710083908));
#49613=CARTESIAN_POINT('Ctrl Pts',(0.309871827623432,-3.53148524906699,
-4.6551405108007));
#49614=CARTESIAN_POINT('Ctrl Pts',(0.116428217970221,-3.54327886708705,
-4.6616539207623));
#49615=CARTESIAN_POINT('Ctrl Pts',(-0.0766918204989502,-3.53915174526628,
-4.66816733072392));
#49616=CARTESIAN_POINT('Ctrl Pts',(-0.112902286566704,-3.53837790011881,
-4.66938861056764));
#49617=CARTESIAN_POINT('Ctrl Pts',(-0.149100544630311,-3.53704430365368,
-4.67060989041136));
#49618=CARTESIAN_POINT('Ctrl Pts',(-0.185269285100072,-3.53514855303133,
-4.67183117025508));
#49619=CARTESIAN_POINT('Ctrl Pts',(-0.341998049399606,-3.52693376178892,
-4.67712330037308));
#49620=CARTESIAN_POINT('Ctrl Pts',(-0.49817233969735,-3.50816226468903,
-4.68241543049107));
#49621=CARTESIAN_POINT('Ctrl Pts',(-0.652411741910373,-3.47918285964478,
-4.687707560609));
#49622=CARTESIAN_POINT('Ctrl Pts',(-0.842245399180027,-3.44351579684425,
-4.69422097028656));
#49623=CARTESIAN_POINT('Ctrl Pts',(-1.02917125682124,-3.39238617446652,
-4.70073437996402));
#49624=CARTESIAN_POINT('Ctrl Pts',(-1.21071388767511,-3.32640898762537,
-4.70724778964203));
#49625=CARTESIAN_POINT('',(-3.939231012049,0.6945927106677,-1.608333333333));
#49626=CARTESIAN_POINT('Ctrl Pts',(-1.507124460135,-3.179723940534,0.3249781788769));
#49627=CARTESIAN_POINT('Ctrl Pts',(-1.847411431725,-3.018434838732,0.3122038733214));
#49628=CARTESIAN_POINT('Ctrl Pts',(-2.475686234802,-2.585698153946,0.2866552622103));
#49629=CARTESIAN_POINT('Ctrl Pts',(-3.165156557639,-1.672326772638,0.2483323455436));
#49630=CARTESIAN_POINT('Ctrl Pts',(-3.531155462695,-0.588062549222,0.2100094288769));
#49631=CARTESIAN_POINT('Ctrl Pts',(-3.53629937207,0.5562993812307,0.1716865122103));
#49632=CARTESIAN_POINT('Ctrl Pts',(-3.180057548144,1.643810961166,0.1333635955436));
#49633=CARTESIAN_POINT('Ctrl Pts',(-2.498836731037,2.563336879767,0.09504067887693));
#49634=CARTESIAN_POINT('Ctrl Pts',(-1.56225248291,3.220907950999,0.05671776221027));
#49635=CARTESIAN_POINT('Ctrl Pts',(-0.466017154887,3.54932513108,0.0183948455436));
#49636=CARTESIAN_POINT('Ctrl Pts',(0.6778418198014,3.515026505956,-0.01992807112307));
#49637=CARTESIAN_POINT('Ctrl Pts',(1.752430176593,3.121517154665,-0.05825098778973));
#49638=CARTESIAN_POINT('Ctrl Pts',(2.647932624627,2.409010935266,-0.0965739044564));
#49639=CARTESIAN_POINT('Ctrl Pts',(3.272835177738,1.450320919686,-0.1348968211231));
#49640=CARTESIAN_POINT('Ctrl Pts',(3.563277236448,0.3434184138391,-0.1732197377897));
#49641=CARTESIAN_POINT('Ctrl Pts',(3.489577686554,-0.7985790131506,-0.2115426544564));
#49642=CARTESIAN_POINT('Ctrl Pts',(3.059268098266,-1.858967340668,-0.2498655711231));
#49643=CARTESIAN_POINT('Ctrl Pts',(2.316323053204,-2.729382418045,-0.2881884877897));
#49644=CARTESIAN_POINT('Ctrl Pts',(1.336666254706,-3.320874010599,-0.3265114044564));
#49645=CARTESIAN_POINT('Ctrl Pts',(0.2204116649468,-3.572995881427,-0.3648343211231));
#49646=CARTESIAN_POINT('Ctrl Pts',(-0.9183674304569,-3.459982967215,-0.4031572377897));
#49647=CARTESIAN_POINT('Ctrl Pts',(-1.9632959015,-2.993384384588,-0.4414801544564));
#49648=CARTESIAN_POINT('Ctrl Pts',(-2.807589484972,-2.220883192474,-0.4798030711231));
#49649=CARTESIAN_POINT('Ctrl Pts',(-3.364967377215,-1.221423522379,-0.5181259877897));
#49650=CARTESIAN_POINT('Ctrl Pts',(-3.578469519044,-0.09714304921396,-0.5564489044564));
#49651=CARTESIAN_POINT('Ctrl Pts',(-3.426277508971,1.037064753165,-0.5947718211231));
#49652=CARTESIAN_POINT('Ctrl Pts',(-2.923944288764,2.06529190841,-0.6330947377897));
#49653=CARTESIAN_POINT('Ctrl Pts',(-2.122804743339,2.882460909084,-0.6714176544564));
#49654=CARTESIAN_POINT('Ctrl Pts',(-1.104729640369,3.405062891112,-0.7097405711231));
#49655=CARTESIAN_POINT('Ctrl Pts',(0.02624098029853,3.579691646175,-0.7480634877897));
#49656=CARTESIAN_POINT('Ctrl Pts',(1.15452995928,3.388501356628,-0.7863864044564));
#49657=CARTESIAN_POINT('Ctrl Pts',(2.164834181912,2.851030311232,-0.8247093211231));
#49658=CARTESIAN_POINT('Ctrl Pts',(2.95390773709,2.022204230908,-0.8630322377897));
#49659=CARTESIAN_POINT('Ctrl Pts',(3.441112915587,0.9867232504197,-0.9013551544564));
#49660=CARTESIAN_POINT('Ctrl Pts',(3.576660810833,-0.1495938334094,-0.9396780711231));
#49661=CARTESIAN_POINT('Ctrl Pts',(3.3466993913,-1.270623490659,-0.9780009877897));
#49662=CARTESIAN_POINT('Ctrl Pts',(2.77472907968,-2.261804457755,-1.016323904456));
#49663=CARTESIAN_POINT('Ctrl Pts',(1.919201176706,-3.021845084393,-1.054646821123));
#49664=CARTESIAN_POINT('Ctrl Pts',(0.8675445536438,-3.473074620302,-1.09296973779));
#49665=CARTESIAN_POINT('Ctrl Pts',(-0.2727689569774,-3.569380613895,-1.131292654456));
#49666=CARTESIAN_POINT('Ctrl Pts',(-1.385207418822,-3.300921277095,-1.169615571123));
#49667=CARTESIAN_POINT('Ctrl Pts',(-2.356087527427,-2.695131246125,-1.20793848779));
#49668=CARTESIAN_POINT('Ctrl Pts',(-3.086192235944,-1.813917956672,-1.246261404456));
#49669=CARTESIAN_POINT('Ctrl Pts',(-3.500910032172,-0.7473351439477,-1.284584321123));
#49670=CARTESIAN_POINT('Ctrl Pts',(-3.557859704823,0.3956200090186,-1.32290723779));
#49671=CARTESIAN_POINT('Ctrl Pts',(-3.251221402107,1.498145608819,-1.361230154456));
#49672=CARTESIAN_POINT('Ctrl Pts',(-2.612331379217,2.447571375037,-1.399553071123));
#49673=CARTESIAN_POINT('Ctrl Pts',(-1.706479655765,3.146872742136,-1.43787598779));
#49674=CARTESIAN_POINT('Ctrl Pts',(-0.6262378398082,3.524586080483,-1.476198904456));
#49675=CARTESIAN_POINT('Ctrl Pts',(0.5180010325718,3.542111771387,-1.514521821123));
#49676=CARTESIAN_POINT('Ctrl Pts',(1.609303880967,3.197658813796,-1.55284473779));
#49677=CARTESIAN_POINT('Ctrl Pts',(2.536147310391,2.526427851876,-1.591167654456));
#49678=CARTESIAN_POINT('Ctrl Pts',(3.203814509633,1.597013919356,-1.629490571123));
#49679=CARTESIAN_POINT('Ctrl Pts',(3.544074636176,0.504396514588,-1.66781348779));
#49680=CARTESIAN_POINT('Ctrl Pts',(3.522155523411,-0.639766629091,-1.706136404456));
#49681=CARTESIAN_POINT('Ctrl Pts',(3.140297148798,-1.718550170333,-1.744459321123));
#49682=CARTESIAN_POINT('Ctrl Pts',(2.437522724574,-2.6217100979,-1.78278223779));
#49683=CARTESIAN_POINT('Ctrl Pts',(1.485650801008,-3.25694988789,-1.821105154456));
#49684=CARTESIAN_POINT('Ctrl Pts',(0.3819559277091,-3.55935254203,-1.859428071123));
#49685=CARTESIAN_POINT('Ctrl Pts',(-0.7607721390542,-3.498014682644,-1.89775098779));
#49686=CARTESIAN_POINT('Ctrl Pts',(-1.825754654292,-3.07920451219,-1.936073904456));
#49687=CARTESIAN_POINT('Ctrl Pts',(-2.704158191128,-2.345721792501,-1.974396821123));
#49688=CARTESIAN_POINT('Ctrl Pts',(-3.306215340777,-1.372521979396,-2.01271973779));
#49689=CARTESIAN_POINT('Ctrl Pts',(-3.570403165657,-0.2590638985198,-2.051042654456));
#49690=CARTESIAN_POINT('Ctrl Pts',(-3.469712261373,0.8808825686702,-2.089365571123));
#49691=CARTESIAN_POINT('Ctrl Pts',(-3.166220516368,1.580799011723,-2.114914182234));
#49692=CARTESIAN_POINT('Ctrl Pts',(-2.963111000121,1.897904549051,-2.12768848779));
#49693=CARTESIAN_POINT('Ctrl Pts',(-1.57884649994,-3.331042755313,0.2282975453458));
#49694=CARTESIAN_POINT('Ctrl Pts',(-1.935327273944,-3.16207812061,0.2155232397903));
#49695=CARTESIAN_POINT('Ctrl Pts',(-2.593500835636,-2.708748075055,0.1899746286792));
#49696=CARTESIAN_POINT('Ctrl Pts',(-3.315782130125,-1.751910569814,0.1516517120125));
#49697=CARTESIAN_POINT('Ctrl Pts',(-3.699198434163,-0.6160476603915,0.1133287953458));
#49698=CARTESIAN_POINT('Ctrl Pts',(-3.704587135314,0.5827729256655,0.07500587867917));
#49699=CARTESIAN_POINT('Ctrl Pts',(-3.331392238863,1.722037728966,0.0366829620125));
#49700=CARTESIAN_POINT('Ctrl Pts',(-2.617753033062,2.685322657708,-0.001639954654168));
#49701=CARTESIAN_POINT('Ctrl Pts',(-1.636597991677,3.374186657821,-0.03996287132083));
#49702=CARTESIAN_POINT('Ctrl Pts',(-0.4881942887712,3.718232772795,-0.0782857879875));
#49703=CARTESIAN_POINT('Ctrl Pts',(0.7100994065285,3.682301921918,-0.1166087046542));
#49704=CARTESIAN_POINT('Ctrl Pts',(1.835825987759,3.270065986259,-0.1549316213208));
#49705=CARTESIAN_POINT('Ctrl Pts',(2.773944201061,2.523652547661,-0.1932545379875));
#49706=CARTESIAN_POINT('Ctrl Pts',(3.428585031915,1.51933975488,-0.2315774546542));
#49707=CARTESIAN_POINT('Ctrl Pts',(3.73284884022,0.3597612374072,-0.2699003713208));
#49708=CARTESIAN_POINT('Ctrl Pts',(3.655642027196,-0.8365823216256,-0.3082232879875));
#49709=CARTESIAN_POINT('Ctrl Pts',(3.20485458042,-1.947433113158,-0.3465462046542));
#49710=CARTESIAN_POINT('Ctrl Pts',(2.426553773107,-2.859270081346,-0.3848691213208));
#49711=CARTESIAN_POINT('Ctrl Pts',(1.400276416216,-3.478909968661,-0.4231920379875));
#49712=CARTESIAN_POINT('Ctrl Pts',(0.2309007616505,-3.743029982531,-0.4615149546542));
#49713=CARTESIAN_POINT('Ctrl Pts',(-0.9620713096952,-3.624638934697,-0.4998378713208));
#49714=CARTESIAN_POINT('Ctrl Pts',(-2.056726530835,-3.135835548816,-0.5381607879875));
#49715=CARTESIAN_POINT('Ctrl Pts',(-2.941198918117,-2.326572056896,-0.5764837046542));
#49716=CARTESIAN_POINT('Ctrl Pts',(-3.525101679693,-1.279549436203,-0.6148066213208));
#49717=CARTESIAN_POINT('Ctrl Pts',(-3.748764103251,-0.10176595716,-0.6531295379875));
#49718=CARTESIAN_POINT('Ctrl Pts',(-3.58932947872,1.086417279432,-0.6914524546542));
#49719=CARTESIAN_POINT('Ctrl Pts',(-3.063090891592,2.163576391465,-0.7297753713208));
#49720=CARTESIAN_POINT('Ctrl Pts',(-2.223826185381,3.019633373288,-0.7680982879875));
#49721=CARTESIAN_POINT('Ctrl Pts',(-1.15730224823,3.567105285536,-0.8064212046542));
#49722=CARTESIAN_POINT('Ctrl Pts',(0.02748975349761,3.750044389779,-0.8447441213208));
#49723=CARTESIAN_POINT('Ctrl Pts',(1.209472497793,3.549755609749,-0.8830670379875));
#49724=CARTESIAN_POINT('Ctrl Pts',(2.267855748792,2.98670703527,-0.9213899546542));
#49725=CARTESIAN_POINT('Ctrl Pts',(3.094480260398,2.118438228948,-0.9597128713208));
#49726=CARTESIAN_POINT('Ctrl Pts',(3.60487088252,1.033680091819,-0.9980357879875));
#49727=CARTESIAN_POINT('Ctrl Pts',(3.746869321032,-0.1567128041103,-1.036358704654));
#49728=CARTESIAN_POINT('Ctrl Pts',(3.505964344731,-1.331090765251,-1.074681621321));
#49729=CARTESIAN_POINT('Ctrl Pts',(2.906774730033,-2.369440710527,-1.113004537988));
#49730=CARTESIAN_POINT('Ctrl Pts',(2.010533396991,-3.165650655307,-1.151327454654));
#49731=CARTESIAN_POINT('Ctrl Pts',(0.908829840065,-3.638353602066,-1.189650371321));
#49732=CARTESIAN_POINT('Ctrl Pts',(-0.2857496672687,-3.739242669247,-1.227973287988));
#49733=CARTESIAN_POINT('Ctrl Pts',(-1.451127589491,-3.458007711223,-1.266296204654));
#49734=CARTESIAN_POINT('Ctrl Pts',(-2.46821058554,-2.823388941908,-1.304619121321));
#49735=CARTESIAN_POINT('Ctrl Pts',(-3.233060001844,-1.900239889155,-1.342942037988));
#49736=CARTESIAN_POINT('Ctrl Pts',(-3.667513664004,-0.7828998251401,-1.381264954654));
#49737=CARTESIAN_POINT('Ctrl Pts',(-3.727173495502,0.4144470367691,-1.419587871321));
#49738=CARTESIAN_POINT('Ctrl Pts',(-3.405942685574,1.569440357084,-1.457910787988));
#49739=CARTESIAN_POINT('Ctrl Pts',(-2.736648739939,2.564048027251,-1.496233704654));
#49740=CARTESIAN_POINT('Ctrl Pts',(-1.787688743027,3.296628212267,-1.534556621321));
#49741=CARTESIAN_POINT('Ctrl Pts',(-0.6560396620613,3.692316423827,-1.572879537988));
#49742=CARTESIAN_POINT('Ctrl Pts',(0.5426520097537,3.71067613895,-1.611202454654));
#49743=CARTESIAN_POINT('Ctrl Pts',(1.685888502915,3.349831125236,-1.649525371321));
#49744=CARTESIAN_POINT('Ctrl Pts',(2.656839173046,2.646657178484,-1.687848287988));
#49745=CARTESIAN_POINT('Ctrl Pts',(3.356279762414,1.673013678449,-1.726171204654));
#49746=CARTESIAN_POINT('Ctrl Pts',(3.712732413852,0.5284000709324,-1.764494121321));
#49747=CARTESIAN_POINT('Ctrl Pts',(3.689770199791,-0.670212268354,-1.802817037988));
#49748=CARTESIAN_POINT('Ctrl Pts',(3.289739695226,-1.800333677259,-1.841139954654));
#49749=CARTESIAN_POINT('Ctrl Pts',(2.553521174936,-2.746473779316,-1.879462871321));
#49750=CARTESIAN_POINT('Ctrl Pts',(1.55635093806,-3.411943782343,-1.917785787988));
#49751=CARTESIAN_POINT('Ctrl Pts',(0.4001327000829,-3.728737374837,-1.956108704654));
#49752=CARTESIAN_POINT('Ctrl Pts',(-0.7969762688943,-3.66448052866,-1.994431621321));
#49753=CARTESIAN_POINT('Ctrl Pts',(-1.912639879403,-3.22573974165,-2.032754537988));
#49754=CARTESIAN_POINT('Ctrl Pts',(-2.832845467165,-2.457351559135,-2.071077454654));
#49755=CARTESIAN_POINT('Ctrl Pts',(-3.463553712324,-1.437838466947,-2.109400371321));
#49756=CARTESIAN_POINT('Ctrl Pts',(-3.740313882881,-0.2713924033866,-2.147723287988));
#49757=CARTESIAN_POINT('Ctrl Pts',(-3.634831232967,0.9228025934093,-2.186046204654));
#49758=CARTESIAN_POINT('Ctrl Pts',(-3.31689672123,1.656027125022,-2.211594815765));
#49759=CARTESIAN_POINT('Ctrl Pts',(-3.104121494422,1.988223291274,-2.224369121321));
#49760=CARTESIAN_POINT('Ctrl Pts',(-1.650568539745,-3.482361570092,0.1316169118147));
#49761=CARTESIAN_POINT('Ctrl Pts',(-2.023243116164,-3.305721402488,0.1188426062592));
#49762=CARTESIAN_POINT('Ctrl Pts',(-2.711315436469,-2.831797996164,0.09329399514806));
#49763=CARTESIAN_POINT('Ctrl Pts',(-3.466407702612,-1.83149436699,0.0549710784814));
#49764=CARTESIAN_POINT('Ctrl Pts',(-3.867241405631,-0.644032771561,0.01664816181473));
#49765=CARTESIAN_POINT('Ctrl Pts',(-3.872874898558,0.6092464701004,-0.02167475485194));
#49766=CARTESIAN_POINT('Ctrl Pts',(-3.482726929583,1.800264496766,-0.0599976715186));
#49767=CARTESIAN_POINT('Ctrl Pts',(-2.736669335086,2.80730843565,-0.09832058818527));
#49768=CARTESIAN_POINT('Ctrl Pts',(-1.710943500445,3.527465364644,-0.1366435048519));
#49769=CARTESIAN_POINT('Ctrl Pts',(-0.5103714226555,3.88714041451,-0.1749664215186));
#49770=CARTESIAN_POINT('Ctrl Pts',(0.7423569932556,3.849577337881,-0.2132893381853));
#49771=CARTESIAN_POINT('Ctrl Pts',(1.919221798925,3.418614817852,-0.2516122548519));
#49772=CARTESIAN_POINT('Ctrl Pts',(2.899955777496,2.638294160056,-0.2899351715186));
#49773=CARTESIAN_POINT('Ctrl Pts',(3.584334886092,1.588358590075,-0.3282580881853));
#49774=CARTESIAN_POINT('Ctrl Pts',(3.902420443991,0.3761040609753,-0.3665810048519));
#49775=CARTESIAN_POINT('Ctrl Pts',(3.821706367838,-0.8745856301006,-0.4049039215186));
#49776=CARTESIAN_POINT('Ctrl Pts',(3.350441062573,-2.035898885647,-0.4432268381853));
#49777=CARTESIAN_POINT('Ctrl Pts',(2.536784493009,-2.989157744647,-0.4815497548519));
#49778=CARTESIAN_POINT('Ctrl Pts',(1.463886577727,-3.636945926723,-0.5198726715186));
#49779=CARTESIAN_POINT('Ctrl Pts',(0.2413898583541,-3.913064083635,-0.5581955881853));
#49780=CARTESIAN_POINT('Ctrl Pts',(-1.005775188934,-3.789294902179,-0.5965185048519));
#49781=CARTESIAN_POINT('Ctrl Pts',(-2.15015716017,-3.278286713044,-0.6348414215186));
#49782=CARTESIAN_POINT('Ctrl Pts',(-3.074808351262,-2.432260921317,-0.6731643381853));
#49783=CARTESIAN_POINT('Ctrl Pts',(-3.685235982171,-1.337675350026,-0.7114872548519));
#49784=CARTESIAN_POINT('Ctrl Pts',(-3.919058687457,-0.1063888651061,-0.7498101715186));
#49785=CARTESIAN_POINT('Ctrl Pts',(-3.752381448469,1.1357698057,-0.7881330881853));
#49786=CARTESIAN_POINT('Ctrl Pts',(-3.20223749442,2.26186087452,-0.8264560048519));
#49787=CARTESIAN_POINT('Ctrl Pts',(-2.324847627423,3.156805837491,-0.8647789215186));
#49788=CARTESIAN_POINT('Ctrl Pts',(-1.209874856091,3.72914767996,-0.9031018381853));
#49789=CARTESIAN_POINT('Ctrl Pts',(0.02873852669669,3.920397133383,-0.9414247548519));
#49790=CARTESIAN_POINT('Ctrl Pts',(1.264415036307,3.71100986287,-0.9797476715186));
#49791=CARTESIAN_POINT('Ctrl Pts',(2.370877315672,3.122383759307,-1.018070588185));
#49792=CARTESIAN_POINT('Ctrl Pts',(3.235052783705,2.214672226988,-1.056393504852));
#49793=CARTESIAN_POINT('Ctrl Pts',(3.768628849452,1.080636933218,-1.094716421519));
#49794=CARTESIAN_POINT('Ctrl Pts',(3.91707783123,-0.1638317748112,-1.133039338185));
#49795=CARTESIAN_POINT('Ctrl Pts',(3.665229298162,-1.391558039842,-1.171362254852));
#49796=CARTESIAN_POINT('Ctrl Pts',(3.038820380385,-2.477076963299,-1.209685171519));
#49797=CARTESIAN_POINT('Ctrl Pts',(2.101865617276,-3.30945622622,-1.248008088185));
#49798=CARTESIAN_POINT('Ctrl Pts',(0.9501151264862,-3.80363258383,-1.286331004852));
#49799=CARTESIAN_POINT('Ctrl Pts',(-0.29873037756,-3.909104724598,-1.324653921519));
#49800=CARTESIAN_POINT('Ctrl Pts',(-1.51704776016,-3.615094145351,-1.362976838185));
#49801=CARTESIAN_POINT('Ctrl Pts',(-2.580333643652,-2.951646637691,-1.401299754852));
#49802=CARTESIAN_POINT('Ctrl Pts',(-3.379927767743,-1.986561821639,-1.439622671519));
#49803=CARTESIAN_POINT('Ctrl Pts',(-3.834117295836,-0.8184645063324,-1.477945588185));
#49804=CARTESIAN_POINT('Ctrl Pts',(-3.896487286181,0.4332740645197,-1.516268504852));
#49805=CARTESIAN_POINT('Ctrl Pts',(-3.560663969041,1.640735105349,-1.554591421519));
#49806=CARTESIAN_POINT('Ctrl Pts',(-2.860966100662,2.680524679464,-1.592914338185));
#49807=CARTESIAN_POINT('Ctrl Pts',(-1.868897830289,3.446383682398,-1.631237254852));
#49808=CARTESIAN_POINT('Ctrl Pts',(-0.6858414843143,3.860046767171,-1.669560171519));
#49809=CARTESIAN_POINT('Ctrl Pts',(0.5673029869357,3.879240506513,-1.707883088185));
#49810=CARTESIAN_POINT('Ctrl Pts',(1.762473124864,3.502003436675,-1.746206004852));
#49811=CARTESIAN_POINT('Ctrl Pts',(2.777531035702,2.766886505093,-1.784528921519));
#49812=CARTESIAN_POINT('Ctrl Pts',(3.508745015196,1.749013437542,-1.822851838185));
#49813=CARTESIAN_POINT('Ctrl Pts',(3.881390191529,0.5524036272767,-1.861174754852));
#49814=CARTESIAN_POINT('Ctrl Pts',(3.857384876171,-0.7006579076169,-1.899497671519));
#49815=CARTESIAN_POINT('Ctrl Pts',(3.439182241653,-1.882117184185,-1.937820588185));
#49816=CARTESIAN_POINT('Ctrl Pts',(2.669519625297,-2.871237460732,-1.976143504852));
#49817=CARTESIAN_POINT('Ctrl Pts',(1.627051075112,-3.566937676797,-2.014466421519));
#49818=CARTESIAN_POINT('Ctrl Pts',(0.4183094724568,-3.898122207644,-2.052789338185));
#49819=CARTESIAN_POINT('Ctrl Pts',(-0.8331803987343,-3.830946374675,-2.091112254852));
#49820=CARTESIAN_POINT('Ctrl Pts',(-1.999525104514,-3.37227497111,-2.129435171519));
#49821=CARTESIAN_POINT('Ctrl Pts',(-2.961532743202,-2.56898132577,-2.167758088185));
#49822=CARTESIAN_POINT('Ctrl Pts',(-3.62089208387,-1.503154954499,-2.206081004852));
#49823=CARTESIAN_POINT('Ctrl Pts',(-3.910224600105,-0.2837209082534,-2.244403921519));
#49824=CARTESIAN_POINT('Ctrl Pts',(-3.799950204561,0.9647226181484,-2.282726838185));
#49825=CARTESIAN_POINT('Ctrl Pts',(-3.467572926091,1.731255238321,-2.308275449296));
#49826=CARTESIAN_POINT('Ctrl Pts',(-3.245131988724,2.078542033497,-2.321049754852));
#49827=CARTESIAN_POINT('Ctrl Pts',(-1.72229057955,-3.633680384871,0.03493627828363));
#49828=CARTESIAN_POINT('Ctrl Pts',(-2.111158958383,-3.449364684366,0.02216197272807));
#49829=CARTESIAN_POINT('Ctrl Pts',(-2.829130037303,-2.954847917273,-0.003386638383041));
#49830=CARTESIAN_POINT('Ctrl Pts',(-3.617033275098,-1.911078164166,-0.04170955504971));
#49831=CARTESIAN_POINT('Ctrl Pts',(-4.035284377099,-0.6720178827305,-0.08003247171637));
#49832=CARTESIAN_POINT('Ctrl Pts',(-4.041162661802,0.6357200145352,-0.118355388383));
#49833=CARTESIAN_POINT('Ctrl Pts',(-3.634061620302,1.878491264566,-0.1566783050497));
#49834=CARTESIAN_POINT('Ctrl Pts',(-2.855585637111,2.929294213592,-0.1950012217164));
#49835=CARTESIAN_POINT('Ctrl Pts',(-1.785289009212,3.680744071466,-0.233324138383));
#49836=CARTESIAN_POINT('Ctrl Pts',(-0.5325485565397,4.056048056224,-0.2716470550497));
#49837=CARTESIAN_POINT('Ctrl Pts',(0.7746145799827,4.016852753843,-0.3099699717164));
#49838=CARTESIAN_POINT('Ctrl Pts',(2.002617610091,3.567163649446,-0.348292888383));
#49839=CARTESIAN_POINT('Ctrl Pts',(3.02596735393,2.752935772451,-0.3866158050497));
#49840=CARTESIAN_POINT('Ctrl Pts',(3.74008474027,1.65737742527,-0.4249387217164));
#49841=CARTESIAN_POINT('Ctrl Pts',(4.071992047763,0.3924468845434,-0.463261638383));
#49842=CARTESIAN_POINT('Ctrl Pts',(3.98777070848,-0.9125889385755,-0.5015845550497));
#49843=CARTESIAN_POINT('Ctrl Pts',(3.496027544726,-2.124364658137,-0.5399074717164));
#49844=CARTESIAN_POINT('Ctrl Pts',(2.647015212912,-3.119045407947,-0.578230388383));
#49845=CARTESIAN_POINT('Ctrl Pts',(1.527496739238,-3.794981884784,-0.6165533050497));
#49846=CARTESIAN_POINT('Ctrl Pts',(0.2518789550578,-4.08309818474,-0.6548762217164));
#49847=CARTESIAN_POINT('Ctrl Pts',(-1.049479068172,-3.953950869661,-0.693199138383));
#49848=CARTESIAN_POINT('Ctrl Pts',(-2.243587789505,-3.420737877273,-0.7315220550497));
#49849=CARTESIAN_POINT('Ctrl Pts',(-3.208417784407,-2.537949785738,-0.7698449717164));
#49850=CARTESIAN_POINT('Ctrl Pts',(-3.845370284649,-1.39580126385,-0.808167888383));
#49851=CARTESIAN_POINT('Ctrl Pts',(-4.089353271664,-0.1110117730522,-0.8464908050497));
#49852=CARTESIAN_POINT('Ctrl Pts',(-3.915433418218,1.185122331967,-0.8848137217164));
#49853=CARTESIAN_POINT('Ctrl Pts',(-3.341384097248,2.360145357575,-0.923136638383));
#49854=CARTESIAN_POINT('Ctrl Pts',(-2.425869069466,3.293978301694,-0.9614595550497));
#49855=CARTESIAN_POINT('Ctrl Pts',(-1.262447463952,3.891190074384,-0.9997824717164));
#49856=CARTESIAN_POINT('Ctrl Pts',(0.02998729989577,4.090749876987,-1.038105388383));
#49857=CARTESIAN_POINT('Ctrl Pts',(1.31935757482,3.872264115991,-1.07642830505));
#49858=CARTESIAN_POINT('Ctrl Pts',(2.473898882552,3.258060483344,-1.114751221716));
#49859=CARTESIAN_POINT('Ctrl Pts',(3.375625307013,2.310906225029,-1.153074138383));
#49860=CARTESIAN_POINT('Ctrl Pts',(3.932386816384,1.127593774617,-1.19139705505));
#49861=CARTESIAN_POINT('Ctrl Pts',(4.087286341429,-0.1709507455122,-1.229719971716));
#49862=CARTESIAN_POINT('Ctrl Pts',(3.824494251593,-1.452025314433,-1.268042888383));
#49863=CARTESIAN_POINT('Ctrl Pts',(3.170866030738,-2.584713216072,-1.30636580505));
#49864=CARTESIAN_POINT('Ctrl Pts',(2.19319783756,-3.453261797134,-1.344688721716));
#49865=CARTESIAN_POINT('Ctrl Pts',(0.9914004129074,-3.968911565595,-1.383011638383));
#49866=CARTESIAN_POINT('Ctrl Pts',(-0.3117110878513,-4.07896677995,-1.42133455505));
#49867=CARTESIAN_POINT('Ctrl Pts',(-1.582967930829,-3.772180579478,-1.459657471716));
#49868=CARTESIAN_POINT('Ctrl Pts',(-2.692456701765,-3.079904333473,-1.497980388383));
#49869=CARTESIAN_POINT('Ctrl Pts',(-3.526795533643,-2.072883754122,-1.53630330505));
#49870=CARTESIAN_POINT('Ctrl Pts',(-4.000720927668,-0.8540291875248,-1.574626221716));
#49871=CARTESIAN_POINT('Ctrl Pts',(-4.06580107686,0.4521010922702,-1.612949138383));
#49872=CARTESIAN_POINT('Ctrl Pts',(-3.715385252509,1.712029853614,-1.65127205505));
#49873=CARTESIAN_POINT('Ctrl Pts',(-2.985283461384,2.797001331678,-1.689594971716));
#49874=CARTESIAN_POINT('Ctrl Pts',(-1.95010691755,3.596139152528,-1.727917888383));
#49875=CARTESIAN_POINT('Ctrl Pts',(-0.7156433065674,4.027777110515,-1.76624080505));
#49876=CARTESIAN_POINT('Ctrl Pts',(0.5919539641177,4.047804874075,-1.804563721716));
#49877=CARTESIAN_POINT('Ctrl Pts',(1.839057746813,3.654175748115,-1.842886638383));
#49878=CARTESIAN_POINT('Ctrl Pts',(2.898222898357,2.887115831701,-1.88120955505));
#49879=CARTESIAN_POINT('Ctrl Pts',(3.661210267978,1.825013196635,-1.919532471716));
#49880=CARTESIAN_POINT('Ctrl Pts',(4.050047969205,0.5764071836211,-1.957855388383));
#49881=CARTESIAN_POINT('Ctrl Pts',(4.024999552551,-0.7311035468799,-1.99617830505));
#49882=CARTESIAN_POINT('Ctrl Pts',(3.588624788081,-1.963900691111,-2.034501221716));
#49883=CARTESIAN_POINT('Ctrl Pts',(2.785518075659,-2.996001142148,-2.072824138383));
#49884=CARTESIAN_POINT('Ctrl Pts',(1.697751212165,-3.72193157125,-2.11114705505));
#49885=CARTESIAN_POINT('Ctrl Pts',(0.4364862448306,-4.067507040451,-2.149469971716));
#49886=CARTESIAN_POINT('Ctrl Pts',(-0.8693845285744,-3.997412220691,-2.187792888383));
#49887=CARTESIAN_POINT('Ctrl Pts',(-2.086410329625,-3.518810200571,-2.22611580505));
#49888=CARTESIAN_POINT('Ctrl Pts',(-3.090220019238,-2.680611092404,-2.264438721716));
#49889=CARTESIAN_POINT('Ctrl Pts',(-3.778230455416,-1.568471442051,-2.302761638383));
#49890=CARTESIAN_POINT('Ctrl Pts',(-4.080135317328,-0.2960494131202,-2.34108455505));
#49891=CARTESIAN_POINT('Ctrl Pts',(-3.965069176156,1.006642642887,-2.379407471716));
#49892=CARTESIAN_POINT('Ctrl Pts',(-3.618249130952,1.80648335162,-2.404956082827));
#49893=CARTESIAN_POINT('Ctrl Pts',(-3.386142483025,2.16886077572,-2.417730388383));
#49894=CARTESIAN_POINT('Ctrl Pts',(-0.264621262814254,3.52921885147511,
9.97465998686664E-17));
#49895=CARTESIAN_POINT('Ctrl Pts',(-0.0628839596244878,3.54453750585823,
-0.00696552242425897));
#49896=CARTESIAN_POINT('Ctrl Pts',(0.140163183717197,3.5427563049603,-0.0140558818516256));
#49897=CARTESIAN_POINT('Ctrl Pts',(0.537930260474703,3.50455590115915,-0.0276799019954263));
#49898=CARTESIAN_POINT('Ctrl Pts',(0.731295751643366,3.46899592207308,-0.0341038307636699));
#49899=CARTESIAN_POINT('Ctrl Pts',(1.18992431903622,3.34465894772215,-0.0497494988331141));
#49900=CARTESIAN_POINT('Ctrl Pts',(1.45082056278735,3.23973099148587,-0.0589569369225457));
#49901=CARTESIAN_POINT('Ctrl Pts',(1.85066944756859,3.02196767273769,-0.074569370893028));
#49902=CARTESIAN_POINT('Ctrl Pts',(1.99916397088873,2.92629851593253,-0.0807773580080322));
#49903=CARTESIAN_POINT('Ctrl Pts',(2.33657049127287,2.67098235688989,-0.0953838985417922));
#49904=CARTESIAN_POINT('Ctrl Pts',(2.51563975010642,2.50232952935312,-0.103322805181874));
#49905=CARTESIAN_POINT('Ctrl Pts',(2.89132158504577,2.06707630387109,-0.122258745710041));
#49906=CARTESIAN_POINT('Ctrl Pts',(3.07220853647605,1.78722204088807,-0.133388652163895));
#49907=CARTESIAN_POINT('Ctrl Pts',(3.26863809705789,1.36506427924163,-0.149476363944854));
#49908=CARTESIAN_POINT('Ctrl Pts',(3.31886051343565,1.23867187327451,-0.15422876836737));
#49909=CARTESIAN_POINT('Ctrl Pts',(3.42440714161648,0.919690468397073,-0.165734443856275));
#49910=CARTESIAN_POINT('Ctrl Pts',(3.47036487208215,0.725128900568946,-0.172214871389973));
#49911=CARTESIAN_POINT('Ctrl Pts',(3.56835533108999,0.0691126171902604,
-0.19388016863945));
#49912=CARTESIAN_POINT('Ctrl Pts',(3.54693882903862,-0.404113247195594,
-0.210083038142292));
#49913=CARTESIAN_POINT('Ctrl Pts',(3.3815526767447,-1.07111787131278,-0.233641822018199));
#49914=CARTESIAN_POINT('Ctrl Pts',(3.30723990028449,-1.28082280745294,-0.240907680301654));
#49915=CARTESIAN_POINT('Ctrl Pts',(3.13654495041243,-1.64967350595082,-0.254212335744979));
#49916=CARTESIAN_POINT('Ctrl Pts',(3.04561017614116,-1.8117263716817,-0.260318688146977));
#49917=CARTESIAN_POINT('Ctrl Pts',(2.83566095862384,-2.12627105633583,-0.273207769133487));
#49918=CARTESIAN_POINT('Ctrl Pts',(2.71559024311982,-2.27814918203614,-0.279941531425139));
#49919=CARTESIAN_POINT('Ctrl Pts',(2.24807694153657,-2.77904914090722,-0.30358438205821));
#49920=CARTESIAN_POINT('Ctrl Pts',(1.90488533547708,-2.99649843384656,-0.316427980546006));
#49921=CARTESIAN_POINT('Ctrl Pts',(1.4395827853575,-3.24171823576112,-0.333888702007015));
#49922=CARTESIAN_POINT('Ctrl Pts',(1.2156718830087,-3.33243065426894,-0.342144528390505));
#49923=CARTESIAN_POINT('Ctrl Pts',(0.814386518254699,-3.44939286173748,
-0.356681912885287));
#49924=CARTESIAN_POINT('Ctrl Pts',(0.639761851128878,-3.48637026674257,
-0.362848739836552));
#49925=CARTESIAN_POINT('Ctrl Pts',(0.242142474236125,-3.53855715483033,
-0.376181945411191));
#49926=CARTESIAN_POINT('Ctrl Pts',(0.0189572614360934,-3.54624657594503,
-0.383406933058502));
#49927=CARTESIAN_POINT('Ctrl Pts',(-0.501721552977363,-3.51578977434586,
-0.400737723420411));
#49928=CARTESIAN_POINT('Ctrl Pts',(-0.798405890422845,-3.4608651947752,
-0.410936210186359));
#49929=CARTESIAN_POINT('Ctrl Pts',(-1.22248236323576,-3.32526349446763,
-0.426425182199499));
#49930=CARTESIAN_POINT('Ctrl Pts',(-1.35899635127016,-3.27209778442608,
-0.431497732221111));
#49931=CARTESIAN_POINT('Ctrl Pts',(-1.69319085004253,-3.11658737782817,
-0.443814152235949));
#49932=CARTESIAN_POINT('Ctrl Pts',(-1.885321005712,-3.00362704783803,-0.450919958514229));
#49933=CARTESIAN_POINT('Ctrl Pts',(-2.25657862337976,-2.73620836477243,
-0.466129897694596));
#49934=CARTESIAN_POINT('Ctrl Pts',(-2.4342404980128,-2.57956481057542,-0.474160506718203));
#49935=CARTESIAN_POINT('Ctrl Pts',(-2.70406189805077,-2.28955596887064,
-0.487792479856233));
#49936=CARTESIAN_POINT('Ctrl Pts',(-2.80544632573569,-2.16466540561564,
-0.49337996726572));
#49937=CARTESIAN_POINT('Ctrl Pts',(-2.99824473911775,-1.8903161208689,-0.504873700329334));
#49938=CARTESIAN_POINT('Ctrl Pts',(-3.08734956143078,-1.74034849548728,
-0.510607146388673));
#49939=CARTESIAN_POINT('Ctrl Pts',(-3.26280650869878,-1.38854699351263,
-0.523458372993033));
#49940=CARTESIAN_POINT('Ctrl Pts',(-3.34246103011777,-1.18313932074248,
-0.530653117795877));
#49941=CARTESIAN_POINT('Ctrl Pts',(-3.51952274767331,-0.564154050130049,
-0.55258135924146));
#49942=CARTESIAN_POINT('Ctrl Pts',(-3.56446029553434,-0.141118654756757,
-0.567315278982563));
#49943=CARTESIAN_POINT('Ctrl Pts',(-3.49980016274106,0.618806706849648,
-0.592438540955659));
#49944=CARTESIAN_POINT('Ctrl Pts',(-3.42730365233934,0.939281313760002,
-0.60307473140123));
#49945=CARTESIAN_POINT('Ctrl Pts',(-3.26608986447908,1.37020091188365,-0.618977520143229));
#49946=CARTESIAN_POINT('Ctrl Pts',(-3.21174510953929,1.49373408262001,-0.623681838734362));
#49947=CARTESIAN_POINT('Ctrl Pts',(-3.04741893366169,1.81570525962115,-0.636158761370165));
#49948=CARTESIAN_POINT('Ctrl Pts',(-2.9257895372206,2.00554947617206,-0.643596937937371));
#49949=CARTESIAN_POINT('Ctrl Pts',(-2.59971973293075,2.42026758161057,-0.660980962533989));
#49950=CARTESIAN_POINT('Ctrl Pts',(-2.38301884184684,2.63344370490353,-0.670916530448369));
#49951=CARTESIAN_POINT('Ctrl Pts',(-2.02680985593994,2.90515541357183,-0.68627707144474));
#49952=CARTESIAN_POINT('Ctrl Pts',(-1.904778192232,2.98691191652053,-0.691416716240337));
#49953=CARTESIAN_POINT('Ctrl Pts',(-1.65582899649891,3.13202153163874,-0.701409064104142));
#49954=CARTESIAN_POINT('Ctrl Pts',(-1.52943609357706,3.19578772470759,-0.706229864017868));
#49955=CARTESIAN_POINT('Ctrl Pts',(-1.2247541139607,3.32652713538526,-0.717189889421697));
#49956=CARTESIAN_POINT('Ctrl Pts',(-1.04459023891923,3.38699095830953,-0.723323530969576));
#49957=CARTESIAN_POINT('Ctrl Pts',(-0.703648151102374,3.47206498648711,
-0.734996960808483));
#49958=CARTESIAN_POINT('Ctrl Pts',(-0.54381980803693,3.50061073469892,-0.7404478038163));
#49959=CARTESIAN_POINT('Ctrl Pts',(-0.201816646292843,3.53808128149046,
-0.75216257198571));
#49960=CARTESIAN_POINT('Ctrl Pts',(-0.0192726672086005,3.54413123318279,
-0.758464403158838));
#49961=CARTESIAN_POINT('Ctrl Pts',(0.279013422284102,3.53083955973339,-0.768819141221532));
#49962=CARTESIAN_POINT('Ctrl Pts',(0.395202241640959,3.51985650823388,-0.772836829640794));
#49963=CARTESIAN_POINT('Ctrl Pts',(0.715918597103892,3.47290766543585,-0.783688019912121));
#49964=CARTESIAN_POINT('Ctrl Pts',(0.918166422680317,3.42449853694842,-0.790336205147484));
#49965=CARTESIAN_POINT('Ctrl Pts',(1.4060534825555,3.26194416863173,-0.807309072604764));
#49966=CARTESIAN_POINT('Ctrl Pts',(1.6850516524377,3.12729642735548,-0.817931124258926));
#49967=CARTESIAN_POINT('Ctrl Pts',(2.11188424682707,2.84815909807049,-0.835521831524876));
#49968=CARTESIAN_POINT('Ctrl Pts',(2.27163940152376,2.72279877301433,-0.842487526307453));
#49969=CARTESIAN_POINT('Ctrl Pts',(2.56828037414233,2.44417699117511,-0.855978783114457));
#49970=CARTESIAN_POINT('Ctrl Pts',(2.70409644770606,2.29234856385226,-0.862545586637578));
#49971=CARTESIAN_POINT('Ctrl Pts',(2.9783319322613,1.92792828456862,-0.877658875229771));
#49972=CARTESIAN_POINT('Ctrl Pts',(3.10917461242445,1.70948764113348,-0.88644525581145));
#49973=CARTESIAN_POINT('Ctrl Pts',(3.28156155473456,1.33648233396227,-0.900674479468243));
#49974=CARTESIAN_POINT('Ctrl Pts',(3.33827373145222,1.18862719992309,-0.906118956223986));
#49975=CARTESIAN_POINT('Ctrl Pts',(3.46604468842926,0.771341027127037,-0.920739709652885));
#49976=CARTESIAN_POINT('Ctrl Pts',(3.5152914165801,0.495653409739684,-0.92976852882634));
#49977=CARTESIAN_POINT('Ctrl Pts',(3.54713653941856,-0.0251639221401792,
-0.947125291843253));
#49978=CARTESIAN_POINT('Ctrl Pts',(3.53724452475388,-0.269969014214833,
-0.955525192271259));
#49979=CARTESIAN_POINT('Ctrl Pts',(3.47766425068042,-0.682888166898913,
-0.970034433472272));
#49980=CARTESIAN_POINT('Ctrl Pts',(3.44021364964715,-0.853007512381875,
-0.976029608802391));
#49981=CARTESIAN_POINT('Ctrl Pts',(3.3603394377886,-1.11773024116344,-0.985196670383434));
#49982=CARTESIAN_POINT('Ctrl Pts',(3.32660260203798,-1.2139929586542,-0.988524242567791));
#49983=CARTESIAN_POINT('Ctrl Pts',(3.16270045761105,-1.62398848765727,-1.00303684624274));
#49984=CARTESIAN_POINT('Ctrl Pts',(2.99112197174943,-1.9213472066483,-1.01437016184374));
#49985=CARTESIAN_POINT('Ctrl Pts',(2.71916743299541,-2.26801202614191,-1.02956577508448));
#49986=CARTESIAN_POINT('Ctrl Pts',(2.65345479161002,-2.34482230175402,-1.03309011572484));
#49987=CARTESIAN_POINT('Ctrl Pts',(2.51938354394797,-2.48850592178276,-1.03991233786383));
#49988=CARTESIAN_POINT('Ctrl Pts',(2.45136413252933,-2.55568782031447,-1.04320973142055));
#49989=CARTESIAN_POINT('Ctrl Pts',(2.30984422638263,-2.68428307531518,-1.04966261566972));
#49990=CARTESIAN_POINT('Ctrl Pts',(2.23634923922314,-2.74567398495228,-1.05281737552517));
#49991=CARTESIAN_POINT('Ctrl Pts',(2.03215211779958,-2.90253737468983,-1.06124771713154));
#49992=CARTESIAN_POINT('Ctrl Pts',(1.89702757004923,-2.9922375826466,-1.06650485891362));
#49993=CARTESIAN_POINT('Ctrl Pts',(1.5646930096777,-3.18182032056654,-1.07925869521061));
#49994=CARTESIAN_POINT('Ctrl Pts',(1.36273027274016,-3.27353529473883,-1.08679861770155));
#49995=CARTESIAN_POINT('Ctrl Pts',(0.945261046853487,-3.41821874298324,
-1.10200645884336));
#49996=CARTESIAN_POINT('Ctrl Pts',(0.729224280881415,-3.47132276863424,
-1.10976827570799));
#49997=CARTESIAN_POINT('Ctrl Pts',(0.382914472640594,-3.52143416142455,
-1.12149300683948));
#49998=CARTESIAN_POINT('Ctrl Pts',(0.255792931202741,-3.53272173764504,
-1.12566442134657));
#49999=CARTESIAN_POINT('Ctrl Pts',(-0.113062510410115,-3.54552346686426,
-1.1377289345704));
#50000=CARTESIAN_POINT('Ctrl Pts',(-0.355466351724561,-3.52922066711232,
-1.1457225507509));
#50001=CARTESIAN_POINT('Ctrl Pts',(-0.871408743345329,-3.44181384528943,
-1.16366965067737));
#50002=CARTESIAN_POINT('Ctrl Pts',(-1.25970345812106,-3.34412341778873,
-1.17754107965305));
#50003=CARTESIAN_POINT('Ctrl Pts',(-1.96907530071397,-2.95845149470074,
-1.20416008647879));
#50004=CARTESIAN_POINT('Ctrl Pts',(-2.23116543632206,-2.76560410716815,
-1.21467297486572));
#50005=CARTESIAN_POINT('Ctrl Pts',(-2.67889924966404,-2.3327143711385,-1.23617432834315));
#50006=CARTESIAN_POINT('Ctrl Pts',(-2.86897605883321,-2.09628119776566,
-1.24672137384146));
#50007=CARTESIAN_POINT('Ctrl Pts',(-3.23973759783859,-1.48375590216976,
-1.27035024270255));
#50008=CARTESIAN_POINT('Ctrl Pts',(-3.3907973744537,-1.09307272587653,-1.28385141224157));
#50009=CARTESIAN_POINT('Ctrl Pts',(-3.52039460900459,-0.444742011367405,
-1.30674376705023));
#50010=CARTESIAN_POINT('Ctrl Pts',(-3.54367240627609,-0.195348451110837,
-1.31550126057737));
#50011=CARTESIAN_POINT('Ctrl Pts',(-3.53684555370509,0.212912125235389,
-1.32897516991721));
#50012=CARTESIAN_POINT('Ctrl Pts',(-3.52355723814933,0.370013095177801,
-1.33406889946687));
#50013=CARTESIAN_POINT('Ctrl Pts',(-3.44969917731903,0.857382716286607,
-1.35037352970638));
#50014=CARTESIAN_POINT('Ctrl Pts',(-3.35257804579177,1.18233803551094,-1.36182222496779));
#50015=CARTESIAN_POINT('Ctrl Pts',(-3.13714253384444,1.64961323241961,-1.37965155151134));
#50016=CARTESIAN_POINT('Ctrl Pts',(-3.04995817443986,1.80621222613115,-1.38584433097576));
#50017=CARTESIAN_POINT('Ctrl Pts',(-2.86678237182935,2.08189311977124,-1.39681812337178));
#50018=CARTESIAN_POINT('Ctrl Pts',(-2.77501506247927,2.20224713487007,-1.40170864192018));
#50019=CARTESIAN_POINT('Ctrl Pts',(-2.52332435703554,2.4922024096765,-1.41429807105808));
#50020=CARTESIAN_POINT('Ctrl Pts',(-2.3533714407419,2.65319226270889,-1.42219795278603));
#50021=CARTESIAN_POINT('Ctrl Pts',(-1.94386074828543,2.97168356561673,-1.44004191719084));
#50022=CARTESIAN_POINT('Ctrl Pts',(-1.61491480619346,3.18591725044698,-1.45353899697759));
#50023=CARTESIAN_POINT('Ctrl Pts',(-0.931878180439088,3.42331584633322,
-1.47725256485255));
#50024=CARTESIAN_POINT('Ctrl Pts',(-0.687664090142368,3.48031865812463,
-1.48542548426783));
#50025=CARTESIAN_POINT('Ctrl Pts',(-0.23381657008611,3.53756006465768,-1.5011152849445));
#50026=CARTESIAN_POINT('Ctrl Pts',(-0.0250415350069334,3.54563700299522,
-1.50841344094553));
#50027=CARTESIAN_POINT('Ctrl Pts',(0.393004384983738,3.52452247866436,-1.52275874360842));
#50028=CARTESIAN_POINT('Ctrl Pts',(0.600418503567333,3.49485515022846,-1.52965062013704));
#50029=CARTESIAN_POINT('Ctrl Pts',(1.09736162060221,3.37808155014134,-1.54646887836633));
#50030=CARTESIAN_POINT('Ctrl Pts',(1.38189734762745,3.27171292848107,-1.55637931072981));
#50031=CARTESIAN_POINT('Ctrl Pts',(1.83090116723113,3.03603789251927,-1.57387390694066));
#50032=CARTESIAN_POINT('Ctrl Pts',(2.00495491799037,2.92459539548152,-1.5811428566297));
#50033=CARTESIAN_POINT('Ctrl Pts',(2.26124338011125,2.72628632279553,-1.59214069984753));
#50034=CARTESIAN_POINT('Ctrl Pts',(2.35063802083803,2.6494228731033,-1.59601970029676));
#50035=CARTESIAN_POINT('Ctrl Pts',(2.56968967832108,2.44106535281573,-1.60593120010558));
#50036=CARTESIAN_POINT('Ctrl Pts',(2.69343555017507,2.30325658977076,-1.612006418483));
#50037=CARTESIAN_POINT('Ctrl Pts',(2.90788195749299,2.02387010049144,-1.62377075774636));
#50038=CARTESIAN_POINT('Ctrl Pts',(3.00061309371375,1.88377651487001,-1.62943608992525));
#50039=CARTESIAN_POINT('Ctrl Pts',(3.18893853513039,1.55064596016399,-1.64255846538333));
#50040=CARTESIAN_POINT('Ctrl Pts',(3.27789892378502,1.35382466996276,-1.65016296159083));
#50041=CARTESIAN_POINT('Ctrl Pts',(3.38230914293851,1.05022243547603,-1.6610576833713));
#50042=CARTESIAN_POINT('Ctrl Pts',(3.41206848626365,0.948630213858275,-1.66455192322864));
#50043=CARTESIAN_POINT('Ctrl Pts',(3.47298243877771,0.699597302697179,-1.67294935037395));
#50044=CARTESIAN_POINT('Ctrl Pts',(3.4993656521765,0.550889227730839,-1.67783645953324));
#50045=CARTESIAN_POINT('Ctrl Pts',(3.53894438372914,0.200661876798343,-1.68954796717138));
#50046=CARTESIAN_POINT('Ctrl Pts',(3.54466152137657,-0.00176295551019043,
-1.69641644230088));
#50047=CARTESIAN_POINT('Ctrl Pts',(3.51829273772974,-0.470493168757712,
-1.71254294048661));
#50048=CARTESIAN_POINT('Ctrl Pts',(3.47318172667174,-0.736754365994446,
-1.72196428124109));
#50049=CARTESIAN_POINT('Ctrl Pts',(3.35537223945156,-1.1373018398422,-1.73588382755945));
#50050=CARTESIAN_POINT('Ctrl Pts',(3.30479181397498,-1.27604640284775,-1.74068350078129));
#50051=CARTESIAN_POINT('Ctrl Pts',(3.16718492377856,-1.5912926594912,-1.7519417711377));
#50052=CARTESIAN_POINT('Ctrl Pts',(3.07361638980968,-1.76497580390325,-1.75848191075209));
#50053=CARTESIAN_POINT('Ctrl Pts',(2.84022721222543,-2.12424226662904,-1.77315559437722));
#50054=CARTESIAN_POINT('Ctrl Pts',(2.69505456286334,-2.30646539287088,-1.78126768471401));
#50055=CARTESIAN_POINT('Ctrl Pts',(2.37886712768591,-2.63106917496356,-1.79674409493971));
#50056=CARTESIAN_POINT('Ctrl Pts',(2.21036711097651,-2.7735214089575,-1.80399408546808));
#50057=CARTESIAN_POINT('Ctrl Pts',(1.84475102259879,-3.02869423119426,-1.81865031742086));
#50058=CARTESIAN_POINT('Ctrl Pts',(1.64685580303852,-3.14046009135748,-1.82608516870827));
#50059=CARTESIAN_POINT('Ctrl Pts',(1.30211229096659,-3.29435184719581,-1.83898859470103));
#50060=CARTESIAN_POINT('Ctrl Pts',(1.15999346675071,-3.34730451232009,-1.84427863704171));
#50061=CARTESIAN_POINT('Ctrl Pts',(0.86236200010171,-3.43691606068077,-1.8550635325919));
#50062=CARTESIAN_POINT('Ctrl Pts',(0.70641438115456,-3.47258240326183,-1.86054104982383));
#50063=CARTESIAN_POINT('Ctrl Pts',(0.38245767886815,-3.52311089768784,-1.87141869044349));
#50064=CARTESIAN_POINT('Ctrl Pts',(0.215109285174395,-3.53692867125598,
-1.87689259850194));
#50065=CARTESIAN_POINT('Ctrl Pts',(-0.17080281501418,-3.54157104116341,
-1.88964570117501));
#50066=CARTESIAN_POINT('Ctrl Pts',(-0.389521567696692,-3.52412842824805,
-1.89693106052957));
#50067=CARTESIAN_POINT('Ctrl Pts',(-0.81192126987469,-3.45129306028026,
-1.91157065871698));
#50068=CARTESIAN_POINT('Ctrl Pts',(-1.01593935698251,-3.3973397238017,-1.91899733085867));
#50069=CARTESIAN_POINT('Ctrl Pts',(-1.37277482230161,-3.26748271910123,
-1.9320158250549));
#50070=CARTESIAN_POINT('Ctrl Pts',(-1.52685384876056,-3.19811464000463,
-1.93755148215728));
#50071=CARTESIAN_POINT('Ctrl Pts',(-1.94098593117999,-2.97477489628643,
-1.95292816354384));
#50072=CARTESIAN_POINT('Ctrl Pts',(-2.18841907487769,-2.7973238359502,-1.96302478119542));
#50073=CARTESIAN_POINT('Ctrl Pts',(-2.56405122407262,-2.44884668828753,
-1.98055727133914));
#50074=CARTESIAN_POINT('Ctrl Pts',(-2.70574308030546,-2.2920728130192,-1.98791057288492));
#50075=CARTESIAN_POINT('Ctrl Pts',(-2.93393460083031,-1.9881997954724,-2.00093313990393));
#50076=CARTESIAN_POINT('Ctrl Pts',(-3.0251948995756,-1.84580897732215,-2.00648843180739));
#50077=CARTESIAN_POINT('Ctrl Pts',(-3.22369794631868,-1.48125161922904,
-2.02004049934766));
#50078=CARTESIAN_POINT('Ctrl Pts',(-3.31897013566167,-1.25234888004105,
-2.02816089470863));
#50079=CARTESIAN_POINT('Ctrl Pts',(-3.51045751553196,-0.614887926350445,
-2.05091020117093));
#50080=CARTESIAN_POINT('Ctrl Pts',(-3.55967612642411,-0.202806351969069,
-2.06524896687874));
#50081=CARTESIAN_POINT('Ctrl Pts',(-3.52443018549891,0.351738831399751,
-2.08353960608183));
#50082=CARTESIAN_POINT('Ctrl Pts',(-3.50852296577055,0.483805038134683,
-2.08788020965693));
#50083=CARTESIAN_POINT('Ctrl Pts',(-3.48534270679742,0.614574670841336,
-2.09226952931372));
#50084=CARTESIAN_POINT('Ctrl Pts',(-3.93889502759575,0.69454040892368,-1.60816409353334));
#50085=CARTESIAN_POINT('Ctrl Pts',(-4.00744659720704,0.306810047460087,
-1.5964556824165));
#50086=CARTESIAN_POINT('Ctrl Pts',(-4.01838996798143,-0.0875683989890832,
-1.58502986037042));
#50087=CARTESIAN_POINT('Ctrl Pts',(-3.92470336328846,-0.861748316404742,
-1.56143896080034));
#50088=CARTESIAN_POINT('Ctrl Pts',(-3.82291771735831,-1.23664973539996,
-1.54999044876737));
#50089=CARTESIAN_POINT('Ctrl Pts',(-3.4330291644234,-2.13834145427003,-1.52095445657165));
#50090=CARTESIAN_POINT('Ctrl Pts',(-3.11045881151132,-2.54889752466793,
-1.50542478621335));
#50091=CARTESIAN_POINT('Ctrl Pts',(-2.63260132188013,-3.02171102766451,
-1.48532088310118));
#50092=CARTESIAN_POINT('Ctrl Pts',(-2.43650516808078,-3.18208186762214,
-1.47792778043916));
#50093=CARTESIAN_POINT('Ctrl Pts',(-2.0173198756678,-3.46319653213006,-1.46302039289925));
#50094=CARTESIAN_POINT('Ctrl Pts',(-1.79626338874197,-3.58272324890874,
-1.45544555299358));
#50095=CARTESIAN_POINT('Ctrl Pts',(-1.10823337490155,-3.87482660455011,
-1.43288939965075));
#50096=CARTESIAN_POINT('Ctrl Pts',(-0.584632652053741,-3.99691429971845,
-1.41746240937877));
#50097=CARTESIAN_POINT('Ctrl Pts',(0.233830615342959,-4.00127063912057,
-1.39303362854051));
#50098=CARTESIAN_POINT('Ctrl Pts',(0.490201285660078,-3.97777504144854,
-1.3852446142734));
#50099=CARTESIAN_POINT('Ctrl Pts',(0.995938468358567,-3.88222301582721,
-1.36976301914108));
#50100=CARTESIAN_POINT('Ctrl Pts',(1.24415481848043,-3.80995446145941,-1.36217322692837));
#50101=CARTESIAN_POINT('Ctrl Pts',(2.01616276652598,-3.50202694919009,-1.33766738862933));
#50102=CARTESIAN_POINT('Ctrl Pts',(2.44508081081143,-3.1987775444315,-1.32196010534453));
#50103=CARTESIAN_POINT('Ctrl Pts',(3.01090964362374,-2.65254240525115,-1.29850917321391));
#50104=CARTESIAN_POINT('Ctrl Pts',(3.21562175227277,-2.40092461921334,-1.28910836238346));
#50105=CARTESIAN_POINT('Ctrl Pts',(3.51776457715512,-1.91951785534438,-1.27214083111131));
#50106=CARTESIAN_POINT('Ctrl Pts',(3.62874538995318,-1.70001972408149,-1.26467049496387));
#50107=CARTESIAN_POINT('Ctrl Pts',(3.81427530798883,-1.23099921631057,-1.24950266268962));
#50108=CARTESIAN_POINT('Ctrl Pts',(3.88616447441406,-0.980605275840849,
-1.24185379598605));
#50109=CARTESIAN_POINT('Ctrl Pts',(4.04000254950994,-0.149723695797231,
-1.21688850567111));
#50110=CARTESIAN_POINT('Ctrl Pts',(4.00632467612848,0.370910426850598,-1.2013571473354));
#50111=CARTESIAN_POINT('Ctrl Pts',(3.86806721181153,1.04847228431323,-1.18068049877335));
#50112=CARTESIAN_POINT('Ctrl Pts',(3.79419777707799,1.29091995395088,-1.17327277042335));
#50113=CARTESIAN_POINT('Ctrl Pts',(3.60137912405081,1.75898868775722,-1.15832902502366));
#50114=CARTESIAN_POINT('Ctrl Pts',(3.48294709266645,1.98293492001914,-1.15069862141123));
#50115=CARTESIAN_POINT('Ctrl Pts',(3.0548197047919,2.63486504159509,-1.12714149943802));
#50116=CARTESIAN_POINT('Ctrl Pts',(2.67806842243565,3.01824425671164,-1.11173986731942));
#50117=CARTESIAN_POINT('Ctrl Pts',(2.02555902554214,3.45869156667143,-1.08823174530743));
#50118=CARTESIAN_POINT('Ctrl Pts',(1.79821101280998,3.58188217699888,-1.08041935974421));
#50119=CARTESIAN_POINT('Ctrl Pts',(1.32350112298141,3.78308453313687,-1.06491464450448));
#50120=CARTESIAN_POINT('Ctrl Pts',(1.07699975502504,3.86055113598766,-1.05732128114226));
#50121=CARTESIAN_POINT('Ctrl Pts',(0.270034970633146,4.03099324476181,-1.03301716956992));
#50122=CARTESIAN_POINT('Ctrl Pts',(-0.25521342163276,4.01927379572924,-1.01728840247899));
#50123=CARTESIAN_POINT('Ctrl Pts',(-0.969575955830072,3.88857553975101,
-0.995653688585681));
#50124=CARTESIAN_POINT('Ctrl Pts',(-1.2141204936574,3.81960306062729,-0.988196368037047));
#50125=CARTESIAN_POINT('Ctrl Pts',(-1.69005956293143,3.6345359373705,-0.973099649565625));
#50126=CARTESIAN_POINT('Ctrl Pts',(-1.91982443837823,3.51828148267251,-0.96534187309345));
#50127=CARTESIAN_POINT('Ctrl Pts',(-2.56734407205033,3.10884896953529,-0.942197836812912));
#50128=CARTESIAN_POINT('Ctrl Pts',(-2.94375611537857,2.75583749190019,-0.927474923905979));
#50129=CARTESIAN_POINT('Ctrl Pts',(-3.39474632506785,2.13146138471936,-0.904363755701564));
#50130=CARTESIAN_POINT('Ctrl Pts',(-3.52633862076298,1.90518052615191,-0.896498084751868));
#50131=CARTESIAN_POINT('Ctrl Pts',(-3.81701733888187,1.27167726524321,-0.875595295234326));
#50132=CARTESIAN_POINT('Ctrl Pts',(-3.93378242934524,0.8470632461161,-0.862985144367765));
#50133=CARTESIAN_POINT('Ctrl Pts',(-4.00531037533674,0.153415730762649,
-0.842014391062206));
#50134=CARTESIAN_POINT('Ctrl Pts',(-4.00669128945411,-0.106473790668588,
-0.834139140561101));
#50135=CARTESIAN_POINT('Ctrl Pts',(-3.95923793090611,-0.622498168961368,
-0.818673884785553));
#50136=CARTESIAN_POINT('Ctrl Pts',(-3.91077151366751,-0.87757469121337,
-0.811047443675081));
#50137=CARTESIAN_POINT('Ctrl Pts',(-3.67021024045104,-1.69994920328026,
-0.785678417398851));
#50138=CARTESIAN_POINT('Ctrl Pts',(-3.39667285554584,-2.1567657173322,-0.769744977442529));
#50139=CARTESIAN_POINT('Ctrl Pts',(-2.98848117293989,-2.66694605409314,
-0.750359967163677));
#50140=CARTESIAN_POINT('Ctrl Pts',(-2.84110394956172,-2.82358937989018,
-0.744090090057257));
#50141=CARTESIAN_POINT('Ctrl Pts',(-2.27902931600789,-3.33202863984671,
-0.721634326703568));
#50142=CARTESIAN_POINT('Ctrl Pts',(-1.84441618373233,-3.5758310320697,-0.706666416766861));
#50143=CARTESIAN_POINT('Ctrl Pts',(-1.19187027314479,-3.8268756418652,-0.685908318678602));
#50144=CARTESIAN_POINT('Ctrl Pts',(-0.940807050262362,-3.8965071798302,
-0.67830414500068));
#50145=CARTESIAN_POINT('Ctrl Pts',(-0.424690974184233,-3.9860202103712,
-0.662684597705209));
#50146=CARTESIAN_POINT('Ctrl Pts',(-0.160507741240573,-4.00514503561195,
-0.654654677364008));
#50147=CARTESIAN_POINT('Ctrl Pts',(0.575348473826228,-3.98607260123649,
-0.632522882400995));
#50148=CARTESIAN_POINT('Ctrl Pts',(1.08945400304019,-3.88946270876767,-0.61759417931966));
#50149=CARTESIAN_POINT('Ctrl Pts',(1.83869836786569,-3.56143102383145,-0.592975290336023));
#50150=CARTESIAN_POINT('Ctrl Pts',(2.06544258583032,-3.43467463037156,-0.585192721734639));
#50151=CARTESIAN_POINT('Ctrl Pts',(2.49249938480152,-3.13890819007588,-0.569691014274639));
#50152=CARTESIAN_POINT('Ctrl Pts',(2.69195657236367,-2.96992092695915,-0.562052898386223));
#50153=CARTESIAN_POINT('Ctrl Pts',(3.23006954478627,-2.41445773272655,-0.539181057923025));
#50154=CARTESIAN_POINT('Ctrl Pts',(3.51185084512747,-1.98068495502258,-0.52360957978045));
#50155=CARTESIAN_POINT('Ctrl Pts',(3.80248490305767,-1.26750730703816,-0.500829955845552));
#50156=CARTESIAN_POINT('Ctrl Pts',(3.87729712792385,-1.01744142158655,-0.493164240787644));
#50157=CARTESIAN_POINT('Ctrl Pts',(4.02178703311848,-0.270710889804952,
-0.470391292799232));
#50158=CARTESIAN_POINT('Ctrl Pts',(4.02404060158649,0.236036749392638,-0.455308717844116));
#50159=CARTESIAN_POINT('Ctrl Pts',(3.83723046698998,1.24543408126294,-0.425085309954019));
#50160=CARTESIAN_POINT('Ctrl Pts',(3.6410761923079,1.73528978493034,-0.409267017824708));
#50161=CARTESIAN_POINT('Ctrl Pts',(3.21563842321284,2.39261837548403,-0.385980583765538));
#50162=CARTESIAN_POINT('Ctrl Pts',(3.05262614733734,2.59791809202657,-0.378282010147998));
#50163=CARTESIAN_POINT('Ctrl Pts',(2.51419179749808,3.1530225884133,-0.355374898172946));
#50164=CARTESIAN_POINT('Ctrl Pts',(2.08897578758717,3.448816708814,-0.339775101775347));
#50165=CARTESIAN_POINT('Ctrl Pts',(1.38576623163163,3.76087087273643,-0.317085552566121));
#50166=CARTESIAN_POINT('Ctrl Pts',(1.1403400596281,3.8427213320877,-0.309499971617901));
#50167=CARTESIAN_POINT('Ctrl Pts',(0.640302589479629,3.95652511673326,-0.294066596827899));
#50168=CARTESIAN_POINT('Ctrl Pts',(0.387035608816613,3.98894608798221,-0.286398346866338));
#50169=CARTESIAN_POINT('Ctrl Pts',(-0.387353382741609,4.01460566729674,
-0.263207054571433));
#50170=CARTESIAN_POINT('Ctrl Pts',(-0.906894917014024,3.93085568448703,
-0.248159509078221));
#50171=CARTESIAN_POINT('Ctrl Pts',(-1.63898710819294,3.65756660871905,-0.224527674913839));
#50172=CARTESIAN_POINT('Ctrl Pts',(-1.87140434482678,3.54415532691843,-0.216784792169306));
#50173=CARTESIAN_POINT('Ctrl Pts',(-2.31212015321213,3.27387546319818,-0.201467507015652));
#50174=CARTESIAN_POINT('Ctrl Pts',(-2.51975552530336,3.11724623449951,-0.193856165457704));
#50175=CARTESIAN_POINT('Ctrl Pts',(-3.08001951418731,2.60137486340935,-0.171158479958212));
#50176=CARTESIAN_POINT('Ctrl Pts',(-3.38288713508128,2.1917199886369,-0.155880597428147));
#50177=CARTESIAN_POINT('Ctrl Pts',(-3.71095897582277,1.51361027607746,-0.133659141724757));
#50178=CARTESIAN_POINT('Ctrl Pts',(-3.79931632169689,1.27633127684376,-0.126271130958857));
#50179=CARTESIAN_POINT('Ctrl Pts',(-3.92575395302178,0.80241628054708,-0.111502977965752));
#50180=CARTESIAN_POINT('Ctrl Pts',(-3.96631179397013,0.56790459229602,-0.104302357156274));
#50181=CARTESIAN_POINT('Ctrl Pts',(-4.02113745954231,-0.095459444094893,
-0.0844081710650721));
#50182=CARTESIAN_POINT('Ctrl Pts',(-3.99676192186721,-0.62281133824077,
-0.0693130354409824));
#50183=CARTESIAN_POINT('Ctrl Pts',(-3.7320206379447,-1.46609048049094,-0.042674421078045));
#50184=CARTESIAN_POINT('Ctrl Pts',(-3.61863802768239,-1.72709802725838,
-0.034100228204948));
#50185=CARTESIAN_POINT('Ctrl Pts',(-3.33597966896508,-2.22537714393393,
-0.0171317201591535));
#50186=CARTESIAN_POINT('Ctrl Pts',(-3.16619428328731,-2.46144472839372,
-0.00869672167633724));
#50187=CARTESIAN_POINT('Ctrl Pts',(-2.97253925539568,-2.67651731155686,
-1.42199285337063E-5));
#50188=CARTESIAN_POINT('Ctrl Pts',(3.987069663918,0.522679131849,0.3152898013535));
#50189=CARTESIAN_POINT('Ctrl Pts',(4.075962269058,-0.1554061172176,0.2949890614009));
#50190=CARTESIAN_POINT('Ctrl Pts',(3.900091378894,-1.557010834613,0.2543875814958));
#50191=CARTESIAN_POINT('Ctrl Pts',(2.642948825861,-3.263519409944,0.193485361638));
#50192=CARTESIAN_POINT('Ctrl Pts',(0.7125717312084,-4.138558721235,0.1325831417803));
#50193=CARTESIAN_POINT('Ctrl Pts',(-1.399304475191,-3.959477965926,0.07168092192261));
#50194=CARTESIAN_POINT('Ctrl Pts',(-3.154752699231,-2.771828540526,0.01077870206489));
#50195=CARTESIAN_POINT('Ctrl Pts',(-4.106624282706,-0.8781447135099,-0.05012351779283));
#50196=CARTESIAN_POINT('Ctrl Pts',(-4.01245983409,1.23922042509,-0.1110257376505));
#50197=CARTESIAN_POINT('Ctrl Pts',(-2.896244687669,3.040932036188,-0.1719279575083));
#50198=CARTESIAN_POINT('Ctrl Pts',(-1.042300344905,4.068059861997,-0.232830177366));
#50199=CARTESIAN_POINT('Ctrl Pts',(1.077137937534,4.058974609329,-0.2937323972237));
#50200=CARTESIAN_POINT('Ctrl Pts',(2.922208477455,3.015990490368,-0.3546346170814));
#50201=CARTESIAN_POINT('Ctrl Pts',(4.022936335639,1.204775606403,-0.4155368369391));
#50202=CARTESIAN_POINT('Ctrl Pts',(4.098944963669,-0.9133187873028,-0.4764390567969));
#50203=CARTESIAN_POINT('Ctrl Pts',(3.130873502694,-2.798773326411,-0.5373412766546));
#50204=CARTESIAN_POINT('Ctrl Pts',(1.365308366059,-3.97132648973,-0.5982434965123));
#50205=CARTESIAN_POINT('Ctrl Pts',(-0.7480270609807,-4.132306442959,-0.65914571637));
#50206=CARTESIAN_POINT('Ctrl Pts',(-2.670825613937,-3.24070849698,-0.7200479362277));
#50207=CARTESIAN_POINT('Ctrl Pts',(-3.913313533437,-1.523639790607,-0.7809501560854));
#50208=CARTESIAN_POINT('Ctrl Pts',(-4.159005258158,0.5815292641248,-0.8418523759432));
#50209=CARTESIAN_POINT('Ctrl Pts',(-3.345318382176,2.538571634652,-0.9027545958009));
#50210=CARTESIAN_POINT('Ctrl Pts',(-1.679514596622,3.848991003293,-0.9636568156586));
#50211=CARTESIAN_POINT('Ctrl Pts',(0.4140938465922,4.178998361075,-1.024559035516));
#50212=CARTESIAN_POINT('Ctrl Pts',(2.402224628031,3.444534494857,-1.085461255374));
#50213=CARTESIAN_POINT('Ctrl Pts',(3.778462602443,1.832681451182,-1.146363475232));
#50214=CARTESIAN_POINT('Ctrl Pts',(4.192253539827,-0.2459907314392,-1.207265695089));
#50215=CARTESIAN_POINT('Ctrl Pts',(3.538196776895,-2.26200457673,-1.268167914947));
#50216=CARTESIAN_POINT('Ctrl Pts',(1.98289372813,-3.701841503134,-1.329070134805));
#50217=CARTESIAN_POINT('Ctrl Pts',(-0.07749218955726,-4.198751449836,-1.389972354663));
#50218=CARTESIAN_POINT('Ctrl Pts',(-2.118132963563,-3.626146647599,-1.45087457452));
#50219=CARTESIAN_POINT('Ctrl Pts',(-3.619268407771,-2.129937470376,-1.511776794378));
#50220=CARTESIAN_POINT('Ctrl Pts',(-4.198417559268,-0.09102472662167,-1.572679014236));
#50221=CARTESIAN_POINT('Ctrl Pts',(-3.871793425676,1.283290749965,-1.613280494141));
#50222=CARTESIAN_POINT('Ctrl Pts',(-3.550837736248,1.887185563384,-1.633581234094));
#50223=CARTESIAN_POINT('Ctrl Pts',(3.821034517157,0.5009129943895,0.2186091678224));
#50224=CARTESIAN_POINT('Ctrl Pts',(3.906225331763,-0.1489344777293,0.1983084278698));
#50225=CARTESIAN_POINT('Ctrl Pts',(3.737678303863,-1.492171605749,0.1577069479647));
#50226=CARTESIAN_POINT('Ctrl Pts',(2.532887444151,-3.127615357629,0.09680472810694));
#50227=CARTESIAN_POINT('Ctrl Pts',(0.6828978198043,-3.966215054687,0.03590250824922));
#50228=CARTESIAN_POINT('Ctrl Pts',(-1.341032675728,-3.794591831349,-0.0249997116085));
#50229=CARTESIAN_POINT('Ctrl Pts',(-3.023378062828,-2.656400168986,-0.08590193146621));
#50230=CARTESIAN_POINT('Ctrl Pts',(-3.935610474836,-0.8415757797628,-0.1468041513239));
#50231=CARTESIAN_POINT('Ctrl Pts',(-3.845367354253,1.187615070157,-0.2077063711817));
#50232=CARTESIAN_POINT('Ctrl Pts',(-2.775635204438,2.914297279467,-0.2686085910394));
#50233=CARTESIAN_POINT('Ctrl Pts',(-0.9988954121289,3.898652007819,-0.3295108108971));
#50234=CARTESIAN_POINT('Ctrl Pts',(1.032282248867,3.889945095985,-0.3904130307548));
#50235=CARTESIAN_POINT('Ctrl Pts',(2.800517773675,2.890394384479,-0.4513152506125));
#50236=CARTESIAN_POINT('Ctrl Pts',(3.855407578631,1.154604650919,-0.5122174704702));
#50237=CARTESIAN_POINT('Ctrl Pts',(3.928250948771,-0.8752850854435,-0.573119690328));
#50238=CARTESIAN_POINT('Ctrl Pts',(3.000493277283,-2.682222882307,-0.6340219101857));
#50239=CARTESIAN_POINT('Ctrl Pts',(1.308452280251,-3.805946942308,-0.6949241300434));
#50240=CARTESIAN_POINT('Ctrl Pts',(-0.7168766690086,-3.960223142552,-0.7558263499011));
#50241=CARTESIAN_POINT('Ctrl Pts',(-2.559603347921,-3.105754368695,-0.8167285697588));
#50242=CARTESIAN_POINT('Ctrl Pts',(-3.750349842903,-1.46019024556,-0.8776307896166));
#50243=CARTESIAN_POINT('Ctrl Pts',(-3.985810128244,0.5573124069205,-0.9385330094743));
#50244=CARTESIAN_POINT('Ctrl Pts',(-3.206007942338,2.432856874326,-0.999435229332));
#50245=CARTESIAN_POINT('Ctrl Pts',(-1.609573894291,3.688705921772,-1.06033744919));
#50246=CARTESIAN_POINT('Ctrl Pts',(0.3968495698709,4.004970650329,-1.121239669047));
#50247=CARTESIAN_POINT('Ctrl Pts',(2.30218782098,3.301092358505,-1.182141888905));
#50248=CARTESIAN_POINT('Ctrl Pts',(3.621114563505,1.756362359879,-1.243044108763));
#50249=CARTESIAN_POINT('Ctrl Pts',(4.017673838337,-0.2357468404016,-1.303946328621));
#50250=CARTESIAN_POINT('Ctrl Pts',(3.390854224434,-2.167807009712,-1.364848548478));
#50251=CARTESIAN_POINT('Ctrl Pts',(1.90031928652,-3.547684227473,-1.425750768336));
#50252=CARTESIAN_POINT('Ctrl Pts',(-0.07426515111787,-4.023901153264,-1.486652988194));
#50253=CARTESIAN_POINT('Ctrl Pts',(-2.029926700038,-3.475141563274,-1.547555208051));
#50254=CARTESIAN_POINT('Ctrl Pts',(-3.468549756755,-2.041239627024,-1.608457427909));
#50255=CARTESIAN_POINT('Ctrl Pts',(-4.023581167035,-0.08723414729463,-1.669359647767));
#50256=CARTESIAN_POINT('Ctrl Pts',(-3.710558773701,1.229850156756,-1.709961127672));
#50257=CARTESIAN_POINT('Ctrl Pts',(-3.402968771228,1.808596735399,-1.730261867625));
#50258=CARTESIAN_POINT('Ctrl Pts',(3.654999370396,0.4791468569299,0.1219285342913));
#50259=CARTESIAN_POINT('Ctrl Pts',(3.736488394468,-0.1424628382409,0.1016277943387));
#50260=CARTESIAN_POINT('Ctrl Pts',(3.575265228833,-1.427332376886,0.06102631443356));
#50261=CARTESIAN_POINT('Ctrl Pts',(2.422826062441,-2.991711305314,0.0001240945758373));
#50262=CARTESIAN_POINT('Ctrl Pts',(0.6532239084002,-3.79387138814,-0.06077812528188));
#50263=CARTESIAN_POINT('Ctrl Pts',(-1.282760876264,-3.629705696773,-0.1216803451396));
#50264=CARTESIAN_POINT('Ctrl Pts',(-2.892003426424,-2.540971797446,-0.1825825649973));
#50265=CARTESIAN_POINT('Ctrl Pts',(-3.764596666965,-0.8050068460156,-0.243484784855));
#50266=CARTESIAN_POINT('Ctrl Pts',(-3.678274874416,1.136009715224,-0.3043870047128));
#50267=CARTESIAN_POINT('Ctrl Pts',(-2.655025721206,2.787662522746,-0.3652892245705));
#50268=CARTESIAN_POINT('Ctrl Pts',(-0.9554904793529,3.729244153642,-0.4261914444282));
#50269=CARTESIAN_POINT('Ctrl Pts',(0.9874265601991,3.720915582642,-0.4870936642859));
#50270=CARTESIAN_POINT('Ctrl Pts',(2.678827069895,2.764798278589,-0.5479958841436));
#50271=CARTESIAN_POINT('Ctrl Pts',(3.687878821624,1.104433695434,-0.6088981040013));
#50272=CARTESIAN_POINT('Ctrl Pts',(3.757556933874,-0.8372513835842,-0.6698003238591));
#50273=CARTESIAN_POINT('Ctrl Pts',(2.870113051872,-2.565672438204,-0.7307025437168));
#50274=CARTESIAN_POINT('Ctrl Pts',(1.251596194444,-3.640567394886,-0.7916047635745));
#50275=CARTESIAN_POINT('Ctrl Pts',(-0.6857262770364,-3.788139842145,-0.8525069834322));
#50276=CARTESIAN_POINT('Ctrl Pts',(-2.448381081905,-2.97080024041,-0.9134092032899));
#50277=CARTESIAN_POINT('Ctrl Pts',(-3.58738615237,-1.396740700514,-0.9743114231477));
#50278=CARTESIAN_POINT('Ctrl Pts',(-3.81261499833,0.5330955497161,-1.035213643005));
#50279=CARTESIAN_POINT('Ctrl Pts',(-3.066697502499,2.327142114001,-1.096115862863));
#50280=CARTESIAN_POINT('Ctrl Pts',(-1.539633191959,3.52842084025,-1.157018082721));
#50281=CARTESIAN_POINT('Ctrl Pts',(0.3796052931495,3.830942939583,-1.217920302579));
#50282=CARTESIAN_POINT('Ctrl Pts',(2.202151013929,3.157650222153,-1.278822522436));
#50283=CARTESIAN_POINT('Ctrl Pts',(3.463766524566,1.680043268575,-1.339724742294));
#50284=CARTESIAN_POINT('Ctrl Pts',(3.843094136847,-0.2255029493641,-1.400626962152));
#50285=CARTESIAN_POINT('Ctrl Pts',(3.243511671973,-2.073609442694,-1.461529182009));
#50286=CARTESIAN_POINT('Ctrl Pts',(1.817744844909,-3.393526951812,-1.522431401867));
#50287=CARTESIAN_POINT('Ctrl Pts',(-0.07103811267848,-3.849050856693,-1.583333621725));
#50288=CARTESIAN_POINT('Ctrl Pts',(-1.941720436514,-3.324136478948,-1.644235841583));
#50289=CARTESIAN_POINT('Ctrl Pts',(-3.317831105739,-1.952541783671,-1.70513806144));
#50290=CARTESIAN_POINT('Ctrl Pts',(-3.848744774803,-0.08344356796759,-1.766040281298));
#50291=CARTESIAN_POINT('Ctrl Pts',(-3.549324121726,1.176409563546,-1.806641761203));
#50292=CARTESIAN_POINT('Ctrl Pts',(-3.255099806209,1.730007907414,-1.826942501156));
#50293=CARTESIAN_POINT('Ctrl Pts',(3.488964223634,0.4573807194704,0.02524790076017));
#50294=CARTESIAN_POINT('Ctrl Pts',(3.566751457173,-0.1359911987526,0.004947160807598));
#50295=CARTESIAN_POINT('Ctrl Pts',(3.412852153803,-1.362493148022,-0.03565431909755));
#50296=CARTESIAN_POINT('Ctrl Pts',(2.312764680731,-2.855807252999,-0.09655653895527));
#50297=CARTESIAN_POINT('Ctrl Pts',(0.6235499969961,-3.621527721592,-0.157458758813));
#50298=CARTESIAN_POINT('Ctrl Pts',(-1.224489076801,-3.464819562196,-0.2183609786707));
#50299=CARTESIAN_POINT('Ctrl Pts',(-2.760628790021,-2.425543425906,-0.2792631985284));
#50300=CARTESIAN_POINT('Ctrl Pts',(-3.593582859094,-0.7684379122684,-0.3401654183861));
#50301=CARTESIAN_POINT('Ctrl Pts',(-3.511182394579,1.084404360291,-0.4010676382439));
#50302=CARTESIAN_POINT('Ctrl Pts',(-2.534416237974,2.661027766025,-0.4619698581016));
#50303=CARTESIAN_POINT('Ctrl Pts',(-0.9120855465769,3.559836299465,-0.5228720779593));
#50304=CARTESIAN_POINT('Ctrl Pts',(0.9425708715315,3.551886069298,-0.583774297817));
#50305=CARTESIAN_POINT('Ctrl Pts',(2.557136366115,2.639202172699,-0.6446765176747));
#50306=CARTESIAN_POINT('Ctrl Pts',(3.520350064616,1.054262739949,-0.7055787375324));
#50307=CARTESIAN_POINT('Ctrl Pts',(3.586862918977,-0.799217681725,-0.7664809573902));
#50308=CARTESIAN_POINT('Ctrl Pts',(2.739732826461,-2.4491219941,-0.8273831772479));
#50309=CARTESIAN_POINT('Ctrl Pts',(1.194740108636,-3.475187847464,-0.8882853971056));
#50310=CARTESIAN_POINT('Ctrl Pts',(-0.6545758850643,-3.616056541738,-0.9491876169633));
#50311=CARTESIAN_POINT('Ctrl Pts',(-2.33715881589,-2.835846112125,-1.010089836821));
#50312=CARTESIAN_POINT('Ctrl Pts',(-3.424422461836,-1.333291155467,-1.070992056679));
#50313=CARTESIAN_POINT('Ctrl Pts',(-3.639419868416,0.5088786925118,-1.131894276536));
#50314=CARTESIAN_POINT('Ctrl Pts',(-2.92738706266,2.221427353675,-1.192796496394));
#50315=CARTESIAN_POINT('Ctrl Pts',(-1.469692489628,3.368135758728,-1.253698716252));
#50316=CARTESIAN_POINT('Ctrl Pts',(0.3623610164282,3.656915228838,-1.31460093611));
#50317=CARTESIAN_POINT('Ctrl Pts',(2.102114206878,3.0142080858,-1.375503155967));
#50318=CARTESIAN_POINT('Ctrl Pts',(3.306418485628,1.603724177272,-1.436405375825));
#50319=CARTESIAN_POINT('Ctrl Pts',(3.668514435358,-0.2152590583265,-1.497307595683));
#50320=CARTESIAN_POINT('Ctrl Pts',(3.096169119512,-1.979411875677,-1.558209815541));
#50321=CARTESIAN_POINT('Ctrl Pts',(1.735170403298,-3.239369676151,-1.619112035398));
#50322=CARTESIAN_POINT('Ctrl Pts',(-0.06781107423909,-3.674200560121,-1.680014255256));
#50323=CARTESIAN_POINT('Ctrl Pts',(-1.85351417299,-3.173131394623,-1.740916475114));
#50324=CARTESIAN_POINT('Ctrl Pts',(-3.167112454723,-1.863843940318,-1.801818694971));
#50325=CARTESIAN_POINT('Ctrl Pts',(-3.673908382571,-0.07965298864055,-1.862720914829));
#50326=CARTESIAN_POINT('Ctrl Pts',(-3.388089469752,1.122968970337,-1.903322394734));
#50327=CARTESIAN_POINT('Ctrl Pts',(-3.10723084119,1.651419079429,-1.923623134687));
#50328=CARTESIAN_POINT('Ctrl Pts',(3.47936545704605,-0.650670105535317,
-4.76018332824096E-10));
#50329=CARTESIAN_POINT('Ctrl Pts',(3.38968160510127,-1.13436012879633,-0.0163342927899063));
#50330=CARTESIAN_POINT('Ctrl Pts',(3.21731640401101,-1.5020431215797,-0.0305998613834371));
#50331=CARTESIAN_POINT('Ctrl Pts',(2.91462511544118,-2.03331814851161,-0.051072270408391));
#50332=CARTESIAN_POINT('Ctrl Pts',(2.71437316642751,-2.29491396340406,-0.0617505493407693));
#50333=CARTESIAN_POINT('Ctrl Pts',(2.31900078354353,-2.68463010998948,-0.0804698268472847));
#50334=CARTESIAN_POINT('Ctrl Pts',(2.14143413280956,-2.82773453209897,-0.0883278725496207));
#50335=CARTESIAN_POINT('Ctrl Pts',(1.75686408167297,-3.0810374614634,-0.103984992970782));
#50336=CARTESIAN_POINT('Ctrl Pts',(1.54943099477353,-3.19014995951601,-0.111846840226663));
#50337=CARTESIAN_POINT('Ctrl Pts',(1.00210135526143,-3.41325842701738,-0.131677489920045));
#50338=CARTESIAN_POINT('Ctrl Pts',(0.544373821935983,-3.54350905670246,
-0.147084119947701));
#50339=CARTESIAN_POINT('Ctrl Pts',(-0.357377907987189,-3.53673648881336,
-0.177838185184495));
#50340=CARTESIAN_POINT('Ctrl Pts',(-0.693343665582159,-3.48661654134669,
-0.189369643270235));
#50341=CARTESIAN_POINT('Ctrl Pts',(-1.16631985005951,-3.3457926319962,-0.205793243319711));
#50342=CARTESIAN_POINT('Ctrl Pts',(-1.31431715107854,-3.29078468383094,
-0.210902681306299));
#50343=CARTESIAN_POINT('Ctrl Pts',(-1.66823366960176,-3.13072836053275,
-0.223802193319174));
#50344=CARTESIAN_POINT('Ctrl Pts',(-1.86879091517682,-3.01462962777927,
-0.231756118939603));
#50345=CARTESIAN_POINT('Ctrl Pts',(-2.27584383075194,-2.72334336428232,
-0.249039274135891));
#50346=CARTESIAN_POINT('Ctrl Pts',(-2.47767451265281,-2.54136729640291,
-0.258366099123228));
#50347=CARTESIAN_POINT('Ctrl Pts',(-2.75400641105814,-2.22855213811819,
-0.272072041886219));
#50348=CARTESIAN_POINT('Ctrl Pts',(-2.84474988098196,-2.11194504812941,
-0.276775941565928));
#50349=CARTESIAN_POINT('Ctrl Pts',(-3.09280421483781,-1.74728848189743,
-0.291270929049092));
#50350=CARTESIAN_POINT('Ctrl Pts',(-3.22624023808558,-1.48418850547433,
-0.301617466166435));
#50351=CARTESIAN_POINT('Ctrl Pts',(-3.38896817920167,-1.03573903467768,
-0.318200875307344));
#50352=CARTESIAN_POINT('Ctrl Pts',(-3.43862282422981,-0.85697874637879,
-0.324545149882344));
#50353=CARTESIAN_POINT('Ctrl Pts',(-3.49480773816316,-0.570080244508614,
-0.334116350045796));
#50354=CARTESIAN_POINT('Ctrl Pts',(-3.510692569015,-0.463741682587342,-0.337557184422652));
#50355=CARTESIAN_POINT('Ctrl Pts',(-3.5322046936541,-0.254588229225586,
-0.344328485772883));
#50356=CARTESIAN_POINT('Ctrl Pts',(-3.53823753943844,-0.151825593456445,
-0.347657538444068));
#50357=CARTESIAN_POINT('Ctrl Pts',(-3.54240969027316,0.149585157253516,
-0.357706645183831));
#50358=CARTESIAN_POINT('Ctrl Pts',(-3.52796952112444,0.348330577797038,
-0.364700189646956));
#50359=CARTESIAN_POINT('Ctrl Pts',(-3.47646306433639,0.676052215094485,
-0.376361244191089));
#50360=CARTESIAN_POINT('Ctrl Pts',(-3.44841356490036,0.806462723056864,
-0.381034515032509));
#50361=CARTESIAN_POINT('Ctrl Pts',(-3.35560332748102,1.14522778786507,-0.393019456018703));
#50362=CARTESIAN_POINT('Ctrl Pts',(-3.27882099545358,1.35034350117479,-0.399978094827215));
#50363=CARTESIAN_POINT('Ctrl Pts',(-3.13698038924816,1.64350653400522,-0.410474690998547));
#50364=CARTESIAN_POINT('Ctrl Pts',(-3.0856854410113,1.73822072635831,-0.413968256504382));
#50365=CARTESIAN_POINT('Ctrl Pts',(-2.94369496598558,1.97346169218265,-0.42315571452732));
#50366=CARTESIAN_POINT('Ctrl Pts',(-2.84709866167595,2.10988559529324,-0.429024287845091));
#50367=CARTESIAN_POINT('Ctrl Pts',(-2.66185301320036,2.3360052457361,-0.439341131585642));
#50368=CARTESIAN_POINT('Ctrl Pts',(-2.57692823718464,2.4290949577846,-0.443787944738417));
#50369=CARTESIAN_POINT('Ctrl Pts',(-2.34801037244829,2.65495355641731,-0.454840078048012));
#50370=CARTESIAN_POINT('Ctrl Pts',(-2.19737874054907,2.78106379178483,-0.461198734534271));
#50371=CARTESIAN_POINT('Ctrl Pts',(-1.92036964617305,2.97668163812499,-0.472153358889957));
#50372=CARTESIAN_POINT('Ctrl Pts',(-1.79827836464648,3.05231368516772,-0.476773484087216));
#50373=CARTESIAN_POINT('Ctrl Pts',(-1.52170858337329,3.20088944047865,-0.487197281551584));
#50374=CARTESIAN_POINT('Ctrl Pts',(-1.36651704388717,3.26994890434684,-0.493106941951451));
#50375=CARTESIAN_POINT('Ctrl Pts',(-1.0882764766723,3.37037022818363,-0.503540441191488));
#50376=CARTESIAN_POINT('Ctrl Pts',(-0.967441676780562,3.4067930852543,-0.507995906633045));
#50377=CARTESIAN_POINT('Ctrl Pts',(-0.626060958562132,3.49033262751781,
-0.520035397606642));
#50378=CARTESIAN_POINT('Ctrl Pts',(-0.401955790064716,3.52324750995501,
-0.527362777079245));
#50379=CARTESIAN_POINT('Ctrl Pts',(0.046994536685491,3.54632696983221,-0.542004409069419));
#50380=CARTESIAN_POINT('Ctrl Pts',(0.272343911910052,3.53676804640221,-0.549351444815277));
#50381=CARTESIAN_POINT('Ctrl Pts',(0.714543154902712,3.47409220313038,-0.564808276006456));
#50382=CARTESIAN_POINT('Ctrl Pts',(0.93070998540505,3.42197040915761,-0.57268477880501));
#50383=CARTESIAN_POINT('Ctrl Pts',(1.35551282987101,3.27687017235962,-0.587857205620805));
#50384=CARTESIAN_POINT('Ctrl Pts',(1.56384301143286,3.18279217961999,-0.595311859425859));
#50385=CARTESIAN_POINT('Ctrl Pts',(1.92537900638715,2.9760312934102,-0.609037087892114));
#50386=CARTESIAN_POINT('Ctrl Pts',(2.08198624499094,2.86916473810887,-0.61529942392855));
#50387=CARTESIAN_POINT('Ctrl Pts',(2.36807079450993,2.63748467631263,-0.627871892321534));
#50388=CARTESIAN_POINT('Ctrl Pts',(2.4980622899226,2.51418367684318,-0.634131858635528));
#50389=CARTESIAN_POINT('Ctrl Pts',(2.91486188186395,2.05465451194467,-0.655285397185308));
#50390=CARTESIAN_POINT('Ctrl Pts',(3.15095910649664,1.67145041150498,-0.669813419630624));
#50391=CARTESIAN_POINT('Ctrl Pts',(3.52463613391811,0.692569723114426,-0.705052234401755));
#50392=CARTESIAN_POINT('Ctrl Pts',(3.54621633695908,0.200862879463424,-0.721539718522704));
#50393=CARTESIAN_POINT('Ctrl Pts',(3.52666383983987,-0.481879494777179,
-0.744564135163527));
#50394=CARTESIAN_POINT('Ctrl Pts',(3.45811077461403,-0.842176755564941,
-0.756420392180674));
#50395=CARTESIAN_POINT('Ctrl Pts',(3.25736628656111,-1.40358634041913,-0.776631454521696));
#50396=CARTESIAN_POINT('Ctrl Pts',(3.15865650858907,-1.61251781614335,-0.784565833919242));
#50397=CARTESIAN_POINT('Ctrl Pts',(2.92821055064976,-1.99952438504932,-0.79997664532621));
#50398=CARTESIAN_POINT('Ctrl Pts',(2.79793621469974,-2.17863074591583,-0.807458959872579));
#50399=CARTESIAN_POINT('Ctrl Pts',(2.51630386371993,-2.49830868772162,-0.821470377673543));
#50400=CARTESIAN_POINT('Ctrl Pts',(2.36755151546159,-2.64000413604234,-0.828064602662562));
#50401=CARTESIAN_POINT('Ctrl Pts',(1.99312519657172,-2.93755773356542,-0.844298502278355));
#50402=CARTESIAN_POINT('Ctrl Pts',(1.76063245456122,-3.08186847586508,-0.853877731932693));
#50403=CARTESIAN_POINT('Ctrl Pts',(1.33245049192624,-3.28478053849265,-0.87012937293106));
#50404=CARTESIAN_POINT('Ctrl Pts',(1.14252574734553,-3.35592075561169,-0.876844985832534));
#50405=CARTESIAN_POINT('Ctrl Pts',(0.835389687708069,-3.44181393966169,
-0.887141175089021));
#50406=CARTESIAN_POINT('Ctrl Pts',(0.721288461272165,-3.46769286696527,
-0.890894806446406));
#50407=CARTESIAN_POINT('Ctrl Pts',(0.387338261788605,-3.52577373228229,
-0.902111489145458));
#50408=CARTESIAN_POINT('Ctrl Pts',(0.165112110420184,-3.54257922935625,
-0.909895716810536));
#50409=CARTESIAN_POINT('Ctrl Pts',(-0.248910843267179,-3.53542029728434,
-0.924394096550147));
#50410=CARTESIAN_POINT('Ctrl Pts',(-0.441035985293887,-3.51655394379901,
-0.931113473593433));
#50411=CARTESIAN_POINT('Ctrl Pts',(-0.740628871199496,-3.46259388153705,
-0.941231187915767));
#50412=CARTESIAN_POINT('Ctrl Pts',(-0.849962403987996,-3.43756499369767,
-0.944845633418973));
#50413=CARTESIAN_POINT('Ctrl Pts',(-1.13273893727573,-3.35856256977466,
-0.954286472322189));
#50414=CARTESIAN_POINT('Ctrl Pts',(-1.30409982554882,-3.29619680482933,
-0.960120117434646));
#50415=CARTESIAN_POINT('Ctrl Pts',(-1.5789481415045,-3.17049461743956,-0.970410037395858));
#50416=CARTESIAN_POINT('Ctrl Pts',(-1.68508967793161,-3.11514817467682,
-0.974596467727152));
#50417=CARTESIAN_POINT('Ctrl Pts',(-1.97738922218214,-2.94340431585692,
-0.986528963749778));
#50418=CARTESIAN_POINT('Ctrl Pts',(-2.1563216082851,-2.81462295238,-0.994303317449499));
#50419=CARTESIAN_POINT('Ctrl Pts',(-2.41987175853691,-2.58567334603244,
-1.00589439518714));
#50420=CARTESIAN_POINT('Ctrl Pts',(-2.51312436759297,-2.49536781564739,
-1.01007085526243));
#50421=CARTESIAN_POINT('Ctrl Pts',(-2.72305745168003,-2.26857122414977,
-1.02002226516135));
#50422=CARTESIAN_POINT('Ctrl Pts',(-2.83508808087039,-2.12753626309955,
-1.02580379523761));
#50423=CARTESIAN_POINT('Ctrl Pts',(-2.99361470261002,-1.89222941309494,
-1.03545767531674));
#50424=CARTESIAN_POINT('Ctrl Pts',(-3.04776462376792,-1.80344547790966,
-1.03909359957781));
#50425=CARTESIAN_POINT('Ctrl Pts',(-3.20701043613858,-1.51431408086861,
-1.05072470901445));
#50426=CARTESIAN_POINT('Ctrl Pts',(-3.29705654279892,-1.30565120601265,
-1.05872996995417));
#50427=CARTESIAN_POINT('Ctrl Pts',(-3.41754289628483,-0.933658716688529,
-1.071713389086));
#50428=CARTESIAN_POINT('Ctrl Pts',(-3.45754212510686,-0.773364951218968,
-1.07702302189057));
#50429=CARTESIAN_POINT('Ctrl Pts',(-3.51751725536643,-0.43432930684903,
-1.08819414784575));
#50430=CARTESIAN_POINT('Ctrl Pts',(-3.5354268517809,-0.2549872896286,-1.094074769187));
#50431=CARTESIAN_POINT('Ctrl Pts',(-3.54172630457513,0.0453303041890943,
-1.10440520742965));
#50432=CARTESIAN_POINT('Ctrl Pts',(-3.53795037963495,0.165791783736955,
-1.10866306074787));
#50433=CARTESIAN_POINT('Ctrl Pts',(-3.5121208012954,0.478496558675268,-1.1197015257511));
#50434=CARTESIAN_POINT('Ctrl Pts',(-3.48036769515908,0.669956557885907,
-1.12632685190405));
#50435=CARTESIAN_POINT('Ctrl Pts',(-3.34339654372091,1.21795369627118,-1.14506294601682));
#50436=CARTESIAN_POINT('Ctrl Pts',(-3.19710898742592,1.56562609795509,-1.15692104335934));
#50437=CARTESIAN_POINT('Ctrl Pts',(-2.9010238832775,2.03669728081193,-1.17620511785791));
#50438=CARTESIAN_POINT('Ctrl Pts',(-2.79175489844723,2.1834392507992,-1.18262151021084));
#50439=CARTESIAN_POINT('Ctrl Pts',(-2.50349542827591,2.51435572427153,-1.19752854069075));
#50440=CARTESIAN_POINT('Ctrl Pts',(-2.31414992392246,2.68963315454088,-1.20598303789464));
#50441=CARTESIAN_POINT('Ctrl Pts',(-1.73142820159205,3.12306231020025,-1.23003668946368));
#50442=CARTESIAN_POINT('Ctrl Pts',(-1.30716002119752,3.32240006877921,-1.24597736898554));
#50443=CARTESIAN_POINT('Ctrl Pts',(-0.47635298230646,3.52788828947166,-1.27486413134219));
#50444=CARTESIAN_POINT('Ctrl Pts',(-0.00281208568693243,3.5803728560144,
-1.2903145799909));
#50445=CARTESIAN_POINT('Ctrl Pts',(0.962642950390408,3.43479177006313,-1.32329300622975));
#50446=CARTESIAN_POINT('Ctrl Pts',(1.38814831774985,3.28503819142457,-1.33859634255934));
#50447=CARTESIAN_POINT('Ctrl Pts',(1.95170676635034,2.96024721458227,-1.36037600144928));
#50448=CARTESIAN_POINT('Ctrl Pts',(2.12275248225467,2.84072814757798,-1.36712528274452));
#50449=CARTESIAN_POINT('Ctrl Pts',(2.43738460292837,2.57508324792456,-1.3808780636241));
#50450=CARTESIAN_POINT('Ctrl Pts',(2.58098915698118,2.43045029872562,-1.38786008447071));
#50451=CARTESIAN_POINT('Ctrl Pts',(2.8586394859375,2.09869429439186,-1.40277376981807));
#50452=CARTESIAN_POINT('Ctrl Pts',(2.98906315475086,1.90841226348734,-1.41070910726487));
#50453=CARTESIAN_POINT('Ctrl Pts',(3.19815239678626,1.5299820023293,-1.42517700597003));
#50454=CARTESIAN_POINT('Ctrl Pts',(3.28109724395731,1.34413783022801,-1.43163438273803));
#50455=CARTESIAN_POINT('Ctrl Pts',(3.39634803821763,1.00968483965148,-1.44327843029447));
#50456=CARTESIAN_POINT('Ctrl Pts',(3.43602173216469,0.864015457437118,-1.44841754354509));
#50457=CARTESIAN_POINT('Ctrl Pts',(3.53497204662554,0.381480622891467,-1.46545574416584));
#50458=CARTESIAN_POINT('Ctrl Pts',(3.55511946807515,0.0361968277201632,
-1.47760960084256));
#50459=CARTESIAN_POINT('Ctrl Pts',(3.51083616031935,-0.485201730785517,
-1.49465759219851));
#50460=CARTESIAN_POINT('Ctrl Pts',(3.48174213458368,-0.664501243521017,
-1.50037677058524));
#50461=CARTESIAN_POINT('Ctrl Pts',(3.41106750725955,-0.953956521790304,
-1.51024647323768));
#50462=CARTESIAN_POINT('Ctrl Pts',(3.37761677741219,-1.065844345292,-1.5142397706781));
#50463=CARTESIAN_POINT('Ctrl Pts',(3.28884372645565,-1.31672952124942,-1.52348839041811));
#50464=CARTESIAN_POINT('Ctrl Pts',(3.2299412503904,-1.45458962814811,-1.52878457157517));
#50465=CARTESIAN_POINT('Ctrl Pts',(3.09404276007104,-1.7245727475059,-1.53934251535052));
#50466=CARTESIAN_POINT('Ctrl Pts',(3.01668666086911,-1.85655784238407,-1.54458881634802));
#50467=CARTESIAN_POINT('Ctrl Pts',(2.85401911859892,-2.09745480011405,-1.55416499746065));
#50468=CARTESIAN_POINT('Ctrl Pts',(2.77017406232646,-2.20737978061453,-1.55857514890632));
#50469=CARTESIAN_POINT('Ctrl Pts',(2.57968153257193,-2.42891544274371,-1.56798252196686));
#50470=CARTESIAN_POINT('Ctrl Pts',(2.47142032382288,-2.53932660034174,-1.57300681173571));
#50471=CARTESIAN_POINT('Ctrl Pts',(2.26674889871784,-2.72156142954571,-1.58237779740596));
#50472=CARTESIAN_POINT('Ctrl Pts',(2.17374705006462,-2.79614947193613,-1.58656527915603));
#50473=CARTESIAN_POINT('Ctrl Pts',(1.91703885326229,-2.981587522261,-1.59773611982311));
#50474=CARTESIAN_POINT('Ctrl Pts',(1.74714305212033,-3.08391680910354,-1.60471445294895));
#50475=CARTESIAN_POINT('Ctrl Pts',(1.45057804879874,-3.23076970868732,-1.61574175119124));
#50476=CARTESIAN_POINT('Ctrl Pts',(1.32782272610411,-3.28327703514645,-1.62005309437341));
#50477=CARTESIAN_POINT('Ctrl Pts',(1.01941548265538,-3.39520141140918,-1.6306426349041));
#50478=CARTESIAN_POINT('Ctrl Pts',(0.830807073977391,-3.44665349448751,
-1.63691624518133));
#50479=CARTESIAN_POINT('Ctrl Pts',(0.537265653796465,-3.50051786116815,
-1.64709107891152));
#50480=CARTESIAN_POINT('Ctrl Pts',(0.434611008595293,-3.51460779609371,
-1.65072101263908));
#50481=CARTESIAN_POINT('Ctrl Pts',(0.225619775887951,-3.5339495654796,-1.65811986209128));
#50482=CARTESIAN_POINT('Ctrl Pts',(0.119263996534475,-3.53894775575562,
-1.66188927246119));
#50483=CARTESIAN_POINT('Ctrl Pts',(-0.162387922266383,-3.53959510891038,
-1.67168223495486));
#50484=CARTESIAN_POINT('Ctrl Pts',(-0.337739076371664,-3.52708781787918,
-1.67751988457496));
#50485=CARTESIAN_POINT('Ctrl Pts',(-0.823259525169688,-3.45652111654826,
-1.69357469929039));
#50486=CARTESIAN_POINT('Ctrl Pts',(-1.13038309976021,-3.36988303997754,
-1.70368211808393));
#50487=CARTESIAN_POINT('Ctrl Pts',(-1.57217878647256,-3.17584433311836,
-1.72045025447723));
#50488=CARTESIAN_POINT('Ctrl Pts',(-1.71819803180833,-3.09889906111367,
-1.72631027718014));
#50489=CARTESIAN_POINT('Ctrl Pts',(-2.00528096082112,-2.92123243107852,
-1.73788904679044));
#50490=CARTESIAN_POINT('Ctrl Pts',(-2.1457412982902,-2.81950204643683,-1.74364609212141));
#50491=CARTESIAN_POINT('Ctrl Pts',(-2.45175935497528,-2.56229840409746,
-1.75683120431308));
#50492=CARTESIAN_POINT('Ctrl Pts',(-2.61159360171125,-2.39988572783075,
-1.76422818059013));
#50493=CARTESIAN_POINT('Ctrl Pts',(-2.90047120263545,-2.04298664406632,
-1.77964685741253));
#50494=CARTESIAN_POINT('Ctrl Pts',(-3.02708811987471,-1.8494542979142,-1.78776396049441));
#50495=CARTESIAN_POINT('Ctrl Pts',(-3.2785531111803,-1.36838472126582,-1.80632724926333));
#50496=CARTESIAN_POINT('Ctrl Pts',(-3.38664983884328,-1.07273690227071,
-1.81667718039125));
#50497=CARTESIAN_POINT('Ctrl Pts',(-3.55709012362553,-0.311449824495371,
-1.84263604131696));
#50498=CARTESIAN_POINT('Ctrl Pts',(-3.56668710098688,0.155659841452416,
-1.85831670276059));
#50499=CARTESIAN_POINT('Ctrl Pts',(-3.48534662539474,0.614552563975331,
-1.87410368362543));
#50500=CARTESIAN_POINT('Ctrl Pts',(-1.474278984797,3.218400452862,0.2851535733017));
#50501=CARTESIAN_POINT('Ctrl Pts',(-0.8630012166369,3.498413453318,0.2624820910321));
#50502=CARTESIAN_POINT('Ctrl Pts',(0.5221776990155,3.700023104325,0.2171391264928));
#50503=CARTESIAN_POINT('Ctrl Pts',(2.435930668196,2.833759612852,0.1491246796839));
#50504=CARTESIAN_POINT('Ctrl Pts',(3.579719046399,1.071968677256,0.0811102328749));
#50505=CARTESIAN_POINT('Ctrl Pts',(3.592463812753,-1.028508980771,0.01309578606595));
#50506=CARTESIAN_POINT('Ctrl Pts',(2.470048545545,-2.804008613372,-0.05491866074299));
#50507=CARTESIAN_POINT('Ctrl Pts',(0.5671562238518,-3.693499629492,-0.1229331075519));
#50508=CARTESIAN_POINT('Ctrl Pts',(-1.514946598719,-3.415924974072,-0.1909475543609));
#50509=CARTESIAN_POINT('Ctrl Pts',(-3.118358578085,-2.058991469437,-0.2589620011698));
#50510=CARTESIAN_POINT('Ctrl Pts',(-3.736436540906,-0.05146107378251,-0.3269764479788));
#50511=CARTESIAN_POINT('Ctrl Pts',(-3.173881046339,1.972329924211,-0.3949908947877));
#50512=CARTESIAN_POINT('Ctrl Pts',(-1.608447541355,3.37290716424,-0.4630053415967));
#50513=CARTESIAN_POINT('Ctrl Pts',(0.4652207285,3.707718423233,-0.5310197884056));
#50514=CARTESIAN_POINT('Ctrl Pts',(2.391889272583,2.870970557034,-0.5990342352146));
#50515=CARTESIAN_POINT('Ctrl Pts',(3.56277234894,1.127057860763,-0.6670486820235));
#50516=CARTESIAN_POINT('Ctrl Pts',(3.607896136365,-0.972980832813,-0.7350631288325));
#50517=CARTESIAN_POINT('Ctrl Pts',(2.513002490438,-2.765578549758,-0.8030775756414));
#50518=CARTESIAN_POINT('Ctrl Pts',(0.6240542096492,-3.6843130398,-0.8710920224504));
#50519=CARTESIAN_POINT('Ctrl Pts',(-1.462081753792,-3.438884001694,-0.9391064692593));
#50520=CARTESIAN_POINT('Ctrl Pts',(-3.086231389081,-2.106841722746,-1.007120916068));
#50521=CARTESIAN_POINT('Ctrl Pts',(-3.735198409991,-0.1090828593897,-1.075135362877));
#50522=CARTESIAN_POINT('Ctrl Pts',(-3.203923222005,1.92314383741,-1.143149809686));
#50523=CARTESIAN_POINT('Ctrl Pts',(-1.660277337509,3.347698521193,-1.211164256495));
#50524=CARTESIAN_POINT('Ctrl Pts',(0.4079804125565,3.714452617722,-1.279178703304));
#50525=CARTESIAN_POINT('Ctrl Pts',(2.347325129349,2.907519704122,-1.347193150113));
#50526=CARTESIAN_POINT('Ctrl Pts',(3.544965740915,1.181873310129,-1.415207596922));
#50527=CARTESIAN_POINT('Ctrl Pts',(3.622473367692,-0.917219927648,-1.483222043731));
#50528=CARTESIAN_POINT('Ctrl Pts',(2.55535821773,-2.726490143077,-1.55123649054));
#50529=CARTESIAN_POINT('Ctrl Pts',(0.6808021457163,-3.674253040803,-1.619250937349));
#50530=CARTESIAN_POINT('Ctrl Pts',(-1.408862321174,-3.461013183469,-1.687265384158));
#50531=CARTESIAN_POINT('Ctrl Pts',(-3.053395514624,-2.154234804974,-1.755279830967));
#50532=CARTESIAN_POINT('Ctrl Pts',(-3.732976491904,-0.1665143620988,-1.823294277776));
#50533=CARTESIAN_POINT('Ctrl Pts',(-3.400031230562,1.193086510473,-1.868637242315));
#50534=CARTESIAN_POINT('Ctrl Pts',(-3.062932791185,1.774835968952,-1.891308724585));
#50535=CARTESIAN_POINT('Ctrl Pts',(-1.474278984797,3.218400452862,0.1959004713425));
#50536=CARTESIAN_POINT('Ctrl Pts',(-0.8630012166369,3.498413453318,0.1732289890729));
#50537=CARTESIAN_POINT('Ctrl Pts',(0.5221776990155,3.700023104325,0.1278860245336));
#50538=CARTESIAN_POINT('Ctrl Pts',(2.435930668196,2.833759612852,0.05987157772462));
#50539=CARTESIAN_POINT('Ctrl Pts',(3.579719046399,1.071968677256,-0.008142869084334));
#50540=CARTESIAN_POINT('Ctrl Pts',(3.592463812753,-1.028508980771,-0.07615731589328));
#50541=CARTESIAN_POINT('Ctrl Pts',(2.470048545545,-2.804008613372,-0.1441717627022));
#50542=CARTESIAN_POINT('Ctrl Pts',(0.5671562238518,-3.693499629492,-0.2121862095112));
#50543=CARTESIAN_POINT('Ctrl Pts',(-1.514946598719,-3.415924974072,-0.2802006563201));
#50544=CARTESIAN_POINT('Ctrl Pts',(-3.118358578085,-2.058991469437,-0.3482151031291));
#50545=CARTESIAN_POINT('Ctrl Pts',(-3.736436540906,-0.05146107378251,-0.416229549938));
#50546=CARTESIAN_POINT('Ctrl Pts',(-3.173881046339,1.972329924211,-0.484243996747));
#50547=CARTESIAN_POINT('Ctrl Pts',(-1.608447541355,3.37290716424,-0.5522584435559));
#50548=CARTESIAN_POINT('Ctrl Pts',(0.4652207285,3.707718423233,-0.6202728903649));
#50549=CARTESIAN_POINT('Ctrl Pts',(2.391889272583,2.870970557034,-0.6882873371738));
#50550=CARTESIAN_POINT('Ctrl Pts',(3.56277234894,1.127057860763,-0.7563017839828));
#50551=CARTESIAN_POINT('Ctrl Pts',(3.607896136365,-0.972980832813,-0.8243162307917));
#50552=CARTESIAN_POINT('Ctrl Pts',(2.513002490438,-2.765578549758,-0.8923306776007));
#50553=CARTESIAN_POINT('Ctrl Pts',(0.6240542096492,-3.6843130398,-0.9603451244096));
#50554=CARTESIAN_POINT('Ctrl Pts',(-1.462081753792,-3.438884001694,-1.028359571219));
#50555=CARTESIAN_POINT('Ctrl Pts',(-3.086231389081,-2.106841722746,-1.096374018028));
#50556=CARTESIAN_POINT('Ctrl Pts',(-3.735198409991,-0.1090828593897,-1.164388464836));
#50557=CARTESIAN_POINT('Ctrl Pts',(-3.203923222005,1.92314383741,-1.232402911645));
#50558=CARTESIAN_POINT('Ctrl Pts',(-1.660277337509,3.347698521193,-1.300417358454));
#50559=CARTESIAN_POINT('Ctrl Pts',(0.4079804125565,3.714452617722,-1.368431805263));
#50560=CARTESIAN_POINT('Ctrl Pts',(2.347325129349,2.907519704122,-1.436446252072));
#50561=CARTESIAN_POINT('Ctrl Pts',(3.544965740915,1.181873310129,-1.504460698881));
#50562=CARTESIAN_POINT('Ctrl Pts',(3.622473367692,-0.917219927648,-1.57247514569));
#50563=CARTESIAN_POINT('Ctrl Pts',(2.55535821773,-2.726490143077,-1.640489592499));
#50564=CARTESIAN_POINT('Ctrl Pts',(0.6808021457163,-3.674253040803,-1.708504039308));
#50565=CARTESIAN_POINT('Ctrl Pts',(-1.408862321174,-3.461013183469,-1.776518486117));
#50566=CARTESIAN_POINT('Ctrl Pts',(-3.053395514624,-2.154234804974,-1.844532932926));
#50567=CARTESIAN_POINT('Ctrl Pts',(-3.732976491904,-0.1665143620988,-1.912547379735));
#50568=CARTESIAN_POINT('Ctrl Pts',(-3.400031230562,1.193086510473,-1.957890344274));
#50569=CARTESIAN_POINT('Ctrl Pts',(-3.062932791185,1.774835968952,-1.980561826544));
#50570=CARTESIAN_POINT('Ctrl Pts',(-1.474278984797,3.218400452862,0.1066473693833));
#50571=CARTESIAN_POINT('Ctrl Pts',(-0.8630012166369,3.498413453318,0.08397588711363));
#50572=CARTESIAN_POINT('Ctrl Pts',(0.5221776990155,3.700023104325,0.03863292257433));
#50573=CARTESIAN_POINT('Ctrl Pts',(2.435930668196,2.833759612852,-0.02938152423462));
#50574=CARTESIAN_POINT('Ctrl Pts',(3.579719046399,1.071968677256,-0.09739597104357));
#50575=CARTESIAN_POINT('Ctrl Pts',(3.592463812753,-1.028508980771,-0.1654104178525));
#50576=CARTESIAN_POINT('Ctrl Pts',(2.470048545545,-2.804008613372,-0.2334248646615));
#50577=CARTESIAN_POINT('Ctrl Pts',(0.5671562238518,-3.693499629492,-0.3014393114704));
#50578=CARTESIAN_POINT('Ctrl Pts',(-1.514946598719,-3.415924974072,-0.3694537582794));
#50579=CARTESIAN_POINT('Ctrl Pts',(-3.118358578085,-2.058991469437,-0.4374682050883));
#50580=CARTESIAN_POINT('Ctrl Pts',(-3.736436540906,-0.05146107378252,-0.5054826518973));
#50581=CARTESIAN_POINT('Ctrl Pts',(-3.173881046339,1.972329924211,-0.5734970987062));
#50582=CARTESIAN_POINT('Ctrl Pts',(-1.608447541355,3.37290716424,-0.6415115455152));
#50583=CARTESIAN_POINT('Ctrl Pts',(0.4652207285,3.707718423233,-0.7095259923241));
#50584=CARTESIAN_POINT('Ctrl Pts',(2.391889272583,2.870970557034,-0.7775404391331));
#50585=CARTESIAN_POINT('Ctrl Pts',(3.56277234894,1.127057860763,-0.845554885942));
#50586=CARTESIAN_POINT('Ctrl Pts',(3.607896136365,-0.972980832813,-0.9135693327509));
#50587=CARTESIAN_POINT('Ctrl Pts',(2.513002490438,-2.765578549758,-0.9815837795599));
#50588=CARTESIAN_POINT('Ctrl Pts',(0.6240542096492,-3.6843130398,-1.049598226369));
#50589=CARTESIAN_POINT('Ctrl Pts',(-1.462081753792,-3.438884001694,-1.117612673178));
#50590=CARTESIAN_POINT('Ctrl Pts',(-3.086231389081,-2.106841722746,-1.185627119987));
#50591=CARTESIAN_POINT('Ctrl Pts',(-3.735198409991,-0.1090828593897,-1.253641566796));
#50592=CARTESIAN_POINT('Ctrl Pts',(-3.203923222005,1.92314383741,-1.321656013605));
#50593=CARTESIAN_POINT('Ctrl Pts',(-1.660277337509,3.347698521193,-1.389670460414));
#50594=CARTESIAN_POINT('Ctrl Pts',(0.4079804125565,3.714452617722,-1.457684907223));
#50595=CARTESIAN_POINT('Ctrl Pts',(2.347325129348,2.907519704122,-1.525699354031));
#50596=CARTESIAN_POINT('Ctrl Pts',(3.544965740915,1.181873310129,-1.59371380084));
#50597=CARTESIAN_POINT('Ctrl Pts',(3.622473367692,-0.917219927648,-1.661728247649));
#50598=CARTESIAN_POINT('Ctrl Pts',(2.55535821773,-2.726490143077,-1.729742694458));
#50599=CARTESIAN_POINT('Ctrl Pts',(0.6808021457163,-3.674253040803,-1.797757141267));
#50600=CARTESIAN_POINT('Ctrl Pts',(-1.408862321174,-3.461013183469,-1.865771588076));
#50601=CARTESIAN_POINT('Ctrl Pts',(-3.053395514624,-2.154234804974,-1.933786034885));
#50602=CARTESIAN_POINT('Ctrl Pts',(-3.732976491904,-0.1665143620988,-2.001800481694));
#50603=CARTESIAN_POINT('Ctrl Pts',(-3.400031230562,1.193086510473,-2.047143446233));
#50604=CARTESIAN_POINT('Ctrl Pts',(-3.062932791185,1.774835968952,-2.069814928503));
#50605=CARTESIAN_POINT('Ctrl Pts',(-1.474278984797,3.218400452862,0.01739426742404));
#50606=CARTESIAN_POINT('Ctrl Pts',(-0.8630012166369,3.498413453318,-0.005277214845608));
#50607=CARTESIAN_POINT('Ctrl Pts',(0.5221776990155,3.700023104325,-0.05062017938491));
#50608=CARTESIAN_POINT('Ctrl Pts',(2.435930668196,2.833759612852,-0.1186346261939));
#50609=CARTESIAN_POINT('Ctrl Pts',(3.579719046399,1.071968677256,-0.1866490730028));
#50610=CARTESIAN_POINT('Ctrl Pts',(3.592463812753,-1.028508980771,-0.2546635198118));
#50611=CARTESIAN_POINT('Ctrl Pts',(2.470048545545,-2.804008613372,-0.3226779666207));
#50612=CARTESIAN_POINT('Ctrl Pts',(0.5671562238518,-3.693499629492,-0.3906924134296));
#50613=CARTESIAN_POINT('Ctrl Pts',(-1.514946598719,-3.415924974072,-0.4587068602386));
#50614=CARTESIAN_POINT('Ctrl Pts',(-3.118358578085,-2.058991469437,-0.5267213070475));
#50615=CARTESIAN_POINT('Ctrl Pts',(-3.736436540906,-0.05146107378252,-0.5947357538565));
#50616=CARTESIAN_POINT('Ctrl Pts',(-3.173881046339,1.972329924211,-0.6627502006654));
#50617=CARTESIAN_POINT('Ctrl Pts',(-1.608447541355,3.37290716424,-0.7307646474744));
#50618=CARTESIAN_POINT('Ctrl Pts',(0.4652207285,3.707718423233,-0.7987790942833));
#50619=CARTESIAN_POINT('Ctrl Pts',(2.391889272583,2.870970557034,-0.8667935410923));
#50620=CARTESIAN_POINT('Ctrl Pts',(3.56277234894,1.127057860763,-0.9348079879012));
#50621=CARTESIAN_POINT('Ctrl Pts',(3.607896136365,-0.972980832813,-1.00282243471));
#50622=CARTESIAN_POINT('Ctrl Pts',(2.513002490438,-2.765578549758,-1.070836881519));
#50623=CARTESIAN_POINT('Ctrl Pts',(0.6240542096492,-3.6843130398,-1.138851328328));
#50624=CARTESIAN_POINT('Ctrl Pts',(-1.462081753792,-3.438884001694,-1.206865775137));
#50625=CARTESIAN_POINT('Ctrl Pts',(-3.086231389081,-2.106841722746,-1.274880221946));
#50626=CARTESIAN_POINT('Ctrl Pts',(-3.735198409991,-0.1090828593897,-1.342894668755));
#50627=CARTESIAN_POINT('Ctrl Pts',(-3.203923222005,1.92314383741,-1.410909115564));
#50628=CARTESIAN_POINT('Ctrl Pts',(-1.660277337509,3.347698521193,-1.478923562373));
#50629=CARTESIAN_POINT('Ctrl Pts',(0.4079804125565,3.714452617722,-1.546938009182));
#50630=CARTESIAN_POINT('Ctrl Pts',(2.347325129348,2.907519704122,-1.614952455991));
#50631=CARTESIAN_POINT('Ctrl Pts',(3.544965740915,1.181873310129,-1.6829669028));
#50632=CARTESIAN_POINT('Ctrl Pts',(3.622473367692,-0.917219927648,-1.750981349609));
#50633=CARTESIAN_POINT('Ctrl Pts',(2.55535821773,-2.726490143077,-1.818995796418));
#50634=CARTESIAN_POINT('Ctrl Pts',(0.6808021457163,-3.674253040803,-1.887010243227));
#50635=CARTESIAN_POINT('Ctrl Pts',(-1.408862321174,-3.461013183469,-1.955024690035));
#50636=CARTESIAN_POINT('Ctrl Pts',(-3.053395514624,-2.154234804974,-2.023039136844));
#50637=CARTESIAN_POINT('Ctrl Pts',(-3.732976491904,-0.1665143620988,-2.091053583653));
#50638=CARTESIAN_POINT('Ctrl Pts',(-3.400031230562,1.193086510473,-2.136396548193));
#50639=CARTESIAN_POINT('Ctrl Pts',(-3.062932791185,1.774835968952,-2.159068030462));
#50640=CARTESIAN_POINT('',(-3.486219445663,0.6147145489409,-1.873914457161));
#50641=CARTESIAN_POINT('Ctrl Pts',(-3.381685401913,-1.046806497156,-1.792787013728));
#50642=CARTESIAN_POINT('Ctrl Pts',(-3.516276022629,-0.6120144524515,-1.80813423595));
#50643=CARTESIAN_POINT('Ctrl Pts',(-3.615602476197,0.3099418872051,-1.838828680394));
#50644=CARTESIAN_POINT('Ctrl Pts',(-3.233351390461,1.647480520897,-1.884870347061));
#50645=CARTESIAN_POINT('Ctrl Pts',(-2.375970535719,2.742894243674,-1.930912013728));
#50646=CARTESIAN_POINT('Ctrl Pts',(-1.16946135002,3.435270189528,-1.976953680394));
#50647=CARTESIAN_POINT('Ctrl Pts',(0.2088925691034,3.622855283072,-2.022995347061));
#50648=CARTESIAN_POINT('Ctrl Pts',(1.556551006228,3.278088863066,-2.069037013728));
#50649=CARTESIAN_POINT('Ctrl Pts',(2.675485639469,2.451630885082,-2.115078680394));
#50650=CARTESIAN_POINT('Ctrl Pts',(3.401277069744,1.264923606363,-2.161120347061));
#50651=CARTESIAN_POINT('Ctrl Pts',(3.627275538361,-0.1076550254197,-2.207162013728));
#50652=CARTESIAN_POINT('Ctrl Pts',(3.320272205746,-1.464414529052,-2.253203680394));
#50653=CARTESIAN_POINT('Ctrl Pts',(2.525378983787,-2.605988952896,-2.299245347061));
#50654=CARTESIAN_POINT('Ctrl Pts',(1.359399658728,-3.364632223854,-2.345287013728));
#50655=CARTESIAN_POINT('Ctrl Pts',(-0.006333574545319,-3.628867222688,-2.391328680394));
#50656=CARTESIAN_POINT('Ctrl Pts',(-1.371136135038,-3.359866535032,-2.437370347061));
#50657=CARTESIAN_POINT('Ctrl Pts',(-2.534460197325,-2.597157858548,-2.483412013728));
#50658=CARTESIAN_POINT('Ctrl Pts',(-3.325363738216,-1.452815694643,-2.529453680394));
#50659=CARTESIAN_POINT('Ctrl Pts',(-3.627629225714,-0.09499281438667,-2.575495347061));
#50660=CARTESIAN_POINT('Ctrl Pts',(-3.396840941408,1.276788570131,-2.621537013728));
#50661=CARTESIAN_POINT('Ctrl Pts',(-2.66691154775,2.460955145979,-2.667578680394));
#50662=CARTESIAN_POINT('Ctrl Pts',(-1.545098868578,3.283502233951,-2.713620347061));
#50663=CARTESIAN_POINT('Ctrl Pts',(-0.1962451307805,3.623562512595,-2.759662013728));
#50664=CARTESIAN_POINT('Ctrl Pts',(1.181445403903,3.431166593396,-2.805703680394));
#50665=CARTESIAN_POINT('Ctrl Pts',(2.385531115837,2.73458565955,-2.851745347061));
#50666=CARTESIAN_POINT('Ctrl Pts',(3.239080353414,1.636177220892,-2.897787013728));
#50667=CARTESIAN_POINT('Ctrl Pts',(3.616670254429,0.2973444211245,-2.943828680394));
#50668=CARTESIAN_POINT('Ctrl Pts',(3.462816724887,-1.085180982088,-2.989870347061));
#50669=CARTESIAN_POINT('Ctrl Pts',(2.80012742371,-2.30824692029,-3.035912013728));
#50670=CARTESIAN_POINT('Ctrl Pts',(1.725979731427,-3.192132735452,-3.081953680394));
#50671=CARTESIAN_POINT('Ctrl Pts',(0.3982118512334,-3.606957825589,-3.127995347061));
#50672=CARTESIAN_POINT('Ctrl Pts',(-0.9880703687869,-3.491766656059,-3.174037013728));
#50673=CARTESIAN_POINT('Ctrl Pts',(-2.229162823228,-2.863485732736,-3.220078680394));
#50674=CARTESIAN_POINT('Ctrl Pts',(-3.142695988404,-1.814436374886,-3.266120347061));
#50675=CARTESIAN_POINT('Ctrl Pts',(-3.594432799537,-0.4987687677191,-3.312162013728));
#50676=CARTESIAN_POINT('Ctrl Pts',(-3.517993812628,0.8901892879335,-3.358203680394));
#50677=CARTESIAN_POINT('Ctrl Pts',(-2.924611181723,2.148340492051,-3.404245347061));
#50678=CARTESIAN_POINT('Ctrl Pts',(-1.90147817544,3.090808661559,-3.450287013728));
#50679=CARTESIAN_POINT('Ctrl Pts',(-0.598936759323,3.579104942911,-3.496328680394));
#50680=CARTESIAN_POINT('Ctrl Pts',(0.791614064251,3.541477743446,-3.542370347061));
#50681=CARTESIAN_POINT('Ctrl Pts',(2.065842949582,2.983456106884,-3.588412013728));
#50682=CARTESIAN_POINT('Ctrl Pts',(3.036511215093,1.98703726051,-3.634453680394));
#50683=CARTESIAN_POINT('Ctrl Pts',(3.560986207913,0.6986377180585,-3.680495347061));
#50684=CARTESIAN_POINT('Ctrl Pts',(3.562200136449,-0.6924215637334,-3.726537013728));
#50685=CARTESIAN_POINT('Ctrl Pts',(3.039974622718,-1.981734524923,-3.772578680394));
#50686=CARTESIAN_POINT('Ctrl Pts',(2.071046913695,-2.979845988523,-3.818620347061));
#50687=CARTESIAN_POINT('Ctrl Pts',(0.7977939001169,-3.540090722987,-3.864662013728));
#50688=CARTESIAN_POINT('Ctrl Pts',(-0.592689133709,-3.58014483294,-3.910703680394));
#50689=CARTESIAN_POINT('Ctrl Pts',(-1.896080803293,-3.094122657786,-3.956745347061));
#50690=CARTESIAN_POINT('Ctrl Pts',(-2.920857167686,-2.153441626797,-4.002787013728));
#50691=CARTESIAN_POINT('Ctrl Pts',(-3.516434781803,-0.8963279864901,-4.048828680394));
#50692=CARTESIAN_POINT('Ctrl Pts',(-3.595297840182,0.4924945425259,-4.094870347061));
#50693=CARTESIAN_POINT('Ctrl Pts',(-3.145857989081,1.808948574891,-4.140912013728));
#50694=CARTESIAN_POINT('Ctrl Pts',(-2.234157150885,2.859590750281,-4.186953680394));
#50695=CARTESIAN_POINT('Ctrl Pts',(-0.9941631432962,3.490036830591,-4.232995347061));
#50696=CARTESIAN_POINT('Ctrl Pts',(0.3919159190425,3.607647342181,-4.279037013728));
#50697=CARTESIAN_POINT('Ctrl Pts',(1.720405782322,3.195140275457,-4.325078680394));
#50698=CARTESIAN_POINT('Ctrl Pts',(2.796094511829,2.313130544526,-4.371120347061));
#50699=CARTESIAN_POINT('Ctrl Pts',(3.460917446918,1.091223088699,-4.417162013728));
#50700=CARTESIAN_POINT('Ctrl Pts',(3.617183734391,-0.2910317178534,-4.463203680394));
#50701=CARTESIAN_POINT('Ctrl Pts',(3.241930993927,-1.630521370031,-4.509245347061));
#50702=CARTESIAN_POINT('Ctrl Pts',(2.390300577984,-2.730418332625,-4.555287013728));
#50703=CARTESIAN_POINT('Ctrl Pts',(1.187430827056,-3.429097964413,-4.601328680394));
#50704=CARTESIAN_POINT('Ctrl Pts',(-0.1899157118936,-3.62390470395,-4.647370347061));
#50705=CARTESIAN_POINT('Ctrl Pts',(-1.539383690082,-3.286174537975,-4.693412013728));
#50706=CARTESIAN_POINT('Ctrl Pts',(-2.288158074621,-2.739177136089,-4.724106458172));
#50707=CARTESIAN_POINT('Ctrl Pts',(-2.59740372034,-2.405222217086,-4.739453680394));
#50708=CARTESIAN_POINT('Ctrl Pts',(-3.381685401913,-1.046806497156,-1.882040115687));
#50709=CARTESIAN_POINT('Ctrl Pts',(-3.516276022629,-0.6120144524515,-1.897387337909));
#50710=CARTESIAN_POINT('Ctrl Pts',(-3.615602476197,0.3099418872051,-1.928081782354));
#50711=CARTESIAN_POINT('Ctrl Pts',(-3.233351390461,1.647480520897,-1.97412344902));
#50712=CARTESIAN_POINT('Ctrl Pts',(-2.375970535719,2.742894243674,-2.020165115687));
#50713=CARTESIAN_POINT('Ctrl Pts',(-1.16946135002,3.435270189528,-2.066206782354));
#50714=CARTESIAN_POINT('Ctrl Pts',(0.2088925691034,3.622855283072,-2.11224844902));
#50715=CARTESIAN_POINT('Ctrl Pts',(1.556551006228,3.278088863066,-2.158290115687));
#50716=CARTESIAN_POINT('Ctrl Pts',(2.675485639469,2.451630885082,-2.204331782354));
#50717=CARTESIAN_POINT('Ctrl Pts',(3.401277069744,1.264923606363,-2.25037344902));
#50718=CARTESIAN_POINT('Ctrl Pts',(3.627275538361,-0.1076550254197,-2.296415115687));
#50719=CARTESIAN_POINT('Ctrl Pts',(3.320272205746,-1.464414529052,-2.342456782354));
#50720=CARTESIAN_POINT('Ctrl Pts',(2.525378983787,-2.605988952896,-2.38849844902));
#50721=CARTESIAN_POINT('Ctrl Pts',(1.359399658728,-3.364632223854,-2.434540115687));
#50722=CARTESIAN_POINT('Ctrl Pts',(-0.006333574545319,-3.628867222688,-2.480581782354));
#50723=CARTESIAN_POINT('Ctrl Pts',(-1.371136135038,-3.359866535032,-2.52662344902));
#50724=CARTESIAN_POINT('Ctrl Pts',(-2.534460197325,-2.597157858548,-2.572665115687));
#50725=CARTESIAN_POINT('Ctrl Pts',(-3.325363738216,-1.452815694643,-2.618706782354));
#50726=CARTESIAN_POINT('Ctrl Pts',(-3.627629225714,-0.09499281438667,-2.66474844902));
#50727=CARTESIAN_POINT('Ctrl Pts',(-3.396840941408,1.276788570131,-2.710790115687));
#50728=CARTESIAN_POINT('Ctrl Pts',(-2.66691154775,2.460955145979,-2.756831782354));
#50729=CARTESIAN_POINT('Ctrl Pts',(-1.545098868578,3.283502233951,-2.80287344902));
#50730=CARTESIAN_POINT('Ctrl Pts',(-0.1962451307805,3.623562512595,-2.848915115687));
#50731=CARTESIAN_POINT('Ctrl Pts',(1.181445403903,3.431166593396,-2.894956782354));
#50732=CARTESIAN_POINT('Ctrl Pts',(2.385531115837,2.73458565955,-2.94099844902));
#50733=CARTESIAN_POINT('Ctrl Pts',(3.239080353414,1.636177220892,-2.987040115687));
#50734=CARTESIAN_POINT('Ctrl Pts',(3.616670254429,0.2973444211245,-3.033081782354));
#50735=CARTESIAN_POINT('Ctrl Pts',(3.462816724887,-1.085180982088,-3.07912344902));
#50736=CARTESIAN_POINT('Ctrl Pts',(2.80012742371,-2.30824692029,-3.125165115687));
#50737=CARTESIAN_POINT('Ctrl Pts',(1.725979731427,-3.192132735452,-3.171206782354));
#50738=CARTESIAN_POINT('Ctrl Pts',(0.3982118512334,-3.606957825589,-3.21724844902));
#50739=CARTESIAN_POINT('Ctrl Pts',(-0.9880703687869,-3.491766656059,-3.263290115687));
#50740=CARTESIAN_POINT('Ctrl Pts',(-2.229162823228,-2.863485732736,-3.309331782354));
#50741=CARTESIAN_POINT('Ctrl Pts',(-3.142695988404,-1.814436374886,-3.35537344902));
#50742=CARTESIAN_POINT('Ctrl Pts',(-3.594432799537,-0.4987687677191,-3.401415115687));
#50743=CARTESIAN_POINT('Ctrl Pts',(-3.517993812628,0.8901892879335,-3.447456782354));
#50744=CARTESIAN_POINT('Ctrl Pts',(-2.924611181723,2.148340492051,-3.49349844902));
#50745=CARTESIAN_POINT('Ctrl Pts',(-1.90147817544,3.090808661559,-3.539540115687));
#50746=CARTESIAN_POINT('Ctrl Pts',(-0.598936759323,3.579104942911,-3.585581782354));
#50747=CARTESIAN_POINT('Ctrl Pts',(0.791614064251,3.541477743446,-3.63162344902));
#50748=CARTESIAN_POINT('Ctrl Pts',(2.065842949582,2.983456106884,-3.677665115687));
#50749=CARTESIAN_POINT('Ctrl Pts',(3.036511215093,1.98703726051,-3.723706782354));
#50750=CARTESIAN_POINT('Ctrl Pts',(3.560986207913,0.6986377180585,-3.76974844902));
#50751=CARTESIAN_POINT('Ctrl Pts',(3.562200136449,-0.6924215637334,-3.815790115687));
#50752=CARTESIAN_POINT('Ctrl Pts',(3.039974622718,-1.981734524923,-3.861831782354));
#50753=CARTESIAN_POINT('Ctrl Pts',(2.071046913695,-2.979845988523,-3.90787344902));
#50754=CARTESIAN_POINT('Ctrl Pts',(0.7977939001169,-3.540090722987,-3.953915115687));
#50755=CARTESIAN_POINT('Ctrl Pts',(-0.592689133709,-3.58014483294,-3.999956782354));
#50756=CARTESIAN_POINT('Ctrl Pts',(-1.896080803293,-3.094122657786,-4.04599844902));
#50757=CARTESIAN_POINT('Ctrl Pts',(-2.920857167686,-2.153441626797,-4.092040115687));
#50758=CARTESIAN_POINT('Ctrl Pts',(-3.516434781803,-0.8963279864901,-4.138081782354));
#50759=CARTESIAN_POINT('Ctrl Pts',(-3.595297840182,0.4924945425259,-4.18412344902));
#50760=CARTESIAN_POINT('Ctrl Pts',(-3.145857989081,1.808948574891,-4.230165115687));
#50761=CARTESIAN_POINT('Ctrl Pts',(-2.234157150885,2.859590750281,-4.276206782354));
#50762=CARTESIAN_POINT('Ctrl Pts',(-0.9941631432962,3.490036830591,-4.32224844902));
#50763=CARTESIAN_POINT('Ctrl Pts',(0.3919159190425,3.607647342181,-4.368290115687));
#50764=CARTESIAN_POINT('Ctrl Pts',(1.720405782322,3.195140275457,-4.414331782354));
#50765=CARTESIAN_POINT('Ctrl Pts',(2.796094511829,2.313130544526,-4.46037344902));
#50766=CARTESIAN_POINT('Ctrl Pts',(3.460917446918,1.091223088699,-4.506415115687));
#50767=CARTESIAN_POINT('Ctrl Pts',(3.617183734391,-0.2910317178534,-4.552456782354));
#50768=CARTESIAN_POINT('Ctrl Pts',(3.241930993927,-1.630521370031,-4.59849844902));
#50769=CARTESIAN_POINT('Ctrl Pts',(2.390300577984,-2.730418332625,-4.644540115687));
#50770=CARTESIAN_POINT('Ctrl Pts',(1.187430827056,-3.429097964413,-4.690581782354));
#50771=CARTESIAN_POINT('Ctrl Pts',(-0.1899157118936,-3.62390470395,-4.73662344902));
#50772=CARTESIAN_POINT('Ctrl Pts',(-1.539383690082,-3.286174537975,-4.782665115687));
#50773=CARTESIAN_POINT('Ctrl Pts',(-2.288158074621,-2.739177136089,-4.813359560131));
#50774=CARTESIAN_POINT('Ctrl Pts',(-2.59740372034,-2.405222217086,-4.828706782354));
#50775=CARTESIAN_POINT('Ctrl Pts',(-3.381685401913,-1.046806497156,-1.971293217646));
#50776=CARTESIAN_POINT('Ctrl Pts',(-3.516276022629,-0.6120144524515,-1.986640439869));
#50777=CARTESIAN_POINT('Ctrl Pts',(-3.615602476197,0.3099418872051,-2.017334884313));
#50778=CARTESIAN_POINT('Ctrl Pts',(-3.233351390461,1.647480520897,-2.06337655098));
#50779=CARTESIAN_POINT('Ctrl Pts',(-2.375970535719,2.742894243674,-2.109418217646));
#50780=CARTESIAN_POINT('Ctrl Pts',(-1.16946135002,3.435270189528,-2.155459884313));
#50781=CARTESIAN_POINT('Ctrl Pts',(0.2088925691034,3.622855283072,-2.20150155098));
#50782=CARTESIAN_POINT('Ctrl Pts',(1.556551006228,3.278088863066,-2.247543217646));
#50783=CARTESIAN_POINT('Ctrl Pts',(2.675485639469,2.451630885082,-2.293584884313));
#50784=CARTESIAN_POINT('Ctrl Pts',(3.401277069744,1.264923606363,-2.33962655098));
#50785=CARTESIAN_POINT('Ctrl Pts',(3.627275538361,-0.1076550254197,-2.385668217646));
#50786=CARTESIAN_POINT('Ctrl Pts',(3.320272205746,-1.464414529052,-2.431709884313));
#50787=CARTESIAN_POINT('Ctrl Pts',(2.525378983787,-2.605988952896,-2.47775155098));
#50788=CARTESIAN_POINT('Ctrl Pts',(1.359399658728,-3.364632223854,-2.523793217646));
#50789=CARTESIAN_POINT('Ctrl Pts',(-0.006333574545318,-3.628867222688,-2.569834884313));
#50790=CARTESIAN_POINT('Ctrl Pts',(-1.371136135038,-3.359866535032,-2.61587655098));
#50791=CARTESIAN_POINT('Ctrl Pts',(-2.534460197325,-2.597157858548,-2.661918217646));
#50792=CARTESIAN_POINT('Ctrl Pts',(-3.325363738216,-1.452815694643,-2.707959884313));
#50793=CARTESIAN_POINT('Ctrl Pts',(-3.627629225714,-0.09499281438668,-2.75400155098));
#50794=CARTESIAN_POINT('Ctrl Pts',(-3.396840941408,1.276788570131,-2.800043217646));
#50795=CARTESIAN_POINT('Ctrl Pts',(-2.66691154775,2.460955145979,-2.846084884313));
#50796=CARTESIAN_POINT('Ctrl Pts',(-1.545098868578,3.283502233951,-2.89212655098));
#50797=CARTESIAN_POINT('Ctrl Pts',(-0.1962451307805,3.623562512595,-2.938168217646));
#50798=CARTESIAN_POINT('Ctrl Pts',(1.181445403903,3.431166593396,-2.984209884313));
#50799=CARTESIAN_POINT('Ctrl Pts',(2.385531115837,2.73458565955,-3.03025155098));
#50800=CARTESIAN_POINT('Ctrl Pts',(3.239080353414,1.636177220892,-3.076293217646));
#50801=CARTESIAN_POINT('Ctrl Pts',(3.616670254429,0.2973444211246,-3.122334884313));
#50802=CARTESIAN_POINT('Ctrl Pts',(3.462816724887,-1.085180982089,-3.16837655098));
#50803=CARTESIAN_POINT('Ctrl Pts',(2.80012742371,-2.30824692029,-3.214418217646));
#50804=CARTESIAN_POINT('Ctrl Pts',(1.725979731427,-3.192132735452,-3.260459884313));
#50805=CARTESIAN_POINT('Ctrl Pts',(0.3982118512334,-3.606957825589,-3.30650155098));
#50806=CARTESIAN_POINT('Ctrl Pts',(-0.9880703687869,-3.491766656059,-3.352543217646));
#50807=CARTESIAN_POINT('Ctrl Pts',(-2.229162823228,-2.863485732736,-3.398584884313));
#50808=CARTESIAN_POINT('Ctrl Pts',(-3.142695988404,-1.814436374886,-3.44462655098));
#50809=CARTESIAN_POINT('Ctrl Pts',(-3.594432799537,-0.4987687677191,-3.490668217646));
#50810=CARTESIAN_POINT('Ctrl Pts',(-3.517993812628,0.8901892879335,-3.536709884313));
#50811=CARTESIAN_POINT('Ctrl Pts',(-2.924611181723,2.148340492051,-3.58275155098));
#50812=CARTESIAN_POINT('Ctrl Pts',(-1.90147817544,3.090808661559,-3.628793217646));
#50813=CARTESIAN_POINT('Ctrl Pts',(-0.598936759323,3.579104942911,-3.674834884313));
#50814=CARTESIAN_POINT('Ctrl Pts',(0.791614064251,3.541477743446,-3.72087655098));
#50815=CARTESIAN_POINT('Ctrl Pts',(2.065842949582,2.983456106884,-3.766918217646));
#50816=CARTESIAN_POINT('Ctrl Pts',(3.036511215093,1.98703726051,-3.812959884313));
#50817=CARTESIAN_POINT('Ctrl Pts',(3.560986207913,0.6986377180585,-3.85900155098));
#50818=CARTESIAN_POINT('Ctrl Pts',(3.562200136449,-0.6924215637334,-3.905043217646));
#50819=CARTESIAN_POINT('Ctrl Pts',(3.039974622718,-1.981734524923,-3.951084884313));
#50820=CARTESIAN_POINT('Ctrl Pts',(2.071046913695,-2.979845988523,-3.99712655098));
#50821=CARTESIAN_POINT('Ctrl Pts',(0.7977939001169,-3.540090722987,-4.043168217646));
#50822=CARTESIAN_POINT('Ctrl Pts',(-0.592689133709,-3.58014483294,-4.089209884313));
#50823=CARTESIAN_POINT('Ctrl Pts',(-1.896080803293,-3.094122657786,-4.13525155098));
#50824=CARTESIAN_POINT('Ctrl Pts',(-2.920857167686,-2.153441626797,-4.181293217646));
#50825=CARTESIAN_POINT('Ctrl Pts',(-3.516434781803,-0.8963279864901,-4.227334884313));
#50826=CARTESIAN_POINT('Ctrl Pts',(-3.595297840182,0.4924945425259,-4.27337655098));
#50827=CARTESIAN_POINT('Ctrl Pts',(-3.145857989081,1.808948574891,-4.319418217646));
#50828=CARTESIAN_POINT('Ctrl Pts',(-2.234157150885,2.859590750281,-4.365459884313));
#50829=CARTESIAN_POINT('Ctrl Pts',(-0.9941631432962,3.490036830591,-4.41150155098));
#50830=CARTESIAN_POINT('Ctrl Pts',(0.3919159190425,3.607647342181,-4.457543217646));
#50831=CARTESIAN_POINT('Ctrl Pts',(1.720405782322,3.195140275457,-4.503584884313));
#50832=CARTESIAN_POINT('Ctrl Pts',(2.796094511829,2.313130544526,-4.54962655098));
#50833=CARTESIAN_POINT('Ctrl Pts',(3.460917446918,1.091223088699,-4.595668217646));
#50834=CARTESIAN_POINT('Ctrl Pts',(3.617183734391,-0.2910317178534,-4.641709884313));
#50835=CARTESIAN_POINT('Ctrl Pts',(3.241930993927,-1.630521370031,-4.68775155098));
#50836=CARTESIAN_POINT('Ctrl Pts',(2.390300577984,-2.730418332625,-4.733793217646));
#50837=CARTESIAN_POINT('Ctrl Pts',(1.187430827056,-3.429097964413,-4.779834884313));
#50838=CARTESIAN_POINT('Ctrl Pts',(-0.1899157118936,-3.62390470395,-4.82587655098));
#50839=CARTESIAN_POINT('Ctrl Pts',(-1.539383690082,-3.286174537975,-4.871918217646));
#50840=CARTESIAN_POINT('Ctrl Pts',(-2.288158074621,-2.739177136089,-4.902612662091));
#50841=CARTESIAN_POINT('Ctrl Pts',(-2.59740372034,-2.405222217086,-4.917959884313));
#50842=CARTESIAN_POINT('Ctrl Pts',(-3.381685401913,-1.046806497156,-2.060546319606));
#50843=CARTESIAN_POINT('Ctrl Pts',(-3.516276022629,-0.6120144524515,-2.075893541828));
#50844=CARTESIAN_POINT('Ctrl Pts',(-3.615602476197,0.3099418872051,-2.106587986272));
#50845=CARTESIAN_POINT('Ctrl Pts',(-3.233351390461,1.647480520897,-2.152629652939));
#50846=CARTESIAN_POINT('Ctrl Pts',(-2.375970535719,2.742894243674,-2.198671319606));
#50847=CARTESIAN_POINT('Ctrl Pts',(-1.16946135002,3.435270189528,-2.244712986272));
#50848=CARTESIAN_POINT('Ctrl Pts',(0.2088925691034,3.622855283072,-2.290754652939));
#50849=CARTESIAN_POINT('Ctrl Pts',(1.556551006228,3.278088863066,-2.336796319606));
#50850=CARTESIAN_POINT('Ctrl Pts',(2.675485639469,2.451630885082,-2.382837986272));
#50851=CARTESIAN_POINT('Ctrl Pts',(3.401277069744,1.264923606363,-2.428879652939));
#50852=CARTESIAN_POINT('Ctrl Pts',(3.627275538361,-0.1076550254197,-2.474921319606));
#50853=CARTESIAN_POINT('Ctrl Pts',(3.320272205746,-1.464414529052,-2.520962986272));
#50854=CARTESIAN_POINT('Ctrl Pts',(2.525378983787,-2.605988952896,-2.567004652939));
#50855=CARTESIAN_POINT('Ctrl Pts',(1.359399658728,-3.364632223854,-2.613046319606));
#50856=CARTESIAN_POINT('Ctrl Pts',(-0.006333574545318,-3.628867222688,-2.659087986272));
#50857=CARTESIAN_POINT('Ctrl Pts',(-1.371136135038,-3.359866535032,-2.705129652939));
#50858=CARTESIAN_POINT('Ctrl Pts',(-2.534460197325,-2.597157858548,-2.751171319606));
#50859=CARTESIAN_POINT('Ctrl Pts',(-3.325363738216,-1.452815694643,-2.797212986272));
#50860=CARTESIAN_POINT('Ctrl Pts',(-3.627629225714,-0.09499281438668,-2.843254652939));
#50861=CARTESIAN_POINT('Ctrl Pts',(-3.396840941408,1.276788570131,-2.889296319606));
#50862=CARTESIAN_POINT('Ctrl Pts',(-2.66691154775,2.460955145979,-2.935337986272));
#50863=CARTESIAN_POINT('Ctrl Pts',(-1.545098868578,3.283502233951,-2.981379652939));
#50864=CARTESIAN_POINT('Ctrl Pts',(-0.1962451307805,3.623562512595,-3.027421319606));
#50865=CARTESIAN_POINT('Ctrl Pts',(1.181445403903,3.431166593396,-3.073462986272));
#50866=CARTESIAN_POINT('Ctrl Pts',(2.385531115837,2.73458565955,-3.119504652939));
#50867=CARTESIAN_POINT('Ctrl Pts',(3.239080353414,1.636177220892,-3.165546319606));
#50868=CARTESIAN_POINT('Ctrl Pts',(3.616670254429,0.2973444211246,-3.211587986272));
#50869=CARTESIAN_POINT('Ctrl Pts',(3.462816724887,-1.085180982089,-3.257629652939));
#50870=CARTESIAN_POINT('Ctrl Pts',(2.80012742371,-2.30824692029,-3.303671319606));
#50871=CARTESIAN_POINT('Ctrl Pts',(1.725979731427,-3.192132735452,-3.349712986272));
#50872=CARTESIAN_POINT('Ctrl Pts',(0.3982118512334,-3.606957825589,-3.395754652939));
#50873=CARTESIAN_POINT('Ctrl Pts',(-0.9880703687869,-3.491766656059,-3.441796319606));
#50874=CARTESIAN_POINT('Ctrl Pts',(-2.229162823228,-2.863485732736,-3.487837986272));
#50875=CARTESIAN_POINT('Ctrl Pts',(-3.142695988404,-1.814436374886,-3.533879652939));
#50876=CARTESIAN_POINT('Ctrl Pts',(-3.594432799537,-0.4987687677191,-3.579921319606));
#50877=CARTESIAN_POINT('Ctrl Pts',(-3.517993812628,0.8901892879335,-3.625962986272));
#50878=CARTESIAN_POINT('Ctrl Pts',(-2.924611181723,2.148340492051,-3.672004652939));
#50879=CARTESIAN_POINT('Ctrl Pts',(-1.90147817544,3.090808661559,-3.718046319606));
#50880=CARTESIAN_POINT('Ctrl Pts',(-0.598936759323,3.579104942911,-3.764087986272));
#50881=CARTESIAN_POINT('Ctrl Pts',(0.791614064251,3.541477743446,-3.810129652939));
#50882=CARTESIAN_POINT('Ctrl Pts',(2.065842949582,2.983456106884,-3.856171319606));
#50883=CARTESIAN_POINT('Ctrl Pts',(3.036511215093,1.98703726051,-3.902212986272));
#50884=CARTESIAN_POINT('Ctrl Pts',(3.560986207913,0.6986377180585,-3.948254652939));
#50885=CARTESIAN_POINT('Ctrl Pts',(3.562200136449,-0.6924215637334,-3.994296319606));
#50886=CARTESIAN_POINT('Ctrl Pts',(3.039974622718,-1.981734524923,-4.040337986272));
#50887=CARTESIAN_POINT('Ctrl Pts',(2.071046913695,-2.979845988523,-4.086379652939));
#50888=CARTESIAN_POINT('Ctrl Pts',(0.7977939001169,-3.540090722987,-4.132421319606));
#50889=CARTESIAN_POINT('Ctrl Pts',(-0.592689133709,-3.58014483294,-4.178462986272));
#50890=CARTESIAN_POINT('Ctrl Pts',(-1.896080803293,-3.094122657786,-4.224504652939));
#50891=CARTESIAN_POINT('Ctrl Pts',(-2.920857167686,-2.153441626797,-4.270546319606));
#50892=CARTESIAN_POINT('Ctrl Pts',(-3.516434781803,-0.8963279864901,-4.316587986272));
#50893=CARTESIAN_POINT('Ctrl Pts',(-3.595297840182,0.4924945425259,-4.362629652939));
#50894=CARTESIAN_POINT('Ctrl Pts',(-3.145857989081,1.808948574891,-4.408671319606));
#50895=CARTESIAN_POINT('Ctrl Pts',(-2.234157150885,2.859590750281,-4.454712986272));
#50896=CARTESIAN_POINT('Ctrl Pts',(-0.9941631432962,3.490036830591,-4.500754652939));
#50897=CARTESIAN_POINT('Ctrl Pts',(0.3919159190425,3.607647342181,-4.546796319606));
#50898=CARTESIAN_POINT('Ctrl Pts',(1.720405782322,3.195140275457,-4.592837986272));
#50899=CARTESIAN_POINT('Ctrl Pts',(2.796094511829,2.313130544526,-4.638879652939));
#50900=CARTESIAN_POINT('Ctrl Pts',(3.460917446918,1.091223088699,-4.684921319606));
#50901=CARTESIAN_POINT('Ctrl Pts',(3.617183734391,-0.2910317178534,-4.730962986272));
#50902=CARTESIAN_POINT('Ctrl Pts',(3.241930993927,-1.630521370031,-4.777004652939));
#50903=CARTESIAN_POINT('Ctrl Pts',(2.390300577984,-2.730418332625,-4.823046319606));
#50904=CARTESIAN_POINT('Ctrl Pts',(1.187430827056,-3.429097964413,-4.869087986272));
#50905=CARTESIAN_POINT('Ctrl Pts',(-0.1899157118936,-3.62390470395,-4.915129652939));
#50906=CARTESIAN_POINT('Ctrl Pts',(-1.539383690082,-3.286174537975,-4.961171319606));
#50907=CARTESIAN_POINT('Ctrl Pts',(-2.288158074621,-2.739177136089,-4.99186576405));
#50908=CARTESIAN_POINT('Ctrl Pts',(-2.59740372034,-2.405222217086,-5.007212986272));
#50909=CARTESIAN_POINT('',(-1.210751307373,-3.326511877582,-4.707247790494));
#50910=CARTESIAN_POINT('Ctrl Pts',(0.4436796468176,-3.512086042653,-4.626120347061));
#50911=CARTESIAN_POINT('Ctrl Pts',(-0.007878345773629,-3.56913108319,-4.641467569283));
#50912=CARTESIAN_POINT('Ctrl Pts',(-0.9330759546625,-3.506852506473,-4.672162013728));
#50913=CARTESIAN_POINT('Ctrl Pts',(-2.183917166627,-2.898147527343,-4.718203680394));
#50914=CARTESIAN_POINT('Ctrl Pts',(-3.113806470581,-1.863575617557,-4.764245347061));
#50915=CARTESIAN_POINT('Ctrl Pts',(-3.586155548622,-0.555166196143,-4.810287013728));
#50916=CARTESIAN_POINT('Ctrl Pts',(-3.531542156858,0.8348212394562,-4.856328680394));
#50917=CARTESIAN_POINT('Ctrl Pts',(-2.957995081733,2.102137656194,-4.902370347061));
#50918=CARTESIAN_POINT('Ctrl Pts',(-1.949791897485,3.060560236328,-4.948412013728));
#50919=CARTESIAN_POINT('Ctrl Pts',(-0.6550810096133,3.56925570756,-4.994453680394));
#50920=CARTESIAN_POINT('Ctrl Pts',(0.7358892908163,3.553474973509,-5.040495347061));
#50921=CARTESIAN_POINT('Ctrl Pts',(2.01872599972,3.01553689601,-5.086537013728));
#50922=CARTESIAN_POINT('Ctrl Pts',(3.004925583529,2.034487569837,-5.132578680394));
#50923=CARTESIAN_POINT('Ctrl Pts',(3.549573173545,0.754485069166,-5.178620347061));
#50924=CARTESIAN_POINT('Ctrl Pts',(3.572636761877,-0.6363835335316,-5.224662013728));
#50925=CARTESIAN_POINT('Ctrl Pts',(3.070727321603,-1.933740197233,-5.270703680394));
#50926=CARTESIAN_POINT('Ctrl Pts',(2.11759680026,-2.946947781277,-5.316745347061));
#50927=CARTESIAN_POINT('Ctrl Pts',(0.8533008065619,-3.527122788841,-5.362787013728));
#50928=CARTESIAN_POINT('Ctrl Pts',(-0.5363815442081,-3.589012715647,-5.408828680394));
#50929=CARTESIAN_POINT('Ctrl Pts',(-1.847246522122,-3.123523286379,-5.454870347061));
#50930=CARTESIAN_POINT('Ctrl Pts',(-2.886672037841,-2.199054792402,-5.500912013728));
#50931=CARTESIAN_POINT('Ctrl Pts',(-3.501922059872,-0.9514511656551,-5.546953680394));
#50932=CARTESIAN_POINT('Ctrl Pts',(-3.602590065264,0.4359613006909,-5.592995347061));
#50933=CARTESIAN_POINT('Ctrl Pts',(-3.173883621652,1.75931241974,-5.639037013728));
#50934=CARTESIAN_POINT('Ctrl Pts',(-2.278798027768,2.824145354383,-5.685078680394));
#50935=CARTESIAN_POINT('Ctrl Pts',(-1.04885961175,3.47399063742,-5.731120347061));
#50936=CARTESIAN_POINT('Ctrl Pts',(0.3352011076653,3.613358223518,-5.777162013728));
#50937=CARTESIAN_POINT('Ctrl Pts',(1.670006458453,3.22176905795,-5.823203680394));
#50938=CARTESIAN_POINT('Ctrl Pts',(2.75941648733,2.356764324978,-5.869245347061));
#50939=CARTESIAN_POINT('Ctrl Pts',(3.44335030157,1.145450188669,-5.915287013728));
#50940=CARTESIAN_POINT('Ctrl Pts',(3.62130879372,-0.2341795348991,-5.961328680394));
#50941=CARTESIAN_POINT('Ctrl Pts',(3.26714225565,-1.579398276366,-6.007370347061));
#50942=CARTESIAN_POINT('Ctrl Pts',(2.432892888262,-2.692535910306,-6.053412013728));
#50943=CARTESIAN_POINT('Ctrl Pts',(1.241147577988,-3.410024944732,-6.099453680394));
#50944=CARTESIAN_POINT('Ctrl Pts',(-0.1329753559758,-3.626435576257,-6.145495347061));
#50945=CARTESIAN_POINT('Ctrl Pts',(-1.487558527012,-3.309967834097,-6.191537013728));
#50946=CARTESIAN_POINT('Ctrl Pts',(-2.623555774772,-2.507124354854,-6.237578680394));
#50947=CARTESIAN_POINT('Ctrl Pts',(-3.374040553019,-1.33587715776,-6.283620347061));
#50948=CARTESIAN_POINT('Ctrl Pts',(-3.628734573418,0.03166748686997,-6.329662013728));
#50949=CARTESIAN_POINT('Ctrl Pts',(-3.350212399193,1.394558824265,-6.375703680394));
#50950=CARTESIAN_POINT('Ctrl Pts',(-2.57940084129,2.552529869363,-6.421745347061));
#50951=CARTESIAN_POINT('Ctrl Pts',(-1.429565060708,3.335425185976,-6.467787013728));
#50952=CARTESIAN_POINT('Ctrl Pts',(-0.06966507558956,3.628203992513,-6.513828680394));
#50953=CARTESIAN_POINT('Ctrl Pts',(1.300471686497,3.387844569437,-6.559870347061));
#50954=CARTESIAN_POINT('Ctrl Pts',(2.479513577945,2.649665988541,-6.605912013728));
#50955=CARTESIAN_POINT('Ctrl Pts',(3.294208954705,1.522138231824,-6.651953680394));
#50956=CARTESIAN_POINT('Ctrl Pts',(3.624844247273,0.1709433153187,-6.697995347061));
#50957=CARTESIAN_POINT('Ctrl Pts',(3.422835000394,-1.205370480026,-6.744037013728));
#50958=CARTESIAN_POINT('Ctrl Pts',(2.717865005957,-2.404563836423,-6.790078680394));
#50959=CARTESIAN_POINT('Ctrl Pts',(1.613524485334,-3.250423998384,-6.836120347061));
#50960=CARTESIAN_POINT('Ctrl Pts',(0.2720882585925,-3.618657957528,-6.882162013728));
#50961=CARTESIAN_POINT('Ctrl Pts',(-1.109329361913,-3.455156407579,-6.928203680394));
#50962=CARTESIAN_POINT('Ctrl Pts',(-2.327739088356,-2.783944714,-6.974245347061));
#50963=CARTESIAN_POINT('Ctrl Pts',(-3.204104459192,-1.70365256098,-7.020287013728));
#50964=CARTESIAN_POINT('Ctrl Pts',(-3.609649947201,-0.3730210356546,-7.066328680394));
#50965=CARTESIAN_POINT('Ctrl Pts',(-3.484783587573,1.012423222237,-7.112370347061));
#50966=CARTESIAN_POINT('Ctrl Pts',(-2.847853586283,2.249099238981,-7.158412013728));
#50967=CARTESIAN_POINT('Ctrl Pts',(-1.792452177415,3.155286457167,-7.204453680394));
#50968=CARTESIAN_POINT('Ctrl Pts',(-0.4736629503042,3.597827235041,-7.250495347061));
#50969=CARTESIAN_POINT('Ctrl Pts',(0.9147276558781,3.51169345825,-7.296537013728));
#50970=CARTESIAN_POINT('Ctrl Pts',(2.168705495876,2.909541712997,-7.342578680394));
#50971=CARTESIAN_POINT('Ctrl Pts',(3.104008482379,1.8798543735,-7.388620347061));
#50972=CARTESIAN_POINT('Ctrl Pts',(3.583197460416,0.5739344720891,-7.434662013728));
#50973=CARTESIAN_POINT('Ctrl Pts',(3.535870931347,-0.8163149133711,-7.480703680394));
#50974=CARTESIAN_POINT('Ctrl Pts',(2.968938990236,-2.086635212868,-7.526745347061));
#50975=CARTESIAN_POINT('Ctrl Pts',(2.300228400622,-2.729048929993,-7.557439791506));
#50976=CARTESIAN_POINT('Ctrl Pts',(1.917647064401,-2.975605776375,-7.572787013728));
#50977=CARTESIAN_POINT('Ctrl Pts',(0.4436796468176,-3.512086042653,-4.71537344902));
#50978=CARTESIAN_POINT('Ctrl Pts',(-0.007878345773629,-3.56913108319,-4.730720671243));
#50979=CARTESIAN_POINT('Ctrl Pts',(-0.9330759546625,-3.506852506473,-4.761415115687));
#50980=CARTESIAN_POINT('Ctrl Pts',(-2.183917166627,-2.898147527343,-4.807456782354));
#50981=CARTESIAN_POINT('Ctrl Pts',(-3.113806470581,-1.863575617557,-4.85349844902));
#50982=CARTESIAN_POINT('Ctrl Pts',(-3.586155548622,-0.555166196143,-4.899540115687));
#50983=CARTESIAN_POINT('Ctrl Pts',(-3.531542156858,0.8348212394562,-4.945581782354));
#50984=CARTESIAN_POINT('Ctrl Pts',(-2.957995081733,2.102137656194,-4.99162344902));
#50985=CARTESIAN_POINT('Ctrl Pts',(-1.949791897485,3.060560236328,-5.037665115687));
#50986=CARTESIAN_POINT('Ctrl Pts',(-0.6550810096133,3.56925570756,-5.083706782354));
#50987=CARTESIAN_POINT('Ctrl Pts',(0.7358892908163,3.553474973509,-5.12974844902));
#50988=CARTESIAN_POINT('Ctrl Pts',(2.01872599972,3.01553689601,-5.175790115687));
#50989=CARTESIAN_POINT('Ctrl Pts',(3.004925583529,2.034487569837,-5.221831782354));
#50990=CARTESIAN_POINT('Ctrl Pts',(3.549573173545,0.754485069166,-5.26787344902));
#50991=CARTESIAN_POINT('Ctrl Pts',(3.572636761877,-0.6363835335316,-5.313915115687));
#50992=CARTESIAN_POINT('Ctrl Pts',(3.070727321603,-1.933740197233,-5.359956782354));
#50993=CARTESIAN_POINT('Ctrl Pts',(2.11759680026,-2.946947781277,-5.40599844902));
#50994=CARTESIAN_POINT('Ctrl Pts',(0.8533008065619,-3.527122788841,-5.452040115687));
#50995=CARTESIAN_POINT('Ctrl Pts',(-0.5363815442081,-3.589012715647,-5.498081782354));
#50996=CARTESIAN_POINT('Ctrl Pts',(-1.847246522122,-3.123523286379,-5.54412344902));
#50997=CARTESIAN_POINT('Ctrl Pts',(-2.886672037841,-2.199054792402,-5.590165115687));
#50998=CARTESIAN_POINT('Ctrl Pts',(-3.501922059872,-0.9514511656551,-5.636206782354));
#50999=CARTESIAN_POINT('Ctrl Pts',(-3.602590065264,0.4359613006909,-5.68224844902));
#51000=CARTESIAN_POINT('Ctrl Pts',(-3.173883621652,1.75931241974,-5.728290115687));
#51001=CARTESIAN_POINT('Ctrl Pts',(-2.278798027768,2.824145354383,-5.774331782354));
#51002=CARTESIAN_POINT('Ctrl Pts',(-1.04885961175,3.47399063742,-5.82037344902));
#51003=CARTESIAN_POINT('Ctrl Pts',(0.3352011076653,3.613358223518,-5.866415115687));
#51004=CARTESIAN_POINT('Ctrl Pts',(1.670006458453,3.22176905795,-5.912456782354));
#51005=CARTESIAN_POINT('Ctrl Pts',(2.75941648733,2.356764324978,-5.95849844902));
#51006=CARTESIAN_POINT('Ctrl Pts',(3.44335030157,1.145450188669,-6.004540115687));
#51007=CARTESIAN_POINT('Ctrl Pts',(3.62130879372,-0.2341795348991,-6.050581782354));
#51008=CARTESIAN_POINT('Ctrl Pts',(3.26714225565,-1.579398276366,-6.09662344902));
#51009=CARTESIAN_POINT('Ctrl Pts',(2.432892888262,-2.692535910306,-6.142665115687));
#51010=CARTESIAN_POINT('Ctrl Pts',(1.241147577988,-3.410024944732,-6.188706782354));
#51011=CARTESIAN_POINT('Ctrl Pts',(-0.1329753559758,-3.626435576257,-6.23474844902));
#51012=CARTESIAN_POINT('Ctrl Pts',(-1.487558527012,-3.309967834097,-6.280790115687));
#51013=CARTESIAN_POINT('Ctrl Pts',(-2.623555774772,-2.507124354854,-6.326831782354));
#51014=CARTESIAN_POINT('Ctrl Pts',(-3.374040553019,-1.33587715776,-6.37287344902));
#51015=CARTESIAN_POINT('Ctrl Pts',(-3.628734573418,0.03166748686997,-6.418915115687));
#51016=CARTESIAN_POINT('Ctrl Pts',(-3.350212399193,1.394558824265,-6.464956782354));
#51017=CARTESIAN_POINT('Ctrl Pts',(-2.57940084129,2.552529869363,-6.51099844902));
#51018=CARTESIAN_POINT('Ctrl Pts',(-1.429565060708,3.335425185976,-6.557040115687));
#51019=CARTESIAN_POINT('Ctrl Pts',(-0.06966507558956,3.628203992513,-6.603081782354));
#51020=CARTESIAN_POINT('Ctrl Pts',(1.300471686497,3.387844569437,-6.64912344902));
#51021=CARTESIAN_POINT('Ctrl Pts',(2.479513577945,2.649665988541,-6.695165115687));
#51022=CARTESIAN_POINT('Ctrl Pts',(3.294208954705,1.522138231824,-6.741206782354));
#51023=CARTESIAN_POINT('Ctrl Pts',(3.624844247273,0.1709433153187,-6.78724844902));
#51024=CARTESIAN_POINT('Ctrl Pts',(3.422835000394,-1.205370480026,-6.833290115687));
#51025=CARTESIAN_POINT('Ctrl Pts',(2.717865005957,-2.404563836423,-6.879331782354));
#51026=CARTESIAN_POINT('Ctrl Pts',(1.613524485334,-3.250423998384,-6.92537344902));
#51027=CARTESIAN_POINT('Ctrl Pts',(0.2720882585925,-3.618657957528,-6.971415115687));
#51028=CARTESIAN_POINT('Ctrl Pts',(-1.109329361913,-3.455156407579,-7.017456782354));
#51029=CARTESIAN_POINT('Ctrl Pts',(-2.327739088356,-2.783944714,-7.06349844902));
#51030=CARTESIAN_POINT('Ctrl Pts',(-3.204104459192,-1.70365256098,-7.109540115687));
#51031=CARTESIAN_POINT('Ctrl Pts',(-3.609649947201,-0.3730210356546,-7.155581782354));
#51032=CARTESIAN_POINT('Ctrl Pts',(-3.484783587573,1.012423222237,-7.20162344902));
#51033=CARTESIAN_POINT('Ctrl Pts',(-2.847853586283,2.249099238981,-7.247665115687));
#51034=CARTESIAN_POINT('Ctrl Pts',(-1.792452177415,3.155286457167,-7.293706782354));
#51035=CARTESIAN_POINT('Ctrl Pts',(-0.4736629503042,3.597827235041,-7.33974844902));
#51036=CARTESIAN_POINT('Ctrl Pts',(0.9147276558781,3.51169345825,-7.385790115687));
#51037=CARTESIAN_POINT('Ctrl Pts',(2.168705495876,2.909541712997,-7.431831782354));
#51038=CARTESIAN_POINT('Ctrl Pts',(3.104008482379,1.8798543735,-7.47787344902));
#51039=CARTESIAN_POINT('Ctrl Pts',(3.583197460416,0.5739344720891,-7.523915115687));
#51040=CARTESIAN_POINT('Ctrl Pts',(3.535870931347,-0.8163149133711,-7.569956782354));
#51041=CARTESIAN_POINT('Ctrl Pts',(2.968938990236,-2.086635212868,-7.61599844902));
#51042=CARTESIAN_POINT('Ctrl Pts',(2.300228400622,-2.729048929993,-7.646692893465));
#51043=CARTESIAN_POINT('Ctrl Pts',(1.917647064401,-2.975605776375,-7.662040115687));
#51044=CARTESIAN_POINT('Ctrl Pts',(0.4436796468176,-3.512086042653,-4.80462655098));
#51045=CARTESIAN_POINT('Ctrl Pts',(-0.007878345773629,-3.56913108319,-4.819973773202));
#51046=CARTESIAN_POINT('Ctrl Pts',(-0.9330759546625,-3.506852506473,-4.850668217646));
#51047=CARTESIAN_POINT('Ctrl Pts',(-2.183917166627,-2.898147527343,-4.896709884313));
#51048=CARTESIAN_POINT('Ctrl Pts',(-3.113806470581,-1.863575617557,-4.94275155098));
#51049=CARTESIAN_POINT('Ctrl Pts',(-3.586155548622,-0.555166196143,-4.988793217646));
#51050=CARTESIAN_POINT('Ctrl Pts',(-3.531542156858,0.8348212394562,-5.034834884313));
#51051=CARTESIAN_POINT('Ctrl Pts',(-2.957995081733,2.102137656194,-5.08087655098));
#51052=CARTESIAN_POINT('Ctrl Pts',(-1.949791897485,3.060560236328,-5.126918217646));
#51053=CARTESIAN_POINT('Ctrl Pts',(-0.6550810096133,3.56925570756,-5.172959884313));
#51054=CARTESIAN_POINT('Ctrl Pts',(0.7358892908163,3.553474973509,-5.21900155098));
#51055=CARTESIAN_POINT('Ctrl Pts',(2.01872599972,3.01553689601,-5.265043217646));
#51056=CARTESIAN_POINT('Ctrl Pts',(3.004925583529,2.034487569837,-5.311084884313));
#51057=CARTESIAN_POINT('Ctrl Pts',(3.549573173545,0.754485069166,-5.35712655098));
#51058=CARTESIAN_POINT('Ctrl Pts',(3.572636761877,-0.6363835335316,-5.403168217646));
#51059=CARTESIAN_POINT('Ctrl Pts',(3.070727321603,-1.933740197233,-5.449209884313));
#51060=CARTESIAN_POINT('Ctrl Pts',(2.11759680026,-2.946947781277,-5.49525155098));
#51061=CARTESIAN_POINT('Ctrl Pts',(0.8533008065619,-3.527122788841,-5.541293217646));
#51062=CARTESIAN_POINT('Ctrl Pts',(-0.5363815442082,-3.589012715647,-5.587334884313));
#51063=CARTESIAN_POINT('Ctrl Pts',(-1.847246522122,-3.123523286379,-5.63337655098));
#51064=CARTESIAN_POINT('Ctrl Pts',(-2.886672037841,-2.199054792402,-5.679418217646));
#51065=CARTESIAN_POINT('Ctrl Pts',(-3.501922059872,-0.9514511656551,-5.725459884313));
#51066=CARTESIAN_POINT('Ctrl Pts',(-3.602590065264,0.4359613006909,-5.77150155098));
#51067=CARTESIAN_POINT('Ctrl Pts',(-3.173883621652,1.75931241974,-5.817543217646));
#51068=CARTESIAN_POINT('Ctrl Pts',(-2.278798027768,2.824145354383,-5.863584884313));
#51069=CARTESIAN_POINT('Ctrl Pts',(-1.04885961175,3.47399063742,-5.90962655098));
#51070=CARTESIAN_POINT('Ctrl Pts',(0.3352011076653,3.613358223518,-5.955668217646));
#51071=CARTESIAN_POINT('Ctrl Pts',(1.670006458453,3.22176905795,-6.001709884313));
#51072=CARTESIAN_POINT('Ctrl Pts',(2.75941648733,2.356764324978,-6.04775155098));
#51073=CARTESIAN_POINT('Ctrl Pts',(3.44335030157,1.145450188669,-6.093793217646));
#51074=CARTESIAN_POINT('Ctrl Pts',(3.62130879372,-0.2341795348991,-6.139834884313));
#51075=CARTESIAN_POINT('Ctrl Pts',(3.26714225565,-1.579398276366,-6.18587655098));
#51076=CARTESIAN_POINT('Ctrl Pts',(2.432892888262,-2.692535910306,-6.231918217646));
#51077=CARTESIAN_POINT('Ctrl Pts',(1.241147577988,-3.410024944732,-6.277959884313));
#51078=CARTESIAN_POINT('Ctrl Pts',(-0.1329753559758,-3.626435576257,-6.32400155098));
#51079=CARTESIAN_POINT('Ctrl Pts',(-1.487558527012,-3.309967834097,-6.370043217646));
#51080=CARTESIAN_POINT('Ctrl Pts',(-2.623555774772,-2.507124354854,-6.416084884313));
#51081=CARTESIAN_POINT('Ctrl Pts',(-3.374040553019,-1.33587715776,-6.46212655098));
#51082=CARTESIAN_POINT('Ctrl Pts',(-3.628734573418,0.03166748686998,-6.508168217646));
#51083=CARTESIAN_POINT('Ctrl Pts',(-3.350212399193,1.394558824265,-6.554209884313));
#51084=CARTESIAN_POINT('Ctrl Pts',(-2.57940084129,2.552529869363,-6.60025155098));
#51085=CARTESIAN_POINT('Ctrl Pts',(-1.429565060708,3.335425185976,-6.646293217646));
#51086=CARTESIAN_POINT('Ctrl Pts',(-0.06966507558957,3.628203992513,-6.692334884313));
#51087=CARTESIAN_POINT('Ctrl Pts',(1.300471686497,3.387844569437,-6.73837655098));
#51088=CARTESIAN_POINT('Ctrl Pts',(2.479513577945,2.649665988541,-6.784418217646));
#51089=CARTESIAN_POINT('Ctrl Pts',(3.294208954705,1.522138231824,-6.830459884313));
#51090=CARTESIAN_POINT('Ctrl Pts',(3.624844247273,0.1709433153187,-6.87650155098));
#51091=CARTESIAN_POINT('Ctrl Pts',(3.422835000394,-1.205370480026,-6.922543217646));
#51092=CARTESIAN_POINT('Ctrl Pts',(2.717865005957,-2.404563836423,-6.968584884313));
#51093=CARTESIAN_POINT('Ctrl Pts',(1.613524485334,-3.250423998384,-7.01462655098));
#51094=CARTESIAN_POINT('Ctrl Pts',(0.2720882585925,-3.618657957528,-7.060668217646));
#51095=CARTESIAN_POINT('Ctrl Pts',(-1.109329361913,-3.455156407579,-7.106709884313));
#51096=CARTESIAN_POINT('Ctrl Pts',(-2.327739088356,-2.783944714,-7.15275155098));
#51097=CARTESIAN_POINT('Ctrl Pts',(-3.204104459192,-1.70365256098,-7.198793217646));
#51098=CARTESIAN_POINT('Ctrl Pts',(-3.609649947201,-0.3730210356546,-7.244834884313));
#51099=CARTESIAN_POINT('Ctrl Pts',(-3.484783587573,1.012423222237,-7.29087655098));
#51100=CARTESIAN_POINT('Ctrl Pts',(-2.847853586283,2.249099238981,-7.336918217646));
#51101=CARTESIAN_POINT('Ctrl Pts',(-1.792452177415,3.155286457167,-7.382959884313));
#51102=CARTESIAN_POINT('Ctrl Pts',(-0.4736629503042,3.597827235041,-7.42900155098));
#51103=CARTESIAN_POINT('Ctrl Pts',(0.9147276558781,3.51169345825,-7.475043217646));
#51104=CARTESIAN_POINT('Ctrl Pts',(2.168705495876,2.909541712997,-7.521084884313));
#51105=CARTESIAN_POINT('Ctrl Pts',(3.104008482379,1.8798543735,-7.56712655098));
#51106=CARTESIAN_POINT('Ctrl Pts',(3.583197460416,0.5739344720891,-7.613168217646));
#51107=CARTESIAN_POINT('Ctrl Pts',(3.535870931347,-0.8163149133711,-7.659209884313));
#51108=CARTESIAN_POINT('Ctrl Pts',(2.968938990236,-2.086635212868,-7.70525155098));
#51109=CARTESIAN_POINT('Ctrl Pts',(2.300228400622,-2.729048929993,-7.735945995424));
#51110=CARTESIAN_POINT('Ctrl Pts',(1.917647064401,-2.975605776375,-7.751293217646));
#51111=CARTESIAN_POINT('Ctrl Pts',(0.4436796468176,-3.512086042653,-4.893879652939));
#51112=CARTESIAN_POINT('Ctrl Pts',(-0.007878345773629,-3.56913108319,-4.909226875161));
#51113=CARTESIAN_POINT('Ctrl Pts',(-0.9330759546625,-3.506852506473,-4.939921319606));
#51114=CARTESIAN_POINT('Ctrl Pts',(-2.183917166627,-2.898147527343,-4.985962986272));
#51115=CARTESIAN_POINT('Ctrl Pts',(-3.113806470581,-1.863575617557,-5.032004652939));
#51116=CARTESIAN_POINT('Ctrl Pts',(-3.586155548622,-0.555166196143,-5.078046319606));
#51117=CARTESIAN_POINT('Ctrl Pts',(-3.531542156858,0.8348212394562,-5.124087986272));
#51118=CARTESIAN_POINT('Ctrl Pts',(-2.957995081733,2.102137656194,-5.170129652939));
#51119=CARTESIAN_POINT('Ctrl Pts',(-1.949791897485,3.060560236328,-5.216171319606));
#51120=CARTESIAN_POINT('Ctrl Pts',(-0.6550810096133,3.56925570756,-5.262212986272));
#51121=CARTESIAN_POINT('Ctrl Pts',(0.7358892908163,3.553474973509,-5.308254652939));
#51122=CARTESIAN_POINT('Ctrl Pts',(2.01872599972,3.01553689601,-5.354296319606));
#51123=CARTESIAN_POINT('Ctrl Pts',(3.004925583529,2.034487569837,-5.400337986272));
#51124=CARTESIAN_POINT('Ctrl Pts',(3.549573173545,0.754485069166,-5.446379652939));
#51125=CARTESIAN_POINT('Ctrl Pts',(3.572636761877,-0.6363835335316,-5.492421319606));
#51126=CARTESIAN_POINT('Ctrl Pts',(3.070727321603,-1.933740197233,-5.538462986272));
#51127=CARTESIAN_POINT('Ctrl Pts',(2.11759680026,-2.946947781277,-5.584504652939));
#51128=CARTESIAN_POINT('Ctrl Pts',(0.8533008065619,-3.527122788841,-5.630546319606));
#51129=CARTESIAN_POINT('Ctrl Pts',(-0.5363815442082,-3.589012715647,-5.676587986272));
#51130=CARTESIAN_POINT('Ctrl Pts',(-1.847246522122,-3.123523286379,-5.722629652939));
#51131=CARTESIAN_POINT('Ctrl Pts',(-2.886672037841,-2.199054792402,-5.768671319606));
#51132=CARTESIAN_POINT('Ctrl Pts',(-3.501922059872,-0.9514511656551,-5.814712986272));
#51133=CARTESIAN_POINT('Ctrl Pts',(-3.602590065264,0.4359613006909,-5.860754652939));
#51134=CARTESIAN_POINT('Ctrl Pts',(-3.173883621652,1.75931241974,-5.906796319606));
#51135=CARTESIAN_POINT('Ctrl Pts',(-2.278798027768,2.824145354383,-5.952837986272));
#51136=CARTESIAN_POINT('Ctrl Pts',(-1.04885961175,3.47399063742,-5.998879652939));
#51137=CARTESIAN_POINT('Ctrl Pts',(0.3352011076653,3.613358223518,-6.044921319606));
#51138=CARTESIAN_POINT('Ctrl Pts',(1.670006458453,3.22176905795,-6.090962986272));
#51139=CARTESIAN_POINT('Ctrl Pts',(2.75941648733,2.356764324978,-6.137004652939));
#51140=CARTESIAN_POINT('Ctrl Pts',(3.44335030157,1.145450188669,-6.183046319606));
#51141=CARTESIAN_POINT('Ctrl Pts',(3.62130879372,-0.2341795348991,-6.229087986272));
#51142=CARTESIAN_POINT('Ctrl Pts',(3.26714225565,-1.579398276366,-6.275129652939));
#51143=CARTESIAN_POINT('Ctrl Pts',(2.432892888262,-2.692535910306,-6.321171319606));
#51144=CARTESIAN_POINT('Ctrl Pts',(1.241147577988,-3.410024944732,-6.367212986272));
#51145=CARTESIAN_POINT('Ctrl Pts',(-0.1329753559758,-3.626435576257,-6.413254652939));
#51146=CARTESIAN_POINT('Ctrl Pts',(-1.487558527012,-3.309967834097,-6.459296319606));
#51147=CARTESIAN_POINT('Ctrl Pts',(-2.623555774772,-2.507124354854,-6.505337986272));
#51148=CARTESIAN_POINT('Ctrl Pts',(-3.374040553019,-1.33587715776,-6.551379652939));
#51149=CARTESIAN_POINT('Ctrl Pts',(-3.628734573418,0.03166748686998,-6.597421319606));
#51150=CARTESIAN_POINT('Ctrl Pts',(-3.350212399193,1.394558824265,-6.643462986272));
#51151=CARTESIAN_POINT('Ctrl Pts',(-2.57940084129,2.552529869363,-6.689504652939));
#51152=CARTESIAN_POINT('Ctrl Pts',(-1.429565060708,3.335425185976,-6.735546319606));
#51153=CARTESIAN_POINT('Ctrl Pts',(-0.06966507558957,3.628203992513,-6.781587986272));
#51154=CARTESIAN_POINT('Ctrl Pts',(1.300471686497,3.387844569437,-6.827629652939));
#51155=CARTESIAN_POINT('Ctrl Pts',(2.479513577945,2.649665988541,-6.873671319606));
#51156=CARTESIAN_POINT('Ctrl Pts',(3.294208954705,1.522138231824,-6.919712986272));
#51157=CARTESIAN_POINT('Ctrl Pts',(3.624844247273,0.1709433153187,-6.965754652939));
#51158=CARTESIAN_POINT('Ctrl Pts',(3.422835000394,-1.205370480026,-7.011796319606));
#51159=CARTESIAN_POINT('Ctrl Pts',(2.717865005957,-2.404563836423,-7.057837986272));
#51160=CARTESIAN_POINT('Ctrl Pts',(1.613524485334,-3.250423998384,-7.103879652939));
#51161=CARTESIAN_POINT('Ctrl Pts',(0.2720882585925,-3.618657957528,-7.149921319606));
#51162=CARTESIAN_POINT('Ctrl Pts',(-1.109329361913,-3.455156407579,-7.195962986272));
#51163=CARTESIAN_POINT('Ctrl Pts',(-2.327739088356,-2.783944714,-7.242004652939));
#51164=CARTESIAN_POINT('Ctrl Pts',(-3.204104459192,-1.70365256098,-7.288046319606));
#51165=CARTESIAN_POINT('Ctrl Pts',(-3.609649947201,-0.3730210356546,-7.334087986272));
#51166=CARTESIAN_POINT('Ctrl Pts',(-3.484783587573,1.012423222237,-7.380129652939));
#51167=CARTESIAN_POINT('Ctrl Pts',(-2.847853586283,2.249099238981,-7.426171319606));
#51168=CARTESIAN_POINT('Ctrl Pts',(-1.792452177415,3.155286457167,-7.472212986272));
#51169=CARTESIAN_POINT('Ctrl Pts',(-0.4736629503042,3.597827235041,-7.518254652939));
#51170=CARTESIAN_POINT('Ctrl Pts',(0.9147276558781,3.51169345825,-7.564296319606));
#51171=CARTESIAN_POINT('Ctrl Pts',(2.168705495876,2.909541712997,-7.610337986272));
#51172=CARTESIAN_POINT('Ctrl Pts',(3.104008482379,1.8798543735,-7.656379652939));
#51173=CARTESIAN_POINT('Ctrl Pts',(3.583197460416,0.5739344720891,-7.702421319606));
#51174=CARTESIAN_POINT('Ctrl Pts',(3.535870931347,-0.8163149133711,-7.748462986272));
#51175=CARTESIAN_POINT('Ctrl Pts',(2.968938990236,-2.086635212868,-7.794504652939));
#51176=CARTESIAN_POINT('Ctrl Pts',(2.300228400622,-2.729048929993,-7.825199097383));
#51177=CARTESIAN_POINT('Ctrl Pts',(1.917647064401,-2.975605776375,-7.840546319606));
#51178=CARTESIAN_POINT('Ctrl Pts',(-1.2107138361353,-3.32640900638413,-4.92608554369097));
#51179=CARTESIAN_POINT('Ctrl Pts',(-1.39219287791354,-3.26025710999361,
-4.93259895336898));
#51180=CARTESIAN_POINT('Ctrl Pts',(-1.56825188018812,-3.17927104787258,
-4.93911236304649));
#51181=CARTESIAN_POINT('Ctrl Pts',(-1.73659924449935,-3.08457088033829,
-4.94562577272425));
#51182=CARTESIAN_POINT('Ctrl Pts',(-1.87338108397249,-3.00762721586959,
-4.9509179028423));
#51183=CARTESIAN_POINT('Ctrl Pts',(-2.00508361696359,-2.92162011815734,
-4.95621003296051));
#51184=CARTESIAN_POINT('Ctrl Pts',(-2.13042518195858,-2.827169705567,-4.96150216307867));
#51185=CARTESIAN_POINT('Ctrl Pts',(-2.15935060962041,-2.80537311656542,
-4.9627234429224));
#51186=CARTESIAN_POINT('Ctrl Pts',(-2.18793730334398,-2.78312691895196,
-4.96394472276613));
#51187=CARTESIAN_POINT('Ctrl Pts',(-2.21617354772985,-2.76044407979828,
-4.96516600260984));
#51188=CARTESIAN_POINT('Ctrl Pts',(-2.36676494282521,-2.63947047062431,
-4.97167941257167));
#51189=CARTESIAN_POINT('Ctrl Pts',(-2.50737055352154,-2.50609287961651,
-4.97819282253333));
#51190=CARTESIAN_POINT('Ctrl Pts',(-2.63627091172052,-2.36224216903429,
-4.98470623249499));
#51191=CARTESIAN_POINT('Ctrl Pts',(-2.76517126991969,-2.21839145845186,
-4.99121964245666));
#51192=CARTESIAN_POINT('Ctrl Pts',(-2.88238227181575,-2.06404968982843,
-4.99773305241833));
#51193=CARTESIAN_POINT('Ctrl Pts',(-2.98616562034842,-1.90113425254753,
-5.00424646238));
#51194=CARTESIAN_POINT('Ctrl Pts',(-3.0036792827206,-1.87364192353623,-5.00534561426297));
#51195=CARTESIAN_POINT('Ctrl Pts',(-3.02081015796238,-1.84590601958711,
-5.00644476614593));
#51196=CARTESIAN_POINT('Ctrl Pts',(-3.03754976626217,-1.81793603228567,
-5.0075439180289));
#51197=CARTESIAN_POINT('Ctrl Pts',(-3.12000657762367,-1.6801600505903,-5.0129581761076));
#51198=CARTESIAN_POINT('Ctrl Pts',(-3.1929686605663,-1.53670385765163,-5.0183724341863));
#51199=CARTESIAN_POINT('Ctrl Pts',(-3.25592170098541,-1.38899996899466,
-5.023786692265));
#51200=CARTESIAN_POINT('Ctrl Pts',(-3.3316548770961,-1.21131062250045,-5.03030010222667));
#51201=CARTESIAN_POINT('Ctrl Pts',(-3.39291563048331,-1.0274545075206,-5.03681351218833));
#51202=CARTESIAN_POINT('Ctrl Pts',(-3.4388318118105,-0.839831766260492,
-5.04332692215));
#51203=CARTESIAN_POINT('Ctrl Pts',(-3.46293778073547,-0.741329934450789,
-5.04674645865311));
#51204=CARTESIAN_POINT('Ctrl Pts',(-3.48281390249413,-0.641787444045981,
-5.05016599515622));
#51205=CARTESIAN_POINT('Ctrl Pts',(-3.49832847032117,-0.541569860445466,
-5.05358553165932));
#51206=CARTESIAN_POINT('Ctrl Pts',(-3.51236549246657,-0.450896600574981,
-5.05667940511788));
#51207=CARTESIAN_POINT('Ctrl Pts',(-3.52283219794054,-0.359670757793759,
-5.05977327857645));
#51208=CARTESIAN_POINT('Ctrl Pts',(-3.52973959895587,-0.268179901742102,
-5.06286715203501));
#51209=CARTESIAN_POINT('Ctrl Pts',(-3.54428147831359,-0.0755678052264873,
-5.06938056199667));
#51210=CARTESIAN_POINT('Ctrl Pts',(-3.54305196908429,0.118222685023444,
-5.07589397195833));
#51211=CARTESIAN_POINT('Ctrl Pts',(-3.52615816121155,0.3106374510054,-5.08240738191999));
#51212=CARTESIAN_POINT('Ctrl Pts',(-3.51127051610728,0.480202700612879,
-5.08814731554883));
#51213=CARTESIAN_POINT('Ctrl Pts',(-3.48421326830643,0.648717483567016,
-5.09388724917767));
#51214=CARTESIAN_POINT('Ctrl Pts',(-3.44505320963117,0.814376069645967,
-5.0996271828065));
#51215=CARTESIAN_POINT('Ctrl Pts',(-3.43977625339156,0.836699149309945,
-5.10040065913933));
#51216=CARTESIAN_POINT('Ctrl Pts',(-3.4342795483969,0.85897036558526,-5.10117413547217));
#51217=CARTESIAN_POINT('Ctrl Pts',(-3.42856490437154,0.881185686590716,
-5.101947611805));
#51218=CARTESIAN_POINT('Ctrl Pts',(-3.38044213998663,1.06825992144005,-5.10846102176667));
#51219=CARTESIAN_POINT('Ctrl Pts',(-3.31687241555554,1.25134319073251,-5.11497443172833));
#51220=CARTESIAN_POINT('Ctrl Pts',(-3.23893637138191,1.42807546042492,-5.12148784169));
#51221=CARTESIAN_POINT('Ctrl Pts',(-3.16100032720827,1.60480773011733,-5.12800125165167));
#51222=CARTESIAN_POINT('Ctrl Pts',(-3.06868910928958,1.77521130597631,-5.13451466161333));
#51223=CARTESIAN_POINT('Ctrl Pts',(-2.96305546573071,1.93693229393157,-5.141028071575));
#51224=CARTESIAN_POINT('Ctrl Pts',(-2.93796716681119,1.97534150098615,-5.1425750254677));
#51225=CARTESIAN_POINT('Ctrl Pts',(-2.91212788447957,2.01326000353812,-5.14412197936041));
#51226=CARTESIAN_POINT('Ctrl Pts',(-2.88555239687917,2.05065535009337,-5.14566893325311));
#51227=CARTESIAN_POINT('Ctrl Pts',(-2.80023247086108,2.1707121576857,-5.15063538932208));
#51228=CARTESIAN_POINT('Ctrl Pts',(-2.70732368293247,2.28537607124037,-5.15560184539104));
#51229=CARTESIAN_POINT('Ctrl Pts',(-2.60768233598873,2.39383487273625,-5.16056830146001));
#51230=CARTESIAN_POINT('Ctrl Pts',(-2.47700465903675,2.53607646881263,-5.16708171142167));
#51231=CARTESIAN_POINT('Ctrl Pts',(-2.3347360735518,2.66766424466987,-5.17359512138333));
#51232=CARTESIAN_POINT('Ctrl Pts',(-2.18272371894347,2.78683825766546,-5.18010853134499));
#51233=CARTESIAN_POINT('Ctrl Pts',(-2.09246668450921,2.85759759181515,-5.1839758556076));
#51234=CARTESIAN_POINT('Ctrl Pts',(-1.99876997137404,2.92398232168098,-5.18784317987021));
#51235=CARTESIAN_POINT('Ctrl Pts',(-1.90204061354772,2.98560571817767,-5.19171050413282));
#51236=CARTESIAN_POINT('Ctrl Pts',(-1.83585682521188,3.02776944098037,-5.19435658983187));
#51237=CARTESIAN_POINT('Ctrl Pts',(-1.7682533936754,3.06770422962763,-5.19700267553092));
#51238=CARTESIAN_POINT('Ctrl Pts',(-1.69939760621079,3.10534408721984,-5.19964876122998));
#51239=CARTESIAN_POINT('Ctrl Pts',(-1.52990726349332,3.19799559260592,-5.20616217119167));
#51240=CARTESIAN_POINT('Ctrl Pts',(-1.35283221159455,3.27674344861159,-5.21267558115337));
#51241=CARTESIAN_POINT('Ctrl Pts',(-1.1705592811959,3.34065903690989,-5.21918899111507));
#51242=CARTESIAN_POINT('Ctrl Pts',(-0.997400068785245,3.40137882073238,
-5.22537672802482));
#51243=CARTESIAN_POINT('Ctrl Pts',(-0.819528440494076,3.44871677050005,
-5.23156446493458));
#51244=CARTESIAN_POINT('Ctrl Pts',(-0.639037774186981,3.4818430066795,-5.23775220184434));
#51245=CARTESIAN_POINT('Ctrl Pts',(-0.629538187021195,3.48358650718565,
-5.23807787489622));
#51246=CARTESIAN_POINT('Ctrl Pts',(-0.62003134595265,3.48529064171064,-5.23840354794811));
#51247=CARTESIAN_POINT('Ctrl Pts',(-0.61051757907874,3.48695541282214,-5.238729221));
#51248=CARTESIAN_POINT('Ctrl Pts',(-0.420243733667227,3.52025057396201,
-5.24524263096164));
#51249=CARTESIAN_POINT('Ctrl Pts',(-0.227230723008247,3.53779512210829,
-5.25175604092327));
#51250=CARTESIAN_POINT('Ctrl Pts',(-0.0340855960367684,3.53962915369353,
-5.2582694508849));
#51251=CARTESIAN_POINT('Ctrl Pts',(0.159059530937512,3.54146318527879,-5.26478286084663));
#51252=CARTESIAN_POINT('Ctrl Pts',(0.352360719567761,3.52758887010852,-5.27129627080837));
#51253=CARTESIAN_POINT('Ctrl Pts',(0.543247550769443,3.4980247813142,-5.27780968077025));
#51254=CARTESIAN_POINT('Ctrl Pts',(0.601707228720348,3.48897068837889,-5.2798044325629));
#51255=CARTESIAN_POINT('Ctrl Pts',(0.659939301890289,3.47844500445235,-5.28179918435557));
#51256=CARTESIAN_POINT('Ctrl Pts',(0.717867025561981,3.466448749601,-5.28379393614825));
#51257=CARTESIAN_POINT('Ctrl Pts',(0.849089156932971,3.43927395262494,-5.28831259431742));
#51258=CARTESIAN_POINT('Ctrl Pts',(0.978749296819402,3.40455233357054,-5.29283125248663));
#51259=CARTESIAN_POINT('Ctrl Pts',(1.10602473720318,3.36262936004284,-5.29734991065576));
#51260=CARTESIAN_POINT('Ctrl Pts',(1.28948564313355,3.30219958129296,-5.30386332061764));
#51261=CARTESIAN_POINT('Ctrl Pts',(1.46801104029239,3.22680554536042,-5.31037673057937));
#51262=CARTESIAN_POINT('Ctrl Pts',(1.63924880370262,3.13743299108219,-5.3168901405411));
#51263=CARTESIAN_POINT('Ctrl Pts',(1.75269332737295,3.07822393200914,-5.32120525582795));
#51264=CARTESIAN_POINT('Ctrl Pts',(1.86294511722153,3.01287435802278,-5.3255203711148));
#51265=CARTESIAN_POINT('Ctrl Pts',(1.96928647887088,2.941685021231,-5.32983548640166));
#51266=CARTESIAN_POINT('Ctrl Pts',(2.02346107989141,2.90541828684098,-5.33203378107644));
#51267=CARTESIAN_POINT('Ctrl Pts',(2.07662086897177,2.86763609085749,-5.33423207575122));
#51268=CARTESIAN_POINT('Ctrl Pts',(2.12869278492199,2.82841085585619,-5.336430370426));
#51269=CARTESIAN_POINT('Ctrl Pts',(2.28297862292286,2.71218893195501,-5.34294378038764));
#51270=CARTESIAN_POINT('Ctrl Pts',(2.42770829556085,2.58330600898348,-5.34945719034927));
#51271=CARTESIAN_POINT('Ctrl Pts',(2.56106883516398,2.44357975449348,-5.35597060031091));
#51272=CARTESIAN_POINT('Ctrl Pts',(2.69442937476905,2.30385350000145,-5.36248401027264));
#51273=CARTESIAN_POINT('Ctrl Pts',(2.81643557043219,2.1532649176556,-5.36899742023437));
#51274=CARTESIAN_POINT('Ctrl Pts',(2.92522794721502,1.99364991391056,-5.3755108301961));
#51275=CARTESIAN_POINT('Ctrl Pts',(2.92726781554804,1.99065711605796,-5.37563295730751));
#51276=CARTESIAN_POINT('Ctrl Pts',(2.92930303206135,1.98766115426643,-5.37575508441893));
#51277=CARTESIAN_POINT('Ctrl Pts',(2.9313335845635,1.984662040754,-5.37587721153035));
#51278=CARTESIAN_POINT('Ctrl Pts',(3.03759856727369,1.82770931719371,-5.38226849438057));
#51279=CARTESIAN_POINT('Ctrl Pts',(3.13108925869377,1.66212467796123,-5.38865977723078));
#51280=CARTESIAN_POINT('Ctrl Pts',(3.21084406279643,1.49018936490803,-5.395051060081));
#51281=CARTESIAN_POINT('Ctrl Pts',(3.29212285262701,1.31496864521171,-5.40156447004263));
#51282=CARTESIAN_POINT('Ctrl Pts',(3.35914855060852,1.13313177099434,-5.40807788000427));
#51283=CARTESIAN_POINT('Ctrl Pts',(3.41090884185987,0.947034149938319,-5.41459128996591));
#51284=CARTESIAN_POINT('Ctrl Pts',(3.43031907907144,0.877247081862021,-5.41703383480781));
#51285=CARTESIAN_POINT('Ctrl Pts',(3.4475820095095,0.806861453565564,-5.41947637964972));
#51286=CARTESIAN_POINT('Ctrl Pts',(3.46264250659767,0.736007385494901,-5.42191892449163));
#51287=CARTESIAN_POINT('Ctrl Pts',(3.48774307025223,0.617918517950802,-5.42598978961145));
#51288=CARTESIAN_POINT('Ctrl Pts',(3.50672549247776,0.498528446452136,-5.43006065473127));
#51289=CARTESIAN_POINT('Ctrl Pts',(3.51957889593106,0.378491351196591,-5.43413151985108));
#51290=CARTESIAN_POINT('Ctrl Pts',(3.54014442282263,0.186431238913331,-5.4406449298127));
#51291=CARTESIAN_POINT('Ctrl Pts',(3.54502560134987,-0.00730000610566984,
-5.4471583397743));
#51292=CARTESIAN_POINT('Ctrl Pts',(3.53418198158554,-0.200151998238902,
-5.45367174973592));
#51293=CARTESIAN_POINT('Ctrl Pts',(3.52625261802275,-0.341174423652751,
-5.45843466071414));
#51294=CARTESIAN_POINT('Ctrl Pts',(3.50991175822703,-0.481737410954006,
-5.46319757169237));
#51295=CARTESIAN_POINT('Ctrl Pts',(3.48514125710933,-0.620798210365567,
-5.46796048267059));
#51296=CARTESIAN_POINT('Ctrl Pts',(3.47603742602251,-0.671906826320724,
-5.46971098165409));
#51297=CARTESIAN_POINT('Ctrl Pts',(3.46579506342518,-0.722812536677146,
-5.4714614806376));
#51298=CARTESIAN_POINT('Ctrl Pts',(3.45443274215295,-0.7734670235766,-5.4732119796211));
#51299=CARTESIAN_POINT('Ctrl Pts',(3.41215482182319,-0.961946675768368,
-5.47972538958273));
#51300=CARTESIAN_POINT('Ctrl Pts',(3.35437640811406,-1.1469330851341,-5.48623879954437));
#51301=CARTESIAN_POINT('Ctrl Pts',(3.28203684521707,-1.32602898115537,-5.492752209506));
#51302=CARTESIAN_POINT('Ctrl Pts',(3.20969728232009,-1.50512487717664,-5.49926561946764));
#51303=CARTESIAN_POINT('Ctrl Pts',(3.12278631763227,-1.67835197646303,-5.50577902942927));
#51304=CARTESIAN_POINT('Ctrl Pts',(3.02223197295951,-1.8432806479056,-5.51229243939091));
#51305=CARTESIAN_POINT('Ctrl Pts',(3.01343337877785,-1.85771205267151,-5.512862368529));
#51306=CARTESIAN_POINT('Ctrl Pts',(3.00453044323614,-1.8720797233967,-5.5134322976671));
#51307=CARTESIAN_POINT('Ctrl Pts',(2.9955238080915,-1.8863820172901,-5.5140022268052));
#51308=CARTESIAN_POINT('Ctrl Pts',(2.90159851161271,-2.03553285694236,-5.51994570762883));
#51309=CARTESIAN_POINT('Ctrl Pts',(2.79639484911094,-2.17757303830368,-5.52588918845246));
#51310=CARTESIAN_POINT('Ctrl Pts',(2.68128796199762,-2.31104848987915,-5.53183266927608));
#51311=CARTESIAN_POINT('Ctrl Pts',(2.55514330578951,-2.45732309927445,-5.5383460792377));
#51312=CARTESIAN_POINT('Ctrl Pts',(2.41709243724114,-2.5933320851481,-5.5448594891993));
#51313=CARTESIAN_POINT('Ctrl Pts',(2.26888276917332,-2.71720685314313,-5.55137289916092));
#51314=CARTESIAN_POINT('Ctrl Pts',(2.20311454325284,-2.77217643666326,-5.55426323299307));
#51315=CARTESIAN_POINT('Ctrl Pts',(2.13534527838208,-2.82475626413618,-5.55715356682523));
#51316=CARTESIAN_POINT('Ctrl Pts',(2.06573588820082,-2.874775685197,-5.56004390065739));
#51317=CARTESIAN_POINT('Ctrl Pts',(1.97847948994207,-2.93747576795006,-5.56366697678695));
#51318=CARTESIAN_POINT('Ctrl Pts',(1.8883316623885,-2.99615253300867,-5.56729005291652));
#51319=CARTESIAN_POINT('Ctrl Pts',(1.79571220403399,-3.05061307565962,-5.57091312904609));
#51320=CARTESIAN_POINT('Ctrl Pts',(1.62920493752531,-3.14851988974053,-5.57742653900773));
#51321=CARTESIAN_POINT('Ctrl Pts',(1.45470238311938,-3.23280915686397,-5.58393994896937));
#51322=CARTESIAN_POINT('Ctrl Pts',(1.27452614193469,-3.30242008610374,-5.590453358931));
#51323=CARTESIAN_POINT('Ctrl Pts',(1.13038560964147,-3.3581086515221,-5.59566407024755));
#51324=CARTESIAN_POINT('Ctrl Pts',(0.982599582851888,-3.40440558395331,
-5.60087478156409));
#51325=CARTESIAN_POINT('Ctrl Pts',(0.832403080383234,-3.440741942048,-5.60608549288073));
#51326=CARTESIAN_POINT('Ctrl Pts',(0.794853354755285,-3.44982617672956,
-5.60738819152584));
#51327=CARTESIAN_POINT('Ctrl Pts',(0.757152994147706,-3.45828791657968,
-5.60869089017095));
#51328=CARTESIAN_POINT('Ctrl Pts',(0.719323216056949,-3.46612616198879,
-5.60999358881607));
#51329=CARTESIAN_POINT('Ctrl Pts',(0.53017674354351,-3.50531688804249,-5.61650699877797));
#51330=CARTESIAN_POINT('Ctrl Pts',(0.337816928320247,-3.52891744226118,
-5.62302040874003));
#51331=CARTESIAN_POINT('Ctrl Pts',(0.14482526557731,-3.53682450849307,-5.62953381870193));
#51332=CARTESIAN_POINT('Ctrl Pts',(-0.0481663971628286,-3.54473157472486,
-5.63604722866373));
#51333=CARTESIAN_POINT('Ctrl Pts',(-0.241813887038626,-3.53694580387158,
-5.64256063862537));
#51334=CARTESIAN_POINT('Ctrl Pts',(-0.43353044931056,-3.51334032191244,
-5.649074048587));
#51335=CARTESIAN_POINT('Ctrl Pts',(-0.463486537026694,-3.50965191920081,
-5.6500917816291));
#51336=CARTESIAN_POINT('Ctrl Pts',(-0.493394854987646,-3.50557733750051,
-5.6511095146712));
#51337=CARTESIAN_POINT('Ctrl Pts',(-0.523245315398818,-3.50111615630133,
-5.6521272477133));
#51338=CARTESIAN_POINT('Ctrl Pts',(-0.684435410967259,-3.4770261351111,
-5.65762292463283));
#51339=CARTESIAN_POINT('Ctrl Pts',(-0.843938087347245,-3.44166213854163,
-5.66311860155237));
#51340=CARTESIAN_POINT('Ctrl Pts',(-1.00025566879186,-3.3955592316282,-5.6686142784719));
#51341=CARTESIAN_POINT('Ctrl Pts',(-1.1855213798375,-3.34091862273666,-5.67512768843364));
#51342=CARTESIAN_POINT('Ctrl Pts',(-1.36633644531484,-3.27119098514052,
-5.68164109839537));
#51343=CARTESIAN_POINT('Ctrl Pts',(-1.54029195487117,-3.18722583254679,
-5.68815450835708));
#51344=CARTESIAN_POINT('Ctrl Pts',(-1.62944410370729,-3.14419371588561,
-5.69149262909737));
#51345=CARTESIAN_POINT('Ctrl Pts',(-1.71679583817648,-3.09742028661071,
-5.69483074983765));
#51346=CARTESIAN_POINT('Ctrl Pts',(-1.80200661175621,-3.04702677559416,
-5.69816887057794));
#51347=CARTESIAN_POINT('Ctrl Pts',(-1.88306085512837,-2.99909142968991,
-5.70134415979926));
#51348=CARTESIAN_POINT('Ctrl Pts',(-1.96217788986923,-2.94788060262952,
-5.70451944902059));
#51349=CARTESIAN_POINT('Ctrl Pts',(-2.03912504838554,-2.89360083987272,
-5.70769473824192));
#51350=CARTESIAN_POINT('Ctrl Pts',(-2.19696528084022,-2.78225780217885,
-5.71420814820364));
#51351=CARTESIAN_POINT('Ctrl Pts',(-2.34568157844476,-2.65800144637074,
-5.72072155816537));
#51352=CARTESIAN_POINT('Ctrl Pts',(-2.48336853770674,-2.52253489439242,
-5.7272349681271));
#51353=CARTESIAN_POINT('Ctrl Pts',(-2.60298386808918,-2.4048485393628,-5.73289348283804));
#51354=CARTESIAN_POINT('Ctrl Pts',(-2.71428549057575,-2.27868697184984,
-5.73855199754897));
#51355=CARTESIAN_POINT('Ctrl Pts',(-2.81597612222633,-2.14519893694035,
-5.74421051225991));
#51356=CARTESIAN_POINT('Ctrl Pts',(-2.83133966592628,-2.12503140307353,
-5.74506540751061));
#51357=CARTESIAN_POINT('Ctrl Pts',(-2.84648385104755,-2.10469665766999,
-5.7459203027613));
#51358=CARTESIAN_POINT('Ctrl Pts',(-2.86140601976011,-2.08420004970933,
-5.746775198012));
#51359=CARTESIAN_POINT('Ctrl Pts',(-2.97509737816046,-1.92803727963656,
-5.75328860797363));
#51360=CARTESIAN_POINT('Ctrl Pts',(-3.07588539103572,-1.76250130618686,
-5.75980201793527));
#51361=CARTESIAN_POINT('Ctrl Pts',(-3.16263326328894,-1.58992343651983,
-5.76631542789691));
#51362=CARTESIAN_POINT('Ctrl Pts',(-3.24938113554341,-1.4173455668503,-5.77282883785864));
#51363=CARTESIAN_POINT('Ctrl Pts',(-3.32210027300758,-1.23770469083994,
-5.77934224782037));
#51364=CARTESIAN_POINT('Ctrl Pts',(-3.37963916765126,-1.05330980373386,
-5.7858556577821));
#51365=CARTESIAN_POINT('Ctrl Pts',(-3.39258558113939,-1.01182043435414,
-5.78732119338379));
#51366=CARTESIAN_POINT('Ctrl Pts',(-3.40476309979245,-0.970091329658437,
-5.78878672898548));
#51367=CARTESIAN_POINT('Ctrl Pts',(-3.41615839043217,-0.928149692388579,
-5.79025226458717));
#51368=CARTESIAN_POINT('Ctrl Pts',(-3.45540820147598,-0.783686388225696,
-5.79530013894711));
#51369=CARTESIAN_POINT('Ctrl Pts',(-3.48537682874472,-0.636701514870851,
-5.80034801330706));
#51370=CARTESIAN_POINT('Ctrl Pts',(-3.50597617628425,-0.488430196162447,
-5.805395887667));
#51371=CARTESIAN_POINT('Ctrl Pts',(-3.53255607623814,-0.297111669702389,
-5.81190929762864));
#51372=CARTESIAN_POINT('Ctrl Pts',(-3.54354418974018,-0.103630424635091,
-5.81842270759027));
#51373=CARTESIAN_POINT('Ctrl Pts',(-3.53875253925765,0.089468803271073,
-5.82493611755191));
#51374=CARTESIAN_POINT('Ctrl Pts',(-3.53596740081211,0.201707391082333,
-5.82872202567726));
#51375=CARTESIAN_POINT('Ctrl Pts',(-3.52784953284791,0.313821101074286,
-5.83250793380262));
#51376=CARTESIAN_POINT('Ctrl Pts',(-3.51436099043,0.425284409474744,-5.83629384192797));
#51377=CARTESIAN_POINT('Ctrl Pts',(-3.50464336839674,0.505586510921572,
-5.83902134376434));
#51378=CARTESIAN_POINT('Ctrl Pts',(-3.49213834393737,0.585551019147991,
-5.84174884560071));
#51379=CARTESIAN_POINT('Ctrl Pts',(-3.47690638446997,0.66499043379555,-5.84447634743708));
#51380=CARTESIAN_POINT('Ctrl Pts',(-3.44053170812434,0.854695704681691,
-5.8509897573987));
#51381=CARTESIAN_POINT('Ctrl Pts',(-3.38860921956519,1.04140602837934,-5.8575031673603));
#51382=CARTESIAN_POINT('Ctrl Pts',(-3.32193574191479,1.22268842298407,-5.86401657732192));
#51383=CARTESIAN_POINT('Ctrl Pts',(-3.25942939273935,1.3926405697123,-5.87012289563216));
#51384=CARTESIAN_POINT('Ctrl Pts',(-3.18394820657006,1.55784068731747,-5.87622921394241));
#51385=CARTESIAN_POINT('Ctrl Pts',(-3.09615376327333,1.71622605567233,-5.88233553225266));
#51386=CARTESIAN_POINT('Ctrl Pts',(-3.09030074626759,1.7267851778631,-5.88274262390414));
#51387=CARTESIAN_POINT('Ctrl Pts',(-3.08439300690686,1.73731401277661,-5.88314971555562));
#51388=CARTESIAN_POINT('Ctrl Pts',(-3.0784309562568,1.74781206796055,-5.8835568072071));
#51389=CARTESIAN_POINT('Ctrl Pts',(-2.98303897276905,1.91577949486414,-5.89007021716873));
#51390=CARTESIAN_POINT('Ctrl Pts',(-2.87375899624301,2.0758403789111,-5.89658362713037));
#51391=CARTESIAN_POINT('Ctrl Pts',(-2.75227553257105,2.22600746165049,-5.903097037092));
#51392=CARTESIAN_POINT('Ctrl Pts',(-2.63079206889909,2.37617454438987,-5.90961044705364));
#51393=CARTESIAN_POINT('Ctrl Pts',(-2.49709140537515,2.51646756267748,-5.91612385701527));
#51394=CARTESIAN_POINT('Ctrl Pts',(-2.35282015491859,2.64491088381421,-5.92263726697691));
#51395=CARTESIAN_POINT('Ctrl Pts',(-2.31044002818164,2.6826415072826,-5.92455060133001));
#51396=CARTESIAN_POINT('Ctrl Pts',(-2.26714849820321,2.71934870346318,-5.92646393568311));
#51397=CARTESIAN_POINT('Ctrl Pts',(-2.222989224079,2.754980745782,-5.92837727003622));
#51398=CARTESIAN_POINT('Ctrl Pts',(-2.11682063965784,2.84064799389807,-5.93297734564484));
#51399=CARTESIAN_POINT('Ctrl Pts',(-2.00563588372431,2.92009993133965,-5.93757742125347));
#51400=CARTESIAN_POINT('Ctrl Pts',(-1.89026706688281,2.99289754536391,-5.94217749686209));
#51401=CARTESIAN_POINT('Ctrl Pts',(-1.72691227343801,3.09597426512039,-5.94869090682373));
#51402=CARTESIAN_POINT('Ctrl Pts',(-1.55515506607057,3.18572418961666,-5.95520431678537));
#51403=CARTESIAN_POINT('Ctrl Pts',(-1.37724999191978,3.26095501036923,-5.96171772674717));
#51404=CARTESIAN_POINT('Ctrl Pts',(-1.26161218703417,3.30985483525111,-5.96595142516132));
#51405=CARTESIAN_POINT('Ctrl Pts',(-1.14336967917687,3.3526213717884,-5.97018512357555));
#51406=CARTESIAN_POINT('Ctrl Pts',(-1.02317256118378,3.3889110212635,-5.97441882198976));
#51407=CARTESIAN_POINT('Ctrl Pts',(-0.958450247245205,3.40845183992259,
-5.97669853353743));
#51408=CARTESIAN_POINT('Ctrl Pts',(-0.893161262302633,3.42611482909649,
-5.9789782450851));
#51409=CARTESIAN_POINT('Ctrl Pts',(-0.827419800164966,3.44188829366148,
-5.98125795663274));
#51410=CARTESIAN_POINT('Ctrl Pts',(-0.639588539302325,3.48695497823278,
-5.98777136659464));
#51411=CARTESIAN_POINT('Ctrl Pts',(-0.448071840368233,3.51659792381026,
-5.99428477655636));
#51412=CARTESIAN_POINT('Ctrl Pts',(-0.255423787888959,3.53056979807232,
-6.00079818651808));
#51413=CARTESIAN_POINT('Ctrl Pts',(-0.0627757354124814,3.54454167233417,
-6.0073115964797));
#51414=CARTESIAN_POINT('Ctrl Pts',(0.131027743644201,3.54284160663297,-6.0138250064413));
#51415=CARTESIAN_POINT('Ctrl Pts',(0.323385332326878,3.52519811655209,-6.02033841640292));
#51416=CARTESIAN_POINT('Ctrl Pts',(0.515742921012345,3.50755462647095,-6.02685182636464));
#51417=CARTESIAN_POINT('Ctrl Pts',(0.706621482692652,3.47396442994213,-6.03336523632637));
#51418=CARTESIAN_POINT('Ctrl Pts',(0.893511611909647,3.42517311385951,-6.03987864628809));
#51419=CARTESIAN_POINT('Ctrl Pts',(1.08040174112393,3.3763817977776,-6.04639205624973));
#51420=CARTESIAN_POINT('Ctrl Pts',(1.26332731289825,3.31238606054051,-6.05290546621136));
#51421=CARTESIAN_POINT('Ctrl Pts',(1.43982452056484,3.23389875855054,-6.059418876173));
#51422=CARTESIAN_POINT('Ctrl Pts',(1.50380522324394,3.20544690484081,-6.06178000444065));
#51423=CARTESIAN_POINT('Ctrl Pts',(1.56694025449916,3.17509076695823,-6.0641411327083));
#51424=CARTESIAN_POINT('Ctrl Pts',(1.62910723813456,3.14286646338266,-6.06650226097594));
#51425=CARTESIAN_POINT('Ctrl Pts',(1.73843413564225,3.08619678233581,-6.07065454266993));
#51426=CARTESIAN_POINT('Ctrl Pts',(1.84476690245898,3.02374911182526,-6.07480682436392));
#51427=CARTESIAN_POINT('Ctrl Pts',(1.94756203567169,2.95595504167199,-6.07895910605791));
#51428=CARTESIAN_POINT('Ctrl Pts',(2.10880996970625,2.84961096281966,-6.08547251601964));
#51429=CARTESIAN_POINT('Ctrl Pts',(2.26136901605629,2.73010640649609,-6.09198592598137));
#51430=CARTESIAN_POINT('Ctrl Pts',(2.40324259782627,2.59902847899996,-6.09849933594308));
#51431=CARTESIAN_POINT('Ctrl Pts',(2.50521379478413,2.50481662507491,-6.10318082915547));
#51432=CARTESIAN_POINT('Ctrl Pts',(2.60167081814559,2.40461726441304,-6.10786232236785));
#51433=CARTESIAN_POINT('Ctrl Pts',(2.69183711822383,2.2990460910885,-6.11254381558023));
#51434=CARTESIAN_POINT('Ctrl Pts',(2.72712012469975,2.25773499826505,-6.11437573232946));
#51435=CARTESIAN_POINT('Ctrl Pts',(2.76143995124405,2.2156014429839,-6.11620764907869));
#51436=CARTESIAN_POINT('Ctrl Pts',(2.79476729971627,2.17269706292566,-6.11803956582792));
#51437=CARTESIAN_POINT('Ctrl Pts',(2.91326323225658,2.02014983795509,-6.12455297578964));
#51438=CARTESIAN_POINT('Ctrl Pts',(3.01920517514468,1.85787088053258,-6.13106638575137));
#51439=CARTESIAN_POINT('Ctrl Pts',(3.11133748932251,1.68810632525813,-6.1375797957131));
#51440=CARTESIAN_POINT('Ctrl Pts',(3.203469803499,1.51834176998613,-6.14409320567473));
#51441=CARTESIAN_POINT('Ctrl Pts',(3.28180255010409,1.34106980168587,-6.15060661563637));
#51442=CARTESIAN_POINT('Ctrl Pts',(3.34504642056238,1.15855163970423,-6.157120025598));
#51443=CARTESIAN_POINT('Ctrl Pts',(3.34978975557038,1.14486264848577,-6.15760853595116));
#51444=CARTESIAN_POINT('Ctrl Pts',(3.35444815655005,1.1311443095087,-6.15809704630431));
#51445=CARTESIAN_POINT('Ctrl Pts',(3.35902108122167,1.11739759079248,-6.15858555665747));
#51446=CARTESIAN_POINT('Ctrl Pts',(3.41541991061322,0.94785645481421,-6.16461045626595));
#51447=CARTESIAN_POINT('Ctrl Pts',(3.45881608303693,0.773998449359656,-6.17063535587443));
#51448=CARTESIAN_POINT('Ctrl Pts',(3.48894891305953,0.597889911087293,-6.17666025548291));
#51449=CARTESIAN_POINT('Ctrl Pts',(3.52152497042123,0.407502156590185,-6.18317366544464));
#51450=CARTESIAN_POINT('Ctrl Pts',(3.53860724556339,0.214461276056274,-6.18968707540637));
#51451=CARTESIAN_POINT('Ctrl Pts',(3.53986050381078,0.021304435887652,-6.1962004853681));
#51452=CARTESIAN_POINT('Ctrl Pts',(3.54040097332149,-0.061994742963288,
-6.19900940324467));
#51453=CARTESIAN_POINT('Ctrl Pts',(3.53799699077534,-0.145315513407627,
-6.20181832112124));
#51454=CARTESIAN_POINT('Ctrl Pts',(3.53262128868333,-0.22844437121557,-6.20462723899781));
#51455=CARTESIAN_POINT('Ctrl Pts',(3.5255316382462,-0.338077407609597,-6.20833173108287));
#51456=CARTESIAN_POINT('Ctrl Pts',(3.51327303496331,-0.447376576378206,
-6.21203622316794));
#51457=CARTESIAN_POINT('Ctrl Pts',(3.49597098000898,-0.555864346356779,
-6.215740715253));
#51458=CARTESIAN_POINT('Ctrl Pts',(3.46554970375613,-0.746612579979145,
-6.22225412521464));
#51459=CARTESIAN_POINT('Ctrl Pts',(3.41953925747835,-0.934864572484402,
-6.22876753517627));
#51460=CARTESIAN_POINT('Ctrl Pts',(3.35859301744289,-1.11815333279855,-6.23528094513791));
#51461=CARTESIAN_POINT('Ctrl Pts',(3.31059801777636,-1.2624927372481,-6.24041023791716));
#51462=CARTESIAN_POINT('Ctrl Pts',(3.25333356013243,-1.40376624524555,-6.24553953069642));
#51463=CARTESIAN_POINT('Ctrl Pts',(3.18712845076366,-1.54071809177819,-6.25066882347567));
#51464=CARTESIAN_POINT('Ctrl Pts',(3.16926329207835,-1.57767394751018,-6.25205294065814));
#51465=CARTESIAN_POINT('Ctrl Pts',(3.15074717578934,-1.61431513677177,-6.25343705784061));
#51466=CARTESIAN_POINT('Ctrl Pts',(3.13159534362019,-1.65062121645643,-6.25482117502308));
#51467=CARTESIAN_POINT('Ctrl Pts',(3.04147021836802,-1.82147118788974,-6.2613345849847));
#51468=CARTESIAN_POINT('Ctrl Pts',(2.93727842881738,-1.98488223342344,-6.2678479949463));
#51469=CARTESIAN_POINT('Ctrl Pts',(2.82057762917812,-2.13879529781198,-6.27436140490792));
#51470=CARTESIAN_POINT('Ctrl Pts',(2.70387682953718,-2.29270836220275,-6.28087481486964));
#51471=CARTESIAN_POINT('Ctrl Pts',(2.57465211340251,-2.43714224335224,-6.28738822483137));
#51472=CARTESIAN_POINT('Ctrl Pts',(2.43444850641693,-2.57001604546182,-6.29390163479326));
#51473=CARTESIAN_POINT('Ctrl Pts',(2.41429399083976,-2.58911688867116,-6.2948379489535));
#51474=CARTESIAN_POINT('Ctrl Pts',(2.39391298941519,-2.60797845638822,-6.29577426311375));
#51475=CARTESIAN_POINT('Ctrl Pts',(2.37331023111434,-2.62659447705366,-6.296710577274));
#51476=CARTESIAN_POINT('Ctrl Pts',(2.25059121040597,-2.73747962127514,-6.30228767307559));
#51477=CARTESIAN_POINT('Ctrl Pts',(2.12000384287054,-2.839652015463,-6.30786476887727));
#51478=CARTESIAN_POINT('Ctrl Pts',(1.98297254939446,-2.93225806317012,-6.31344186467883));
#51479=CARTESIAN_POINT('Ctrl Pts',(1.82293567289756,-3.04041133417721,-6.31995527464063));
#51480=CARTESIAN_POINT('Ctrl Pts',(1.65409266030275,-3.13553304456699,-6.32646868460227));
#51481=CARTESIAN_POINT('Ctrl Pts',(1.47862930850234,-3.2163003073892,-6.33298209456391));
#51482=CARTESIAN_POINT('Ctrl Pts',(1.390897632601,-3.25668393880083,-6.33623879954477));
#51483=CARTESIAN_POINT('Ctrl Pts',(1.30150905535828,-3.29347875878619,-6.33949550452563));
#51484=CARTESIAN_POINT('Ctrl Pts',(1.21075130737302,-3.32651187758184,-6.34275220950649));
#51485=CARTESIAN_POINT('Ctrl Pts',(1.1199935593875,-3.35954499637758,-6.34600891448736));
#51486=CARTESIAN_POINT('Ctrl Pts',(1.02786668212491,-3.3888163988914,-6.34926561946823));
#51487=CARTESIAN_POINT('Ctrl Pts',(0.934702221409373,-3.414273576702,-6.3525223244491));
#51488=CARTESIAN_POINT('Ctrl Pts',(0.748373299981275,-3.46518793232237,
-6.35903573441073));
#51489=CARTESIAN_POINT('Ctrl Pts',(0.557888991572958,-3.50085067113629,
-6.36554914437237));
#51490=CARTESIAN_POINT('Ctrl Pts',(0.365774049088018,-3.52087018018125,
-6.372062554334));
#51491=CARTESIAN_POINT('Ctrl Pts',(0.20127596813921,-3.53801184952169,-6.37763965013542));
#51492=CARTESIAN_POINT('Ctrl Pts',(0.0355650918612497,-3.54368319654726,
-6.38321674593683));
#51493=CARTESIAN_POINT('Ctrl Pts',(-0.1297187288212,-3.53762251397617,-6.38879384173825));
#51494=CARTESIAN_POINT('Ctrl Pts',(-0.157467504755981,-3.53660501255357,
-6.38973015589847));
#51495=CARTESIAN_POINT('Ctrl Pts',(-0.185204239670332,-3.53525686860412,
-6.39066647005869));
#51496=CARTESIAN_POINT('Ctrl Pts',(-0.212921279681585,-3.53357984669696,
-6.39160278421891));
#51497=CARTESIAN_POINT('Ctrl Pts',(-0.405733107366116,-3.52191375035853,
-6.39811619418064));
#51498=CARTESIAN_POINT('Ctrl Pts',(-0.597565292296506,-3.49433502470254,
-6.40462960414237));
#51499=CARTESIAN_POINT('Ctrl Pts',(-0.785896702128393,-3.45144460505232,
-6.41114301410408));
#51500=CARTESIAN_POINT('Ctrl Pts',(-0.97422811195755,-3.40855418540273,
-6.4176564240657));
#51501=CARTESIAN_POINT('Ctrl Pts',(-1.15908224871662,-3.35034725338159,
-6.4241698340273));
#51502=CARTESIAN_POINT('Ctrl Pts',(-1.33794234485403,-3.27739989599169,
-6.43068324398892));
#51503=CARTESIAN_POINT('Ctrl Pts',(-1.37595059764031,-3.26189838581898,
-6.43206736117139));
#51504=CARTESIAN_POINT('Ctrl Pts',(-1.41368726809313,-3.24573153652599,
-6.43345147835386));
#51505=CARTESIAN_POINT('Ctrl Pts',(-1.4511275397993,-3.22890521124983,-6.43483559553633));
#51506=CARTESIAN_POINT('Ctrl Pts',(-1.58987454601214,-3.16654983423889,
-6.43996488831558));
#51507=CARTESIAN_POINT('Ctrl Pts',(-1.72455052609608,-3.09513693232657,
-6.44509418109484));
#51508=CARTESIAN_POINT('Ctrl Pts',(-1.85409640965779,-3.01541712473751,
-6.45022347387409));
#51509=CARTESIAN_POINT('Ctrl Pts',(-2.01859968229062,-2.91418527636456,
-6.45673688383573));
#51510=CARTESIAN_POINT('Ctrl Pts',(-2.17485177726832,-2.79955082838338,
-6.46325029379736));
#51511=CARTESIAN_POINT('Ctrl Pts',(-2.32076642803647,-2.67298362342837,
-6.469763703759));
#51512=CARTESIAN_POINT('Ctrl Pts',(-2.40375516543355,-2.60099871663665,
-6.47346819584406));
#51513=CARTESIAN_POINT('Ctrl Pts',(-2.48340195179236,-2.52515037406617,
-6.47717268792913));
#51514=CARTESIAN_POINT('Ctrl Pts',(-2.55930369651983,-2.44572373521217,
-6.48087718001419));
#51515=CARTESIAN_POINT('Ctrl Pts',(-2.61685592304164,-2.38549877032363,
-6.48368609789077));
#51516=CARTESIAN_POINT('Ctrl Pts',(-2.67225503938364,-2.32321660732287,
-6.48649501576734));
#51517=CARTESIAN_POINT('Ctrl Pts',(-2.72538469578074,-2.25905832714279,
-6.48930393364391));
#51518=CARTESIAN_POINT('Ctrl Pts',(-2.84858346785115,-2.11028602420789,
-6.49581734360564));
#51519=CARTESIAN_POINT('Ctrl Pts',(-2.95958197207277,-1.95142785557342,
-6.50233075356736));
#51520=CARTESIAN_POINT('Ctrl Pts',(-3.05700615397888,-1.7846428881584,-6.50884416352909));
#51521=CARTESIAN_POINT('Ctrl Pts',(-3.14712345334602,-1.63036691124576,
-6.51486906313757));
#51522=CARTESIAN_POINT('Ctrl Pts',(-3.22563382835918,-1.46928943033375,
-6.52089396274604));
#51523=CARTESIAN_POINT('Ctrl Pts',(-3.29140876004433,-1.30316091650401,
-6.52691886235452));
#51524=CARTESIAN_POINT('Ctrl Pts',(-3.29674191697551,-1.28969089970129,
-6.52740737270768));
#51525=CARTESIAN_POINT('Ctrl Pts',(-3.3019913531112,-1.2761876799283,-6.52789588306084));
#51526=CARTESIAN_POINT('Ctrl Pts',(-3.30715686163083,-1.26265234730166,
-6.528384393414));
#51527=CARTESIAN_POINT('Ctrl Pts',(-3.37602965916945,-1.08218294722828,
-6.53489780337563));
#51528=CARTESIAN_POINT('Ctrl Pts',(-3.42997151868652,-0.89603342204106,
-6.54141121333727));
#51529=CARTESIAN_POINT('Ctrl Pts',(-3.46851662407281,-0.706764717832116,
-6.54792462329891));
#51530=CARTESIAN_POINT('Ctrl Pts',(-3.50706172945967,-0.517496013620438,
-6.55443803326064));
#51531=CARTESIAN_POINT('Ctrl Pts',(-3.53021639596121,-0.32508495181709,
-6.56095144322237));
#51532=CARTESIAN_POINT('Ctrl Pts',(-3.53749871140976,-0.132059280579998,
-6.56746485318408));
#51533=CARTESIAN_POINT('Ctrl Pts',(-3.53954688521147,-0.0777702119891359,
-6.56929676993332));
#51534=CARTESIAN_POINT('Ctrl Pts',(-3.5403393000852,-0.0234336768277606,
-6.57112868668255));
#51535=CARTESIAN_POINT('Ctrl Pts',(-3.53986520764733,0.0308919356641561,
-6.57296060343179));
#51536=CARTESIAN_POINT('Ctrl Pts',(-3.53865365666892,0.169721926844386,
-6.57764209664417));
#51537=CARTESIAN_POINT('Ctrl Pts',(-3.52917019745509,0.308480469767332,
-6.58232358985654));
#51538=CARTESIAN_POINT('Ctrl Pts',(-3.51161394105595,0.446196758891985,
-6.58700508306892));
#51539=CARTESIAN_POINT('Ctrl Pts',(-3.48718773981356,0.637802857369744,
-6.59351849303064));
#51540=CARTESIAN_POINT('Ctrl Pts',(-3.4471367782153,0.827411723408665,-6.60003190299237));
#51541=CARTESIAN_POINT('Ctrl Pts',(-3.39197035063338,1.01252418815714,-6.6065453129541));
#51542=CARTESIAN_POINT('Ctrl Pts',(-3.35680189836082,1.13053289683955,-6.61069759464808));
#51543=CARTESIAN_POINT('Ctrl Pts',(-3.31548686207736,1.24671997283311,-6.61484987634206));
#51544=CARTESIAN_POINT('Ctrl Pts',(-3.26816416858,1.3604054422155,-6.61900215803608));
#51545=CARTESIAN_POINT('Ctrl Pts',(-3.2412548792897,1.42505085771546,-6.62136328630376));
#51546=CARTESIAN_POINT('Ctrl Pts',(-3.21240318873926,1.48888742428309,-6.62372441457145));
#51547=CARTESIAN_POINT('Ctrl Pts',(-3.1816796260222,1.55180881165512,-6.62608554283917));
#51548=CARTESIAN_POINT('Ctrl Pts',(-3.0969255861,1.72538379143208,-6.63259895280097));
#51549=CARTESIAN_POINT('Ctrl Pts',(-2.9979321353066,1.89198966135704,-6.63911236276294));
#51550=CARTESIAN_POINT('Ctrl Pts',(-2.88612844378586,2.04949663734564,-6.64562577272474));
#51551=CARTESIAN_POINT('Ctrl Pts',(-2.7743247522635,2.20700361333651,-6.65213918268664));
#51552=CARTESIAN_POINT('Ctrl Pts',(-2.64969465291328,2.3554295711336,-6.65865259264837));
#51553=CARTESIAN_POINT('Ctrl Pts',(-2.51368120782473,2.4925903433037,-6.66516600261008));
#51554=CARTESIAN_POINT('Ctrl Pts',(-2.37766776273814,2.62975111547182,-6.6716794125717));
#51555=CARTESIAN_POINT('Ctrl Pts',(-2.23029846571805,2.75562791640694,-6.6781928225333));
#51556=CARTESIAN_POINT('Ctrl Pts',(-2.07374054798118,2.86875662093084,-6.68470623249492));
#51557=CARTESIAN_POINT('Ctrl Pts',(-1.91718263024204,2.98188532545637,-6.69121964245664));
#51558=CARTESIAN_POINT('Ctrl Pts',(-1.75141820912731,3.08228207284204,-6.69773305241837));
#51559=CARTESIAN_POINT('Ctrl Pts',(-1.57856280904735,3.16849459675079,-6.7042464623801));
#51560=CARTESIAN_POINT('Ctrl Pts',(-1.51806293971028,3.19866921917673,-6.70652617392767));
#51561=CARTESIAN_POINT('Ctrl Pts',(-1.45669512500734,3.22710553504123,-6.70880588547525));
#51562=CARTESIAN_POINT('Ctrl Pts',(-1.39455435995192,3.25373910096334,-6.71108559702283));
#51563=CARTESIAN_POINT('Ctrl Pts',(-1.27915148859172,3.30320083480635,-6.71531929543689));
#51564=CARTESIAN_POINT('Ctrl Pts',(-1.16108267271159,3.34644458612958,-6.71955299385094));
#51565=CARTESIAN_POINT('Ctrl Pts',(-1.04106677331439,3.38331569520124,-6.723786692265));
#51566=CARTESIAN_POINT('Ctrl Pts',(-0.85642614041225,3.44004072037697,-6.73030010222663));
#51567=CARTESIAN_POINT('Ctrl Pts',(-0.667162346706339,3.48169169421644,
-6.73681351218827));
#51568=CARTESIAN_POINT('Ctrl Pts',(-0.475768876624546,3.5077327830413,-6.74332692214991));
#51569=CARTESIAN_POINT('Ctrl Pts',(-0.340597831264551,3.5261242213556,-6.74792699775853));
#51570=CARTESIAN_POINT('Ctrl Pts',(-0.20435464586928,3.53672868968354,-6.75252707336715));
#51571=CARTESIAN_POINT('Ctrl Pts',(-0.0679589460948703,3.53934762091083,
-6.75712714897577));
#51572=CARTESIAN_POINT('Ctrl Pts',(-0.0112271442293234,3.54043692715533,
-6.75904048332888));
#51573=CARTESIAN_POINT('Ctrl Pts',(0.045531022636134,3.54014484257323,-6.76095381768199));
#51574=CARTESIAN_POINT('Ctrl Pts',(0.102248860493041,3.53848292849331,-6.76286715203509));
#51575=CARTESIAN_POINT('Ctrl Pts',(0.295328825580806,3.53282540830823,-6.76938056199673));
#51576=CARTESIAN_POINT('Ctrl Pts',(0.487928089795474,3.51129585116066,-6.77589397195837));
#51577=CARTESIAN_POINT('Ctrl Pts',(0.677515362239867,3.47434925711893,-6.78240738192));
#51578=CARTESIAN_POINT('Ctrl Pts',(0.867102634684259,3.43740266307719,-6.78892079188164));
#51579=CARTESIAN_POINT('Ctrl Pts',(1.053701106507,3.38503272719013,-6.79543420184327));
#51580=CARTESIAN_POINT('Ctrl Pts',(1.23474298622044,3.31767899823506,-6.80194761180491));
#51581=CARTESIAN_POINT('Ctrl Pts',(1.24605820178868,3.31346935368399,-6.80235470345639));
#51582=CARTESIAN_POINT('Ctrl Pts',(1.25735159732433,3.30920121986826,-6.80276179510787));
#51583=CARTESIAN_POINT('Ctrl Pts',(1.26862254139057,3.30487470980033,-6.80316888675936));
#51584=CARTESIAN_POINT('Ctrl Pts',(1.43768513914876,3.2399776588513,-6.8092752050696));
#51585=CARTESIAN_POINT('Ctrl Pts',(1.60169567108907,3.16194539799143,-6.81538152337985));
#51586=CARTESIAN_POINT('Ctrl Pts',(1.75882144669102,3.07193280717094,-6.82148784169008));
#51587=CARTESIAN_POINT('Ctrl Pts',(1.92642237085479,2.97591932147712,-6.8280012516517));
#51588=CARTESIAN_POINT('Ctrl Pts',(2.08621238736183,2.86626604784555,-6.8345146616133));
#51589=CARTESIAN_POINT('Ctrl Pts',(2.23601720366442,2.74432457051421,-6.84102807157492));
#51590=CARTESIAN_POINT('Ctrl Pts',(2.29874823302859,2.6932613631756,-6.8437555734113));
#51591=CARTESIAN_POINT('Ctrl Pts',(2.3597278326295,2.64004307078317,-6.84648307524768));
#51592=CARTESIAN_POINT('Ctrl Pts',(2.41878915883033,2.5847744592375,-6.84921057708405));
#51593=CARTESIAN_POINT('Ctrl Pts',(2.50076921536961,2.50805887916477,-6.8529964852094));
#51594=CARTESIAN_POINT('Ctrl Pts',(2.57905316667217,2.42739285957258,-6.85678239333475));
#51595=CARTESIAN_POINT('Ctrl Pts',(2.65333228007531,2.34320336556039,-6.86056830146009));
#51596=CARTESIAN_POINT('Ctrl Pts',(2.78112468843889,2.19836078861232,-6.86708171142173));
#51597=CARTESIAN_POINT('Ctrl Pts',(2.89707465218622,2.04308253276765,-6.87359512138337));
#51598=CARTESIAN_POINT('Ctrl Pts',(2.9996904458398,1.87943880835007,-6.880108531345));
#51599=CARTESIAN_POINT('Ctrl Pts',(3.07921739666291,1.75261538321336,-6.88515640570495));
#51600=CARTESIAN_POINT('Ctrl Pts',(3.15074015167961,1.62075497546953,-6.8902042800649));
#51601=CARTESIAN_POINT('Ctrl Pts',(3.21353227400634,1.48486037185928,-6.89525215442485));
#51602=CARTESIAN_POINT('Ctrl Pts',(3.23176253970101,1.44540646206153,-6.89671769002653));
#51603=CARTESIAN_POINT('Ctrl Pts',(3.2492569706675,1.40561255518628,-6.89818322562822));
#51604=CARTESIAN_POINT('Ctrl Pts',(3.26600829512753,1.36550806014452,-6.89964876122991));
#51605=CARTESIAN_POINT('Ctrl Pts',(3.34045769334387,1.18726809298532,-6.90616217119164));
#51606=CARTESIAN_POINT('Ctrl Pts',(3.4002225314738,1.00291223761149,-6.91267558115337));
#51607=CARTESIAN_POINT('Ctrl Pts',(3.44470072231061,0.814949462094048,-6.91918899111509));
#51608=CARTESIAN_POINT('Ctrl Pts',(3.48917891314677,0.626986686579336,-6.92570240107673));
#51609=CARTESIAN_POINT('Ctrl Pts',(3.51837528864164,0.435393488100818,-6.93221581103837));
#51610=CARTESIAN_POINT('Ctrl Pts',(3.53166214900558,0.242686469356258,-6.938729221));
#51611=CARTESIAN_POINT('Ctrl Pts',(3.53340607022177,0.217393371567027,-6.9395841162507));
#51612=CARTESIAN_POINT('Ctrl Pts',(3.53487587375559,0.192081558293536,-6.9404390115014));
#51613=CARTESIAN_POINT('Ctrl Pts',(3.53607015736517,0.16675683551214,-6.9412939067521));
#51614=CARTESIAN_POINT('Ctrl Pts',(3.54397506895323,-0.000866409899313997,
-6.94695242146303));
#51615=CARTESIAN_POINT('Ctrl Pts',(3.53980817195322,-0.169055081500192,
-6.95261093617397));
#51616=CARTESIAN_POINT('Ctrl Pts',(3.52382484364409,-0.336095312099889,
-6.95826945088491));
#51617=CARTESIAN_POINT('Ctrl Pts',(3.50542673475007,-0.52837218290042,-6.96478286084664));
#51618=CARTESIAN_POINT('Ctrl Pts',(3.47137388730705,-0.719151067248053,
-6.97129627080837));
#51619=CARTESIAN_POINT('Ctrl Pts',(3.42203117938897,-0.905902528285193,
-6.97780968077025));
#51620=CARTESIAN_POINT('Ctrl Pts',(3.39797659515054,-0.99694391901358,-6.98098496999166));
#51621=CARTESIAN_POINT('Ctrl Pts',(3.37028711544748,-1.08702913815711,-6.9841602592131));
#51622=CARTESIAN_POINT('Ctrl Pts',(3.33900820913433,-1.17585040686805,-6.98733554843455));
#51623=CARTESIAN_POINT('Ctrl Pts',(3.30612529402972,-1.2692265054204,-6.99067366917496));
#51624=CARTESIAN_POINT('Ctrl Pts',(3.2692753640432,-1.3612056436035,-6.99401178991538));
#51625=CARTESIAN_POINT('Ctrl Pts',(3.2286413672435,-1.45147605409633,-6.99734991065576));
#51626=CARTESIAN_POINT('Ctrl Pts',(3.14935547553055,-1.62761353883595,-7.00386332061764));
#51627=CARTESIAN_POINT('Ctrl Pts',(3.05566316088876,-1.79725369188204,-7.01037673057937));
#51628=CARTESIAN_POINT('Ctrl Pts',(2.94886369882296,-1.95819733025196,-7.0168901405411));
#51629=CARTESIAN_POINT('Ctrl Pts',(2.85875186152997,-2.09399321043342,-7.02238581746063));
#51630=CARTESIAN_POINT('Ctrl Pts',(2.75929726145042,-2.22360994758072,-7.02788149438017));
#51631=CARTESIAN_POINT('Ctrl Pts',(2.65130325159267,-2.34567497068367,-7.0333771712997));
#51632=CARTESIAN_POINT('Ctrl Pts',(2.63130406426958,-2.36827993984675,-7.03439490434181));
#51633=CARTESIAN_POINT('Ctrl Pts',(2.61101205412421,-2.39062594672813,-7.0354126373839));
#51634=CARTESIAN_POINT('Ctrl Pts',(2.5904352191543,-2.41270682914795,-7.036430370426));
#51635=CARTESIAN_POINT('Ctrl Pts',(2.45874512329616,-2.55402270822995,-7.04294378038764));
#51636=CARTESIAN_POINT('Ctrl Pts',(2.3154071367893,-2.68446116186662,-7.04945719034927));
#51637=CARTESIAN_POINT('Ctrl Pts',(2.1624843817763,-2.80245664730059,-7.05597060031091));
#51638=CARTESIAN_POINT('Ctrl Pts',(2.00956162676109,-2.92045213273626,-7.06248401027264));
#51639=CARTESIAN_POINT('Ctrl Pts',(1.84703531539659,-3.02601956514964,-7.06899742023437));
#51640=CARTESIAN_POINT('Ctrl Pts',(1.67694939807015,-3.11757873618206,-7.0755108301961));
#51641=CARTESIAN_POINT('Ctrl Pts',(1.64293177974845,-3.13589080447667,-7.07681352884119));
#51642=CARTESIAN_POINT('Ctrl Pts',(1.60861252646917,-3.15364206036475,-7.07811622748629));
#51643=CARTESIAN_POINT('Ctrl Pts',(1.57400853431423,-3.17081963124785,-7.07941892613138));
#51644=CARTESIAN_POINT('Ctrl Pts',(1.43559477745792,-3.2395288168513,-7.08462963744792));
#51645=CARTESIAN_POINT('Ctrl Pts',(1.29262501833188,-3.29905833593406,-7.08984034876446));
#51646=CARTESIAN_POINT('Ctrl Pts',(1.14641104468838,-3.34905016806174,-7.095051060081));
#51647=CARTESIAN_POINT('Ctrl Pts',(0.963642993532519,-3.41154015793072,
-7.10156447004264));
#51648=CARTESIAN_POINT('Ctrl Pts',(0.775786184883246,-3.45913891306697,
-7.10807788000427));
#51649=CARTESIAN_POINT('Ctrl Pts',(0.585300931640267,-3.49116675003133,
-7.11459128996591));
#51650=CARTESIAN_POINT('Ctrl Pts',(0.479343748210392,-3.50898219421044,
-7.11821436609547));
#51651=CARTESIAN_POINT('Ctrl Pts',(0.372569808297704,-3.52197909098866,
-7.12183744222504));
#51652=CARTESIAN_POINT('Ctrl Pts',(0.265424692965157,-3.53003537267917,
-7.1254605183546));
#51653=CARTESIAN_POINT('Ctrl Pts',(0.1799489423262,-3.53646232665386,-7.12835085218676));
#51654=CARTESIAN_POINT('Ctrl Pts',(0.0942370119385343,-3.53974508577457,
-7.13124118601892));
#51655=CARTESIAN_POINT('Ctrl Pts',(0.00852186074184726,-3.53991094251116,
-7.13413151985108));
#51656=CARTESIAN_POINT('Ctrl Pts',(-0.184638497918042,-3.54028470311567,
-7.1406449298127));
#51657=CARTESIAN_POINT('Ctrl Pts',(-0.377816489562962,-3.52483316308227,
-7.1471583397743));
#51658=CARTESIAN_POINT('Ctrl Pts',(-0.568472409011395,-3.49386453342436,
-7.15367174973592));
#51659=CARTESIAN_POINT('Ctrl Pts',(-0.742445766719096,-3.46560568627825,
-7.15961523055953));
#51660=CARTESIAN_POINT('Ctrl Pts',(-0.914338116430782,-3.42442020539666,
-7.16555871138316));
#51661=CARTESIAN_POINT('Ctrl Pts',(-1.08216137956925,-3.37053805030733,
-7.17150219220678));
#51662=CARTESIAN_POINT('Ctrl Pts',(-1.09825419967799,-3.36537121102231,
-7.17207212134489));
#51663=CARTESIAN_POINT('Ctrl Pts',(-1.11430960469959,-3.3600876333587,-7.17264205048299));
#51664=CARTESIAN_POINT('Ctrl Pts',(-1.13032604705382,-3.35468816325393,
-7.17321197962109));
#51665=CARTESIAN_POINT('Ctrl Pts',(-1.31336925050718,-3.29298055784017,
-7.17972538958273));
#51666=CARTESIAN_POINT('Ctrl Pts',(-1.49129514513555,-3.21614619228149,
-7.18623879954437));
#51667=CARTESIAN_POINT('Ctrl Pts',(-1.66183108821857,-3.12544975106934,
-7.192752209506));
#51668=CARTESIAN_POINT('Ctrl Pts',(-1.83236703130161,-3.0347533098572,-7.19926561946763));
#51669=CARTESIAN_POINT('Ctrl Pts',(-1.99553483595644,-2.93018474734963,
-7.20577902942927));
#51670=CARTESIAN_POINT('Ctrl Pts',(-2.14907398699859,-2.81297668049842,
-7.21229243939091));
#51671=CARTESIAN_POINT('Ctrl Pts',(-2.19033810662407,-2.78147665162115,
-7.21404293837441));
#51672=CARTESIAN_POINT('Ctrl Pts',(-2.23090577145553,-2.74906427885111,
-7.21579343735791));
#51673=CARTESIAN_POINT('Ctrl Pts',(-2.27073169575485,-2.71576463742649,
-7.21754393634141));
#51674=CARTESIAN_POINT('Ctrl Pts',(-2.37909355934424,-2.62516005598574,
-7.22230684731964));
#51675=CARTESIAN_POINT('Ctrl Pts',(-2.48196353080434,-2.52798626286371,
-7.22706975829786));
#51676=CARTESIAN_POINT('Ctrl Pts',(-2.57868524344307,-2.42505371417111,
-7.23183266927608));
#51677=CARTESIAN_POINT('Ctrl Pts',(-2.71095480915343,-2.28429066168171,
-7.2383460792377));
#51678=CARTESIAN_POINT('Ctrl Pts',(-2.83174365337413,-2.13274635689841,
-7.2448594891993));
#51679=CARTESIAN_POINT('Ctrl Pts',(-2.93944340626971,-1.97240050926644,
-7.25137289916092));
#51680=CARTESIAN_POINT('Ctrl Pts',(-3.00675548551217,-1.8721847509957,-7.25544376428074));
#51681=CARTESIAN_POINT('Ctrl Pts',(-3.0689565651283,-1.76852498435215,-7.25951462940056));
#51682=CARTESIAN_POINT('Ctrl Pts',(-3.12563447872083,-1.66192933226244,
-7.26358549452038));
#51683=CARTESIAN_POINT('Ctrl Pts',(-3.15964158566754,-1.59797126622053,
-7.26602803936228));
#51684=CARTESIAN_POINT('Ctrl Pts',(-3.19166042350247,-1.53295634899612,
-7.26847058420419));
#51685=CARTESIAN_POINT('Ctrl Pts',(-3.22164958182273,-1.467019693314,-7.2709131290461));
#51686=CARTESIAN_POINT('Ctrl Pts',(-3.30162014334238,-1.29118977093615,
-7.27742653900773));
#51687=CARTESIAN_POINT('Ctrl Pts',(-3.36715796958855,-1.10881135569454,
-7.28393994896937));
#51688=CARTESIAN_POINT('Ctrl Pts',(-3.41752451187652,-0.92233949801837,
-7.290453358931));
#51689=CARTESIAN_POINT('Ctrl Pts',(-3.46694667627976,-0.739364006987898,
-7.29684464178121));
#51690=CARTESIAN_POINT('Ctrl Pts',(-3.50176440608703,-0.552424156172237,
-7.30323592463143));
#51691=CARTESIAN_POINT('Ctrl Pts',(-3.52124797259483,-0.363885580226897,
-7.3096272074818));
#51692=CARTESIAN_POINT('Ctrl Pts',(-3.52162027213994,-0.360282911997128,
-7.30974933459322));
#51693=CARTESIAN_POINT('Ctrl Pts',(-3.52198697295808,-0.35667966015706,
-7.30987146170465));
#51694=CARTESIAN_POINT('Ctrl Pts',(-3.52234807653483,-0.353075841902743,
-7.30999358881607));
#51695=CARTESIAN_POINT('Ctrl Pts',(-3.54160682757397,-0.160873263421083,
-7.31650699877797));
#51696=CARTESIAN_POINT('Ctrl Pts',(-3.54494113425226,0.0329083541594109,
-7.32302040874003));
#51697=CARTESIAN_POINT('Ctrl Pts',(-3.53259533909181,0.22566737745008,-7.32953381870193));
#51698=CARTESIAN_POINT('Ctrl Pts',(-3.52024954393154,0.418426400737956,
-7.33604722866373));
#51699=CARTESIAN_POINT('Ctrl Pts',(-3.49222452843905,0.610186888018826,
-7.34256063862537));
#51700=CARTESIAN_POINT('Ctrl Pts',(-3.44874073224416,0.798391072008908,
-7.349074048587));
#51701=CARTESIAN_POINT('Ctrl Pts',(-3.43406482543378,0.861910527697223,
-7.35127234326179));
#51702=CARTESIAN_POINT('Ctrl Pts',(-3.4176279918563,0.925023822733724,-7.35347063793657));
#51703=CARTESIAN_POINT('Ctrl Pts',(-3.399439647296,0.987628515379085,-7.35566893261136));
#51704=CARTESIAN_POINT('Ctrl Pts',(-3.36373706176239,1.11051762090298,-7.35998404789821));
#51705=CARTESIAN_POINT('Ctrl Pts',(-3.32128518726173,1.23144678337572,-7.36429916318506));
#51706=CARTESIAN_POINT('Ctrl Pts',(-3.27244048985516,1.34972428826295,-7.36861427847191));
#51707=CARTESIAN_POINT('Ctrl Pts',(-3.19871232327865,1.52825714946575,-7.37512768843364));
#51708=CARTESIAN_POINT('Ctrl Pts',(-3.11041628697104,1.7007662450445,-7.38164109839537));
#51709=CARTESIAN_POINT('Ctrl Pts',(-3.00872059248994,1.86498453844867,-7.38815450835708));
#51710=CARTESIAN_POINT('Ctrl Pts',(-2.9381695165832,1.97891047545466,-7.39267316652609));
#51711=CARTESIAN_POINT('Ctrl Pts',(-2.86116271344563,2.08885271017646,-7.3971918246951));
#51712=CARTESIAN_POINT('Ctrl Pts',(-2.77810835168668,2.19401777255465,-7.40171048286411));
#51713=CARTESIAN_POINT('Ctrl Pts',(-2.74144418484653,2.24044265995526,-7.40370523465671));
#51714=CARTESIAN_POINT('Ctrl Pts',(-2.70360160799484,2.2859366567572,-7.40569998644932));
#51715=CARTESIAN_POINT('Ctrl Pts',(-2.66463875530979,2.33044965099088,-7.40769473824192));
#51716=CARTESIAN_POINT('Ctrl Pts',(-2.53741438897186,2.47579674687627,-7.41420814820364));
#51717=CARTESIAN_POINT('Ctrl Pts',(-2.39825532545772,2.61067669790369,-7.42072155816537));
#51718=CARTESIAN_POINT('Ctrl Pts',(-2.24911868144474,2.73342304268973,-7.4272349681271));
#51719=CARTESIAN_POINT('Ctrl Pts',(-2.09998203743392,2.85616938747399,-7.43374837808873));
#51720=CARTESIAN_POINT('Ctrl Pts',(-1.94084807500285,2.96679585561946,-7.44026178805037));
#51721=CARTESIAN_POINT('Ctrl Pts',(-1.7736881360114,3.06359595272342,-7.446775198012));
#51722=CARTESIAN_POINT('Ctrl Pts',(-1.76533007352107,3.0684359955324,-7.44710087106389));
#51723=CARTESIAN_POINT('Ctrl Pts',(-1.75695201419097,3.07324143239533,-7.44742654411577));
#51724=CARTESIAN_POINT('Ctrl Pts',(-1.74855420770786,3.07801205044834,-7.44775221716766));
#51725=CARTESIAN_POINT('Ctrl Pts',(-1.58899720157694,3.16865304526785,-7.45393995407741));
#51726=CARTESIAN_POINT('Ctrl Pts',(-1.42231138155771,3.24672375067996,-7.46012769098716));
#51727=CARTESIAN_POINT('Ctrl Pts',(-1.25063380441199,3.31151429393604,-7.46631542789691));
#51728=CARTESIAN_POINT('Ctrl Pts',(-1.0699204907246,3.37971489393329,-7.47282883785864));
#51729=CARTESIAN_POINT('Ctrl Pts',(-0.883654985072044,3.43321218577804,
-7.47934224782037));
#51730=CARTESIAN_POINT('Ctrl Pts',(-0.69426261018899,3.47118330719089,-7.4858556577821));
#51731=CARTESIAN_POINT('Ctrl Pts',(-0.61732158273511,3.48660915047991,-7.48850174348113));
#51732=CARTESIAN_POINT('Ctrl Pts',(-0.539864762333473,3.49947197571339,
-7.49114782918016));
#51733=CARTESIAN_POINT('Ctrl Pts',(-0.462062720458959,3.5097148092635,-7.49379391487919));
#51734=CARTESIAN_POINT('Ctrl Pts',(-0.34835297767497,3.52468498151477,-7.4976612391418));
#51735=CARTESIAN_POINT('Ctrl Pts',(-0.233905849409282,3.53405841436472,
-7.5015285634044));
#51736=CARTESIAN_POINT('Ctrl Pts',(-0.119281726467647,3.53786972306194,
-7.505395887667));
#51737=CARTESIAN_POINT('Ctrl Pts',(0.0737700720151849,3.54428879070397,
-7.51190929762864));
#51738=CARTESIAN_POINT('Ctrl Pts',(0.267337123262925,3.53493519022353,-7.51842270759027));
#51739=CARTESIAN_POINT('Ctrl Pts',(0.45887316707087,3.50996979757638,-7.52493611755191));
#51740=CARTESIAN_POINT('Ctrl Pts',(0.604918840965994,3.49093375861096,-7.52990257362091));
#51741=CARTESIAN_POINT('Ctrl Pts',(0.749795644587637,3.46281672251746,-7.53486902968991));
#51742=CARTESIAN_POINT('Ctrl Pts',(0.892325528180709,3.42569046350633,-7.5398354857589));
#51743=CARTESIAN_POINT('Ctrl Pts',(0.936720798206521,3.4141263602299,-7.54138243965163));
#51744=CARTESIAN_POINT('Ctrl Pts',(0.98088838046976,3.40168827258433,-7.54292939354435));
#51745=CARTESIAN_POINT('Ctrl Pts',(1.02479609483758,3.38839156064891,-7.54447634743708));
#51746=CARTESIAN_POINT('Ctrl Pts',(1.2096684077747,3.33240609373605,-7.5509897573987));
#51747=CARTESIAN_POINT('Ctrl Pts',(1.38991621050558,3.26120588847558,-7.5575031673603));
#51748=CARTESIAN_POINT('Ctrl Pts',(1.56321999725237,3.17591743890142,-7.56401657732192));
#51749=CARTESIAN_POINT('Ctrl Pts',(1.73652378400167,3.09062898932603,-7.57052998728364));
#51750=CARTESIAN_POINT('Ctrl Pts',(1.90290467519647,2.99124089947101,-7.57704339724536));
#51751=CARTESIAN_POINT('Ctrl Pts',(2.06001785169516,2.87886643810324,-7.58355680720709));
#51752=CARTESIAN_POINT('Ctrl Pts',(2.07867525608196,2.86552181726869,-7.5843302835399));
#51753=CARTESIAN_POINT('Ctrl Pts',(2.09720163827227,2.85199428966467,-7.5851037598727));
#51754=CARTESIAN_POINT('Ctrl Pts',(2.11559302029352,2.83828578062299,-7.5858772362055));
#51755=CARTESIAN_POINT('Ctrl Pts',(2.25207465220354,2.73655554181339,-7.59161716983433));
#51756=CARTESIAN_POINT('Ctrl Pts',(2.38112092105923,2.62485779238668,-7.59735710346317));
#51757=CARTESIAN_POINT('Ctrl Pts',(2.50151996034344,2.50453286898932,-7.603097037092));
#51758=CARTESIAN_POINT('Ctrl Pts',(2.63814319548082,2.36799373711636,-7.60961044705364));
#51759=CARTESIAN_POINT('Ctrl Pts',(2.76365118020096,2.22033192223027,-7.61612385701527));
#51760=CARTESIAN_POINT('Ctrl Pts',(2.87632012344211,2.06343515614491,-7.6226372669769));
#51761=CARTESIAN_POINT('Ctrl Pts',(2.92983793594804,1.98890910248192,-7.62573114043549));
#51762=CARTESIAN_POINT('Ctrl Pts',(2.98045881580538,1.91229818395693,-7.62882501389408));
#51763=CARTESIAN_POINT('Ctrl Pts',(3.02798948096801,1.83381561318099,-7.63191888735267));
#51764=CARTESIAN_POINT('Ctrl Pts',(3.08052325350839,1.74707191819124,-7.63533842385581));
#51765=CARTESIAN_POINT('Ctrl Pts',(3.12928194035441,1.65804182176638,-7.63875796035895));
#51766=CARTESIAN_POINT('Ctrl Pts',(3.17413145383252,1.5670900227261,-7.64217749686209));
#51767=CARTESIAN_POINT('Ctrl Pts',(3.25955919165442,1.39384831194062,-7.64869090682373));
#51768=CARTESIAN_POINT('Ctrl Pts',(3.33081116461456,1.21362870349055,-7.65520431678536));
#51769=CARTESIAN_POINT('Ctrl Pts',(3.38701269619474,1.02883041976208,-7.66171772674717));
#51770=CARTESIAN_POINT('Ctrl Pts',(3.43373009893555,0.87521724225577,-7.66713198482601));
#51771=CARTESIAN_POINT('Ctrl Pts',(3.47004976409285,0.718424299931465,-7.67254624290497));
#51772=CARTESIAN_POINT('Ctrl Pts',(3.49544487589833,0.559879558080886,-7.67796050098386));
#51773=CARTESIAN_POINT('Ctrl Pts',(3.50060035326059,0.527693291929511,-7.67905965286682));
#51774=CARTESIAN_POINT('Ctrl Pts',(3.50530563687768,0.495434842487014,-7.68015880474978));
#51775=CARTESIAN_POINT('Ctrl Pts',(3.50956112158859,0.463116931447565,-7.68125795663274));
#51776=CARTESIAN_POINT('Ctrl Pts',(3.53477848866818,0.271605815489876,-7.68777136659463));
#51777=CARTESIAN_POINT('Ctrl Pts',(3.54419862852173,0.0780313815552228,
-7.69428477655637));
#51778=CARTESIAN_POINT('Ctrl Pts',(3.53792067981413,-0.115020209061044,
-7.70079818651808));
#51779=CARTESIAN_POINT('Ctrl Pts',(3.53164273110663,-0.308071799674505,
-7.7073115964797));
#51780=CARTESIAN_POINT('Ctrl Pts',(3.50966604727128,-0.500624506508935,
-7.7138250064413));
#51781=CARTESIAN_POINT('Ctrl Pts',(3.47206668295341,-0.690093950472241,
-7.72033841640292));
#51782=CARTESIAN_POINT('Ctrl Pts',(3.46501671280743,-0.725619921396251,
-7.72155969624664));
#51783=CARTESIAN_POINT('Ctrl Pts',(3.45741761512174,-0.761036669986838,
-7.72278097609036));
#51784=CARTESIAN_POINT('Ctrl Pts',(3.44927002934,-0.796326732377223,-7.72400225593407));
#51785=CARTESIAN_POINT('Ctrl Pts',(3.41396437492646,-0.949247951050361,
-7.72929438605207));
#51786=CARTESIAN_POINT('Ctrl Pts',(3.36835867813816,-1.09978996669337,-7.73458651617007));
#51787=CARTESIAN_POINT('Ctrl Pts',(3.31303614425419,-1.24665390493681,-7.739878646288));
#51788=CARTESIAN_POINT('Ctrl Pts',(3.24494668131607,-1.42741002686256,-7.74639205542224));
#51789=CARTESIAN_POINT('Ctrl Pts',(3.16213450638776,-1.60261748080289,-7.75290546455638));
#51790=CARTESIAN_POINT('Ctrl Pts',(3.06563512458071,-1.76994524026474,-7.75941887369107));
#51791=CARTESIAN_POINT('Ctrl Pts',(0.4410246309536,-3.491069428017,-4.85718848779));
#51792=CARTESIAN_POINT('Ctrl Pts',(-0.007831201098047,-3.547773106292,-4.872535710012));
#51793=CARTESIAN_POINT('Ctrl Pts',(-0.9274923506371,-3.485867209753,-4.903230154456));
#51794=CARTESIAN_POINT('Ctrl Pts',(-2.170848424879,-2.880804771784,-4.949271821123));
#51795=CARTESIAN_POINT('Ctrl Pts',(-3.09517319399,-1.85242382625,-4.99531348779));
#51796=CARTESIAN_POINT('Ctrl Pts',(-3.564695695909,-0.5518440355064,-5.041355154456));
#51797=CARTESIAN_POINT('Ctrl Pts',(-3.510409115218,0.8298255998088,-5.087396821123));
#51798=CARTESIAN_POINT('Ctrl Pts',(-2.940294193437,2.08955828983,-5.13343848779));
#51799=CARTESIAN_POINT('Ctrl Pts',(-1.938124180797,3.042245589626,-5.179480154456));
#51800=CARTESIAN_POINT('Ctrl Pts',(-0.6511609504327,3.5478969849,-5.225521821123));
#51801=CARTESIAN_POINT('Ctrl Pts',(0.7314856681681,3.532210684072,-5.27156348779));
#51802=CARTESIAN_POINT('Ctrl Pts',(2.006645775638,2.997491672717,-5.317605154456));
#51803=CARTESIAN_POINT('Ctrl Pts',(2.986943859211,2.022313027209,-5.363646821123));
#51804=CARTESIAN_POINT('Ctrl Pts',(3.528332232803,0.7499701678353,-5.40968848779));
#51805=CARTESIAN_POINT('Ctrl Pts',(3.551257806707,-0.6325753616011,-5.455730154456));
#51806=CARTESIAN_POINT('Ctrl Pts',(3.052351834218,-1.922168535253,-5.501771821123));
#51807=CARTESIAN_POINT('Ctrl Pts',(2.104924925093,-2.929313000944,-5.54781348779));
#51808=CARTESIAN_POINT('Ctrl Pts',(0.8481945836498,-3.506016193067,-5.593855154456));
#51809=CARTESIAN_POINT('Ctrl Pts',(-0.5331717924892,-3.567535765409,-5.639896821123));
#51810=CARTESIAN_POINT('Ctrl Pts',(-1.836192445479,-3.104831863555,-5.68593848779));
#51811=CARTESIAN_POINT('Ctrl Pts',(-2.869397952564,-2.185895465844,-5.731980154456));
#51812=CARTESIAN_POINT('Ctrl Pts',(-3.480966267353,-0.9457576028406,-5.778021821123));
#51813=CARTESIAN_POINT('Ctrl Pts',(-3.581031867039,0.4333524720513,-5.82406348779));
#51814=CARTESIAN_POINT('Ctrl Pts',(-3.154890838399,1.74878454807,-5.870105154456));
#51815=CARTESIAN_POINT('Ctrl Pts',(-2.265161511065,2.807245433975,-5.916146821123));
#51816=CARTESIAN_POINT('Ctrl Pts',(-1.042583148702,3.453201988854,-5.96218848779));
#51817=CARTESIAN_POINT('Ctrl Pts',(0.3331952363912,3.591735587738,-6.008230154456));
#51818=CARTESIAN_POINT('Ctrl Pts',(1.660013001075,3.202489724268,-6.054271821123));
#51819=CARTESIAN_POINT('Ctrl Pts',(2.742903909839,2.342661251476,-6.10031348779));
#51820=CARTESIAN_POINT('Ctrl Pts',(3.422745007318,1.138595719585,-6.146355154456));
#51821=CARTESIAN_POINT('Ctrl Pts',(3.599638581068,-0.2327781851084,-6.192396821123));
#51822=CARTESIAN_POINT('Ctrl Pts',(3.247591404983,-1.569947025876,-6.23843848779));
#51823=CARTESIAN_POINT('Ctrl Pts',(2.418334255113,-2.676423551744,-6.284480154456));
#51824=CARTESIAN_POINT('Ctrl Pts',(1.233720447776,-3.389619072185,-6.330521821123));
#51825=CARTESIAN_POINT('Ctrl Pts',(-0.1321796203991,-3.604734684513,-6.37656348779));
#51826=CARTESIAN_POINT('Ctrl Pts',(-1.478656853211,-3.290160711611,-6.422605154456));
#51827=CARTESIAN_POINT('Ctrl Pts',(-2.607856199071,-2.492121514442,-6.468646821123));
#51828=CARTESIAN_POINT('Ctrl Pts',(-3.353850014061,-1.327883157873,-6.51468848779));
#51829=CARTESIAN_POINT('Ctrl Pts',(-3.607019924283,0.03147798599785,-6.560730154456));
#51830=CARTESIAN_POINT('Ctrl Pts',(-3.330164449886,1.386213668412,-6.606771821123));
#51831=CARTESIAN_POINT('Ctrl Pts',(-2.563965492379,2.537255318581,-6.65281348779));
#51832=CARTESIAN_POINT('Ctrl Pts',(-1.421010424628,3.315465724582,-6.698855154456));
#51833=CARTESIAN_POINT('Ctrl Pts',(-0.06924819399,3.606492518418,-6.744896821123));
#51834=CARTESIAN_POINT('Ctrl Pts',(1.292689555892,3.367571426097,-6.79093848779));
#51835=CARTESIAN_POINT('Ctrl Pts',(2.464675962715,2.633810167152,-6.836980154456));
#51836=CARTESIAN_POINT('Ctrl Pts',(3.274496134663,1.513029630198,-6.883021821123));
#51837=CARTESIAN_POINT('Ctrl Pts',(3.603152878174,0.1699203763192,-6.92906348779));
#51838=CARTESIAN_POINT('Ctrl Pts',(3.402352471409,-1.198157442941,-6.975105154456));
#51839=CARTESIAN_POINT('Ctrl Pts',(2.701601075983,-2.390174726673,-7.021146821123));
#51840=CARTESIAN_POINT('Ctrl Pts',(1.603869020775,-3.230973191157,-7.06718848779));
#51841=CARTESIAN_POINT('Ctrl Pts',(0.2704600598501,-3.5970036077,-7.113230154456));
#51842=CARTESIAN_POINT('Ctrl Pts',(-1.102691042857,-3.434480464608,-7.159271821123));
#51843=CARTESIAN_POINT('Ctrl Pts',(-2.313809704281,-2.767285357563,-7.20531348779));
#51844=CARTESIAN_POINT('Ctrl Pts',(-3.184930831936,-1.693457762528,-7.251355154456));
#51845=CARTESIAN_POINT('Ctrl Pts',(-3.588049502055,-0.3707888467895,-7.297396821123));
#51846=CARTESIAN_POINT('Ctrl Pts',(-3.463930353097,1.00636479757,-7.34343848779));
#51847=CARTESIAN_POINT('Ctrl Pts',(-2.830811793846,2.235640442297,-7.389480154456));
#51848=CARTESIAN_POINT('Ctrl Pts',(-1.781725994683,3.136404960891,-7.435521821123));
#51849=CARTESIAN_POINT('Ctrl Pts',(-0.4708285118613,3.576297537987,-7.48156348779));
#51850=CARTESIAN_POINT('Ctrl Pts',(0.9092538495968,3.490679192871,-7.527605154456));
#51851=CARTESIAN_POINT('Ctrl Pts',(2.155727782029,2.892130773684,-7.573646821123));
#51852=CARTESIAN_POINT('Ctrl Pts',(3.085433837764,1.868605168765,-7.61968848779));
#51853=CARTESIAN_POINT('Ctrl Pts',(3.561755309148,0.5705000005301,-7.665730154456));
#51854=CARTESIAN_POINT('Ctrl Pts',(3.514711985961,-0.8114300171164,-7.711771821123));
#51855=CARTESIAN_POINT('Ctrl Pts',(2.951172612682,-2.074148614413,-7.75781348779));
#51856=CARTESIAN_POINT('Ctrl Pts',(2.286463642788,-2.712718074487,-7.788507932234));
#51857=CARTESIAN_POINT('Ctrl Pts',(1.906171705064,-2.957799504219,-7.803855154456));
#51858=CARTESIAN_POINT('Ctrl Pts',(0.4620124040095,-3.657204758643,-4.953869121321));
#51859=CARTESIAN_POINT('Ctrl Pts',(-0.008203877497198,-3.716606889221,-4.969216343543));
#51860=CARTESIAN_POINT('Ctrl Pts',(-0.9716304726375,-3.65175497376,-4.999910787988));
#51861=CARTESIAN_POINT('Ctrl Pts',(-2.274156201548,-3.017898422626,-5.045952454654));
#51862=CARTESIAN_POINT('Ctrl Pts',(-3.242468351686,-1.94057820163,-5.091994121321));
#51863=CARTESIAN_POINT('Ctrl Pts',(-3.734334802272,-0.5781055559897,-5.138035787988));
#51864=CARTESIAN_POINT('Ctrl Pts',(-3.677464795723,0.8693158916029,-5.184077454654));
#51865=CARTESIAN_POINT('Ctrl Pts',(-3.080218866387,2.188997577561,-5.230119121321));
#51866=CARTESIAN_POINT('Ctrl Pts',(-2.030356921569,3.187021993332,-5.276160787988));
#51867=CARTESIAN_POINT('Ctrl Pts',(-0.6821488302275,3.716736663046,-5.322202454654));
#51868=CARTESIAN_POINT('Ctrl Pts',(0.7662960939803,3.700303872116,-5.368244121321));
#51869=CARTESIAN_POINT('Ctrl Pts',(2.102139367575,3.140138297301,-5.414285787988));
#51870=CARTESIAN_POINT('Ctrl Pts',(3.129088527441,2.11855220272,-5.460327454654));
#51871=CARTESIAN_POINT('Ctrl Pts',(3.696240850532,0.7856602462946,-5.506369121321));
#51872=CARTESIAN_POINT('Ctrl Pts',(3.720257421874,-0.6626787780505,-5.552410787988));
#51873=CARTESIAN_POINT('Ctrl Pts',(3.197609180605,-2.013641968167,-5.598452454654));
#51874=CARTESIAN_POINT('Ctrl Pts',(2.20509549047,-3.068715093613,-5.644494121321));
#51875=CARTESIAN_POINT('Ctrl Pts',(0.8885590308471,-3.672862820275,-5.690535787988));
#51876=CARTESIAN_POINT('Ctrl Pts',(-0.5585447258702,-3.737310026886,-5.736577454654));
#51877=CARTESIAN_POINT('Ctrl Pts',(-1.92357439113,-3.252586664433,-5.782619121321));
#51878=CARTESIAN_POINT('Ctrl Pts',(-3.005948768117,-2.289919311093,-5.828660787988));
#51879=CARTESIAN_POINT('Ctrl Pts',(-3.646620802058,-0.9907649437943,-5.874702454654));
#51880=CARTESIAN_POINT('Ctrl Pts',(-3.751448389963,0.4539751373136,-5.920744121321));
#51881=CARTESIAN_POINT('Ctrl Pts',(-3.30502787902,1.832006868644,-5.966785787988));
#51882=CARTESIAN_POINT('Ctrl Pts',(-2.372957521519,2.940838494192,-6.012827454654));
#51883=CARTESIAN_POINT('Ctrl Pts',(-1.092198288041,3.617535258634,-6.058869121321));
#51884=CARTESIAN_POINT('Ctrl Pts',(0.3490515526009,3.762661486433,-6.104910787988));
#51885=CARTESIAN_POINT('Ctrl Pts',(1.739010802311,3.354891932284,-6.150952454654));
#51886=CARTESIAN_POINT('Ctrl Pts',(2.873435042872,2.454145371051,-6.196994121321));
#51887=CARTESIAN_POINT('Ctrl Pts',(3.585628870032,1.192779968917,-6.243035787988));
#51888=CARTESIAN_POINT('Ctrl Pts',(3.770940572659,-0.2438557879871,-6.289077454654));
#51889=CARTESIAN_POINT('Ctrl Pts',(3.402139941737,-1.644658707665,-6.335119121321));
#51890=CARTESIAN_POINT('Ctrl Pts',(2.533419551845,-2.803790973341,-6.381160787988));
#51891=CARTESIAN_POINT('Ctrl Pts',(1.292431555853,-3.550926515896,-6.427202454654));
#51892=CARTESIAN_POINT('Ctrl Pts',(-0.1384698719652,-3.776279192858,-6.473244121321));
#51893=CARTESIAN_POINT('Ctrl Pts',(-1.549024157631,-3.446735064802,-6.519285787988));
#51894=CARTESIAN_POINT('Ctrl Pts',(-2.731960591949,-2.610718248279,-6.565327454654));
#51895=CARTESIAN_POINT('Ctrl Pts',(-3.513455256077,-1.391075343539,-6.611369121321));
#51896=CARTESIAN_POINT('Ctrl Pts',(-3.778673184137,0.03297598130245,-6.657410787988));
#51897=CARTESIAN_POINT('Ctrl Pts',(-3.488642527544,1.452181725154,-6.703452454654));
#51898=CARTESIAN_POINT('Ctrl Pts',(-2.685981185156,2.657999909866,-6.749494121321));
#51899=CARTESIAN_POINT('Ctrl Pts',(-1.488634412516,3.473244309537,-6.795535787988));
#51900=CARTESIAN_POINT('Ctrl Pts',(-0.0725436230386,3.778120679731,-6.841577454654));
#51901=CARTESIAN_POINT('Ctrl Pts',(1.354206925051,3.527829651783,-6.887619121321));
#51902=CARTESIAN_POINT('Ctrl Pts',(2.581966599408,2.7591496747,-6.933660787988));
#51903=CARTESIAN_POINT('Ctrl Pts',(3.430325031562,1.585032689158,-6.979702454654));
#51904=CARTESIAN_POINT('Ctrl Pts',(3.774622110468,0.1780066600445,-7.025744121321));
#51905=CARTESIAN_POINT('Ctrl Pts',(3.56426588058,-1.255176155123,-7.071785787988));
#51906=CARTESIAN_POINT('Ctrl Pts',(2.830166662326,-2.503919949063,-7.117827454654));
#51907=CARTESIAN_POINT('Ctrl Pts',(1.680195004987,-3.384730889313,-7.163869121321));
#51908=CARTESIAN_POINT('Ctrl Pts',(0.2833308928114,-3.768180204427,-7.209910787988));
#51909=CARTESIAN_POINT('Ctrl Pts',(-1.155166636586,-3.597922802058,-7.255952454654));
#51910=CARTESIAN_POINT('Ctrl Pts',(-2.423920817265,-2.898976771123,-7.301994121321));
#51911=CARTESIAN_POINT('Ctrl Pts',(-3.336497435721,-1.774047155286,-7.348035787988));
#51912=CARTESIAN_POINT('Ctrl Pts',(-3.758799984856,-0.3884341926996,-7.394077454654));
#51913=CARTESIAN_POINT('Ctrl Pts',(-3.6287741714,1.054256353961,-7.440119121321));
#51914=CARTESIAN_POINT('Ctrl Pts',(-2.965526345649,2.342031584525,-7.486160787988));
#51915=CARTESIAN_POINT('Ctrl Pts',(-1.866515954698,3.285662283295,-7.532202454654));
#51916=CARTESIAN_POINT('Ctrl Pts',(-0.4932346117968,3.746488760516,-7.578244121321));
#51917=CARTESIAN_POINT('Ctrl Pts',(0.9525240256962,3.656795952728,-7.624285787988));
#51918=CARTESIAN_POINT('Ctrl Pts',(2.258315987503,3.029763413827,-7.670327454654));
#51919=CARTESIAN_POINT('Ctrl Pts',(3.232265512507,1.957529592619,-7.716369121321));
#51920=CARTESIAN_POINT('Ctrl Pts',(3.731254486433,0.5976493334679,-7.762410787988));
#51921=CARTESIAN_POINT('Ctrl Pts',(3.681972434336,-0.8500448877034,-7.808452454654));
#51922=CARTESIAN_POINT('Ctrl Pts',(3.091614975073,-2.172854576276,-7.854494121321));
#51923=CARTESIAN_POINT('Ctrl Pts',(2.395273393235,-2.841812703939,-7.885188565765));
#51924=CARTESIAN_POINT('Ctrl Pts',(1.996883870199,-3.098557231525,-7.900535787988));
#51925=CARTESIAN_POINT('Ctrl Pts',(0.4830001770654,-3.823340089268,-5.050549754852));
#51926=CARTESIAN_POINT('Ctrl Pts',(-0.008576553896349,-3.885440672149,-5.065896977074));
#51927=CARTESIAN_POINT('Ctrl Pts',(-1.015768594638,-3.817642737768,-5.096591421519));
#51928=CARTESIAN_POINT('Ctrl Pts',(-2.377463978216,-3.154992073467,-5.142633088185));
#51929=CARTESIAN_POINT('Ctrl Pts',(-3.389763509381,-2.028732577009,-5.188674754852));
#51930=CARTESIAN_POINT('Ctrl Pts',(-3.903973908634,-0.604367076473,-5.234716421519));
#51931=CARTESIAN_POINT('Ctrl Pts',(-3.844520476228,0.908806183397,-5.280758088185));
#51932=CARTESIAN_POINT('Ctrl Pts',(-3.220143539338,2.288436865292,-5.326799754852));
#51933=CARTESIAN_POINT('Ctrl Pts',(-2.12258966234,3.331798397039,-5.372841421519));
#51934=CARTESIAN_POINT('Ctrl Pts',(-0.7131367100223,3.885576341192,-5.418883088185));
#51935=CARTESIAN_POINT('Ctrl Pts',(0.8011065197924,3.86839706016,-5.464924754852));
#51936=CARTESIAN_POINT('Ctrl Pts',(2.197632959513,3.282784921885,-5.510966421519));
#51937=CARTESIAN_POINT('Ctrl Pts',(3.27123319567,2.214791378231,-5.557008088185));
#51938=CARTESIAN_POINT('Ctrl Pts',(3.864149468261,0.8213503247539,-5.603049754852));
#51939=CARTESIAN_POINT('Ctrl Pts',(3.88925703704,-0.6927821944998,-5.649091421519));
#51940=CARTESIAN_POINT('Ctrl Pts',(3.342866526991,-2.105115401081,-5.695133088185));
#51941=CARTESIAN_POINT('Ctrl Pts',(2.305266055846,-3.208117186282,-5.741174754852));
#51942=CARTESIAN_POINT('Ctrl Pts',(0.9289234780445,-3.839709447483,-5.787216421519));
#51943=CARTESIAN_POINT('Ctrl Pts',(-0.5839176592511,-3.907084288362,-5.833258088185));
#51944=CARTESIAN_POINT('Ctrl Pts',(-2.01095633678,-3.400341465311,-5.879299754852));
#51945=CARTESIAN_POINT('Ctrl Pts',(-3.142499583669,-2.393943156341,-5.925341421519));
#51946=CARTESIAN_POINT('Ctrl Pts',(-3.812275336764,-1.035772284748,-5.971383088185));
#51947=CARTESIAN_POINT('Ctrl Pts',(-3.921864912888,0.474597802576,-6.017424754852));
#51948=CARTESIAN_POINT('Ctrl Pts',(-3.455164919641,1.915229189219,-6.063466421519));
#51949=CARTESIAN_POINT('Ctrl Pts',(-2.480753531974,3.07443155441,-6.109508088185));
#51950=CARTESIAN_POINT('Ctrl Pts',(-1.14181342738,3.781868528414,-6.155549754852));
#51951=CARTESIAN_POINT('Ctrl Pts',(0.3649078688106,3.933587385127,-6.201591421519));
#51952=CARTESIAN_POINT('Ctrl Pts',(1.818008603547,3.5072941403,-6.247633088185));
#51953=CARTESIAN_POINT('Ctrl Pts',(3.003966175905,2.565629490626,-6.293674754852));
#51954=CARTESIAN_POINT('Ctrl Pts',(3.748512732746,1.246964218249,-6.339716421519));
#51955=CARTESIAN_POINT('Ctrl Pts',(3.942242564249,-0.2549333908658,-6.385758088185));
#51956=CARTESIAN_POINT('Ctrl Pts',(3.55668847849,-1.719370389453,-6.431799754852));
#51957=CARTESIAN_POINT('Ctrl Pts',(2.648504848577,-2.931158394938,-6.477841421519));
#51958=CARTESIAN_POINT('Ctrl Pts',(1.351142663929,-3.712233959607,-6.523883088185));
#51959=CARTESIAN_POINT('Ctrl Pts',(-0.1447601235313,-3.947823701204,-6.569924754852));
#51960=CARTESIAN_POINT('Ctrl Pts',(-1.61939146205,-3.603309417992,-6.615966421519));
#51961=CARTESIAN_POINT('Ctrl Pts',(-2.856064984826,-2.729314982116,-6.662008088185));
#51962=CARTESIAN_POINT('Ctrl Pts',(-3.673060498094,-1.454267529204,-6.708049754852));
#51963=CARTESIAN_POINT('Ctrl Pts',(-3.95032644399,0.03447397660705,-6.754091421519));
#51964=CARTESIAN_POINT('Ctrl Pts',(-3.647120605201,1.518149781897,-6.800133088185));
#51965=CARTESIAN_POINT('Ctrl Pts',(-2.807996877932,2.778744501151,-6.846174754852));
#51966=CARTESIAN_POINT('Ctrl Pts',(-1.556258400404,3.631022894492,-6.892216421519));
#51967=CARTESIAN_POINT('Ctrl Pts',(-0.07583905208719,3.949748841044,-6.938258088185));
#51968=CARTESIAN_POINT('Ctrl Pts',(1.41572429421,3.688087877469,-6.984299754852));
#51969=CARTESIAN_POINT('Ctrl Pts',(2.699257236101,2.884489182249,-7.030341421519));
#51970=CARTESIAN_POINT('Ctrl Pts',(3.58615392846,1.657035748118,-7.076383088185));
#51971=CARTESIAN_POINT('Ctrl Pts',(3.946091342763,0.1860929437699,-7.122424754852));
#51972=CARTESIAN_POINT('Ctrl Pts',(3.726179289751,-1.312194867306,-7.168466421519));
#51973=CARTESIAN_POINT('Ctrl Pts',(2.958732248669,-2.617665171453,-7.214508088185));
#51974=CARTESIAN_POINT('Ctrl Pts',(1.7565209892,-3.53848858747,-7.260549754852));
#51975=CARTESIAN_POINT('Ctrl Pts',(0.2962017257726,-3.939356801154,-7.306591421519));
#51976=CARTESIAN_POINT('Ctrl Pts',(-1.207642230314,-3.761365139508,-7.352633088185));
#51977=CARTESIAN_POINT('Ctrl Pts',(-2.53403193025,-3.030668184684,-7.398674754852));
#51978=CARTESIAN_POINT('Ctrl Pts',(-3.488064039506,-1.854636548043,-7.444716421519));
#51979=CARTESIAN_POINT('Ctrl Pts',(-3.929550467657,-0.4060795386097,-7.490758088185));
#51980=CARTESIAN_POINT('Ctrl Pts',(-3.793617989703,1.102147910351,-7.536799754852));
#51981=CARTESIAN_POINT('Ctrl Pts',(-3.100240897452,2.448422726752,-7.582841421519));
#51982=CARTESIAN_POINT('Ctrl Pts',(-1.951305914712,3.434919605699,-7.628883088185));
#51983=CARTESIAN_POINT('Ctrl Pts',(-0.5156407117324,3.916679983045,-7.674924754852));
#51984=CARTESIAN_POINT('Ctrl Pts',(0.9957942017955,3.822912712584,-7.720966421519));
#51985=CARTESIAN_POINT('Ctrl Pts',(2.360904192978,3.167396053969,-7.767008088185));
#51986=CARTESIAN_POINT('Ctrl Pts',(3.37909718725,2.046454016473,-7.813049754852));
#51987=CARTESIAN_POINT('Ctrl Pts',(3.900753663718,0.6247986664056,-7.859091421519));
#51988=CARTESIAN_POINT('Ctrl Pts',(3.849232882712,-0.8886597582905,-7.905133088185));
#51989=CARTESIAN_POINT('Ctrl Pts',(3.232057337464,-2.271560538139,-7.951174754852));
#51990=CARTESIAN_POINT('Ctrl Pts',(2.504083143683,-2.97090733339,-7.981869199296));
#51991=CARTESIAN_POINT('Ctrl Pts',(2.087596035333,-3.239314958832,-7.997216421519));
#51992=CARTESIAN_POINT('Ctrl Pts',(0.5039879501212,-3.989475419894,-5.147230388383));
#51993=CARTESIAN_POINT('Ctrl Pts',(-0.0089492302955,-4.054274455078,-5.162577610605));
#51994=CARTESIAN_POINT('Ctrl Pts',(-1.059906716638,-3.983530501776,-5.19327205505));
#51995=CARTESIAN_POINT('Ctrl Pts',(-2.480771754885,-3.292085724309,-5.239313721716));
#51996=CARTESIAN_POINT('Ctrl Pts',(-3.537058667077,-2.116886952389,-5.285355388383));
#51997=CARTESIAN_POINT('Ctrl Pts',(-4.073613014997,-0.6306285969564,-5.33139705505));
#51998=CARTESIAN_POINT('Ctrl Pts',(-4.011576156733,0.9482964751911,-5.377438721716));
#51999=CARTESIAN_POINT('Ctrl Pts',(-3.360068212288,2.387876153023,-5.423480388383));
#52000=CARTESIAN_POINT('Ctrl Pts',(-2.214822403112,3.476574800745,-5.46952205505));
#52001=CARTESIAN_POINT('Ctrl Pts',(-0.7441245898171,4.054416019338,-5.515563721716));
#52002=CARTESIAN_POINT('Ctrl Pts',(0.8359169456045,4.036490248204,-5.561605388383));
#52003=CARTESIAN_POINT('Ctrl Pts',(2.29312655145,3.425431546469,-5.60764705505));
#52004=CARTESIAN_POINT('Ctrl Pts',(3.413377863899,2.311030553742,-5.653688721716));
#52005=CARTESIAN_POINT('Ctrl Pts',(4.03205808599,0.8570404032131,-5.699730388383));
#52006=CARTESIAN_POINT('Ctrl Pts',(4.058256652206,-0.7228856109492,-5.74577205505));
#52007=CARTESIAN_POINT('Ctrl Pts',(3.488123873377,-2.196588833996,-5.791813721716));
#52008=CARTESIAN_POINT('Ctrl Pts',(2.405436621222,-3.347519278951,-5.837855388383));
#52009=CARTESIAN_POINT('Ctrl Pts',(0.9692879252418,-4.006556074691,-5.88389705505));
#52010=CARTESIAN_POINT('Ctrl Pts',(-0.6092905926321,-4.076858549839,-5.929938721716));
#52011=CARTESIAN_POINT('Ctrl Pts',(-2.098338282431,-3.548096266189,-5.975980388383));
#52012=CARTESIAN_POINT('Ctrl Pts',(-3.279050399221,-2.497967001589,-6.02202205505));
#52013=CARTESIAN_POINT('Ctrl Pts',(-3.97792987147,-1.080779625702,-6.068063721716));
#52014=CARTESIAN_POINT('Ctrl Pts',(-4.092281435813,0.4952204678384,-6.114105388383));
#52015=CARTESIAN_POINT('Ctrl Pts',(-3.605301960262,1.998451509793,-6.16014705505));
#52016=CARTESIAN_POINT('Ctrl Pts',(-2.588549542429,3.208024614627,-6.206188721716));
#52017=CARTESIAN_POINT('Ctrl Pts',(-1.19142856672,3.946201798194,-6.252230388383));
#52018=CARTESIAN_POINT('Ctrl Pts',(0.3807641850203,4.104513283822,-6.29827205505));
#52019=CARTESIAN_POINT('Ctrl Pts',(1.897006404783,3.659696348315,-6.344313721716));
#52020=CARTESIAN_POINT('Ctrl Pts',(3.134497308938,2.677113610201,-6.390355388383));
#52021=CARTESIAN_POINT('Ctrl Pts',(3.91139659546,1.30114846758,-6.43639705505));
#52022=CARTESIAN_POINT('Ctrl Pts',(4.113544555839,-0.2660109937444,-6.482438721716));
#52023=CARTESIAN_POINT('Ctrl Pts',(3.711237015243,-1.794082071242,-6.528480388383));
#52024=CARTESIAN_POINT('Ctrl Pts',(2.763590145309,-3.058525816535,-6.57452205505));
#52025=CARTESIAN_POINT('Ctrl Pts',(1.409853772006,-3.873541403319,-6.620563721716));
#52026=CARTESIAN_POINT('Ctrl Pts',(-0.1510503750974,-4.119368209549,-6.666605388383));
#52027=CARTESIAN_POINT('Ctrl Pts',(-1.689758766469,-3.759883771183,-6.71264705505));
#52028=CARTESIAN_POINT('Ctrl Pts',(-2.980169377703,-2.847911715953,-6.758688721716));
#52029=CARTESIAN_POINT('Ctrl Pts',(-3.83266574011,-1.517459714869,-6.804730388383));
#52030=CARTESIAN_POINT('Ctrl Pts',(-4.121979703844,0.03597197191164,-6.85077205505));
#52031=CARTESIAN_POINT('Ctrl Pts',(-3.805598682858,1.584117838639,-6.896813721716));
#52032=CARTESIAN_POINT('Ctrl Pts',(-2.930012570708,2.899489092436,-6.942855388383));
#52033=CARTESIAN_POINT('Ctrl Pts',(-1.623882388293,3.788801479446,-6.98889705505));
#52034=CARTESIAN_POINT('Ctrl Pts',(-0.07913448113579,4.121377002357,-7.034938721716));
#52035=CARTESIAN_POINT('Ctrl Pts',(1.47724166337,3.848346103155,-7.080980388383));
#52036=CARTESIAN_POINT('Ctrl Pts',(2.816547872794,3.009828689797,-7.12702205505));
#52037=CARTESIAN_POINT('Ctrl Pts',(3.741982825359,1.729038807078,-7.173063721716));
#52038=CARTESIAN_POINT('Ctrl Pts',(4.117560575058,0.1941792274952,-7.219105388383));
#52039=CARTESIAN_POINT('Ctrl Pts',(3.888092698922,-1.369213579488,-7.26514705505));
#52040=CARTESIAN_POINT('Ctrl Pts',(3.087297835011,-2.731410393844,-7.311188721716));
#52041=CARTESIAN_POINT('Ctrl Pts',(1.832846973412,-3.692246285626,-7.357230388383));
#52042=CARTESIAN_POINT('Ctrl Pts',(0.3090725587339,-4.110533397882,-7.40327205505));
#52043=CARTESIAN_POINT('Ctrl Pts',(-1.260117824043,-3.924807476958,-7.449313721716));
#52044=CARTESIAN_POINT('Ctrl Pts',(-2.644143043235,-3.162359598245,-7.495355388383));
#52045=CARTESIAN_POINT('Ctrl Pts',(-3.639630643292,-1.935225940801,-7.54139705505));
#52046=CARTESIAN_POINT('Ctrl Pts',(-4.100300950458,-0.4237248845199,-7.587438721716));
#52047=CARTESIAN_POINT('Ctrl Pts',(-3.958461808006,1.150039466741,-7.633480388383));
#52048=CARTESIAN_POINT('Ctrl Pts',(-3.234955449255,2.554813868979,-7.67952205505));
#52049=CARTESIAN_POINT('Ctrl Pts',(-2.036095874727,3.584176928104,-7.725563721716));
#52050=CARTESIAN_POINT('Ctrl Pts',(-0.5380468116679,4.086871205575,-7.771605388383));
#52051=CARTESIAN_POINT('Ctrl Pts',(1.039064377895,3.98902947244,-7.81764705505));
#52052=CARTESIAN_POINT('Ctrl Pts',(2.463492398452,3.305028694111,-7.863688721716));
#52053=CARTESIAN_POINT('Ctrl Pts',(3.525928861993,2.135378440328,-7.909730388383));
#52054=CARTESIAN_POINT('Ctrl Pts',(4.070252841003,0.6519479993433,-7.95577205505));
#52055=CARTESIAN_POINT('Ctrl Pts',(4.016493331088,-0.9272746288775,-8.001813721716));
#52056=CARTESIAN_POINT('Ctrl Pts',(3.372499699855,-2.370266500001,-8.047855388383));
#52057=CARTESIAN_POINT('Ctrl Pts',(2.612892894131,-3.100001962842,-8.078549832827));
#52058=CARTESIAN_POINT('Ctrl Pts',(2.178308200468,-3.380072686139,-8.09389705505));
#52059=CARTESIAN_POINT('Origin',(0.,5.773502691896,-10.5));
#52060=CARTESIAN_POINT('',(4.5,3.175426480543,-11.73961639634));
#52061=CARTESIAN_POINT('Origin',(4.,2.309401076759,-28.10392));
#52062=CARTESIAN_POINT('',(5.,2.309401076759,-11.73961639634));
#52063=CARTESIAN_POINT('Origin',(5.,2.886751345948,-10.5));
#52064=CARTESIAN_POINT('',(5.,-2.309401076759,-11.73961639634));
#52065=CARTESIAN_POINT('Origin',(4.,-2.309401076759,-28.10392));
#52066=CARTESIAN_POINT('',(4.5,-3.175426480543,-11.73961639634));
#52067=CARTESIAN_POINT('Origin',(5.,-2.886751345948,-10.5));
#52068=CARTESIAN_POINT('',(0.5,-5.484827557301,-11.73961639634));
#52069=CARTESIAN_POINT('Origin',(0.,-4.618802153517,-28.10392));
#52070=CARTESIAN_POINT('',(-0.5,-5.484827557301,-11.73961639634));
#52071=CARTESIAN_POINT('Origin',(-5.,2.886751345948,-10.5));
#52072=CARTESIAN_POINT('',(-4.5,3.175426480543,-11.73961639634));
#52073=CARTESIAN_POINT('Origin',(-4.,2.309401076759,-28.10392));
#52074=CARTESIAN_POINT('',(-5.,2.309401076758,-11.73961639634));
#52075=CARTESIAN_POINT('Origin',(-5.,-2.886751345948,-10.5));
#52076=CARTESIAN_POINT('',(-5.,-2.309401076759,-11.73961639634));
#52077=CARTESIAN_POINT('Origin',(-4.,-2.309401076759,-28.10392));
#52078=CARTESIAN_POINT('',(-4.5,-3.175426480543,-11.73961639634));
#52079=CARTESIAN_POINT('Origin',(0.,-5.773502691896,-10.5));
#52145=UNCERTAINTY_MEASURE_WITH_UNIT(LENGTH_MEASURE(0.01),#52165,
'DISTANCE_ACCURACY_VALUE',
'Maximum model space distance between geometric entities at asserted c
onnectivities');
#52149=UNCERTAINTY_MEASURE_WITH_UNIT(LENGTH_MEASURE(0.01),#52165,
'DISTANCE_ACCURACY_VALUE',
'Maximum model space distance between geometric entities at asserted c
onnectivities');
#52160=(
GEOMETRIC_REPRESENTATION_CONTEXT(3)
GLOBAL_UNCERTAINTY_ASSIGNED_CONTEXT((#52145))
GLOBAL_UNIT_ASSIGNED_CONTEXT((#52165,#52167,#52168))
REPRESENTATION_CONTEXT('','3D')
);
#52164=(
GEOMETRIC_REPRESENTATION_CONTEXT(3)
GLOBAL_UNCERTAINTY_ASSIGNED_CONTEXT((#52149))
GLOBAL_UNIT_ASSIGNED_CONTEXT((#52165,#52167,#52168))
REPRESENTATION_CONTEXT('','3D')
);
#52165=(
LENGTH_UNIT()
NAMED_UNIT(*)
SI_UNIT(.MILLI.,.METRE.)
);
#52167=(
NAMED_UNIT(*)
PLANE_ANGLE_UNIT()
SI_UNIT($,.RADIAN.)
);
#52168=(
NAMED_UNIT(*)
SI_UNIT($,.STERADIAN.)
SOLID_ANGLE_UNIT()
);
#52179=SHAPE_DEFINITION_REPRESENTATION(#52193,#52220);
#52193=PRODUCT_DEFINITION_SHAPE('',$,#52235);
#52220=SHAPE_REPRESENTATION('',(#10142),#52160);
#52224=PRODUCT_DEFINITION_CONTEXT('part definition',#52268,'design');
#52235=PRODUCT_DEFINITION('Bushing / Bearing Sleeve',
'Bushing / Bearing Sleeve',#52249,#52224);
#52249=PRODUCT_DEFINITION_FORMATION('',$,#52280);
#52268=APPLICATION_CONTEXT('Managed model based 3d engineering');
#52269=PRODUCT_CONTEXT('part definition',#52268,'mechanical');
#52280=PRODUCT('Bushing / Bearing Sleeve','Bushing / Bearing Sleeve',
'NOT SPECIFIED',(#52269));
#52312=COLOUR_RGB('Grey',0.48,0.52,0.57);
#52313=FILL_AREA_STYLE_COLOUR('',#52312);
#52314=FILL_AREA_STYLE('',(#52313));
#52315=SURFACE_STYLE_FILL_AREA(#52314);
#52316=SURFACE_SIDE_STYLE('',(#52315));
#52317=SURFACE_STYLE_USAGE(.BOTH.,#52316);
#52318=PRESENTATION_STYLE_ASSIGNMENT((#52317));
ENDSEC;
END-ISO-10303-21;
